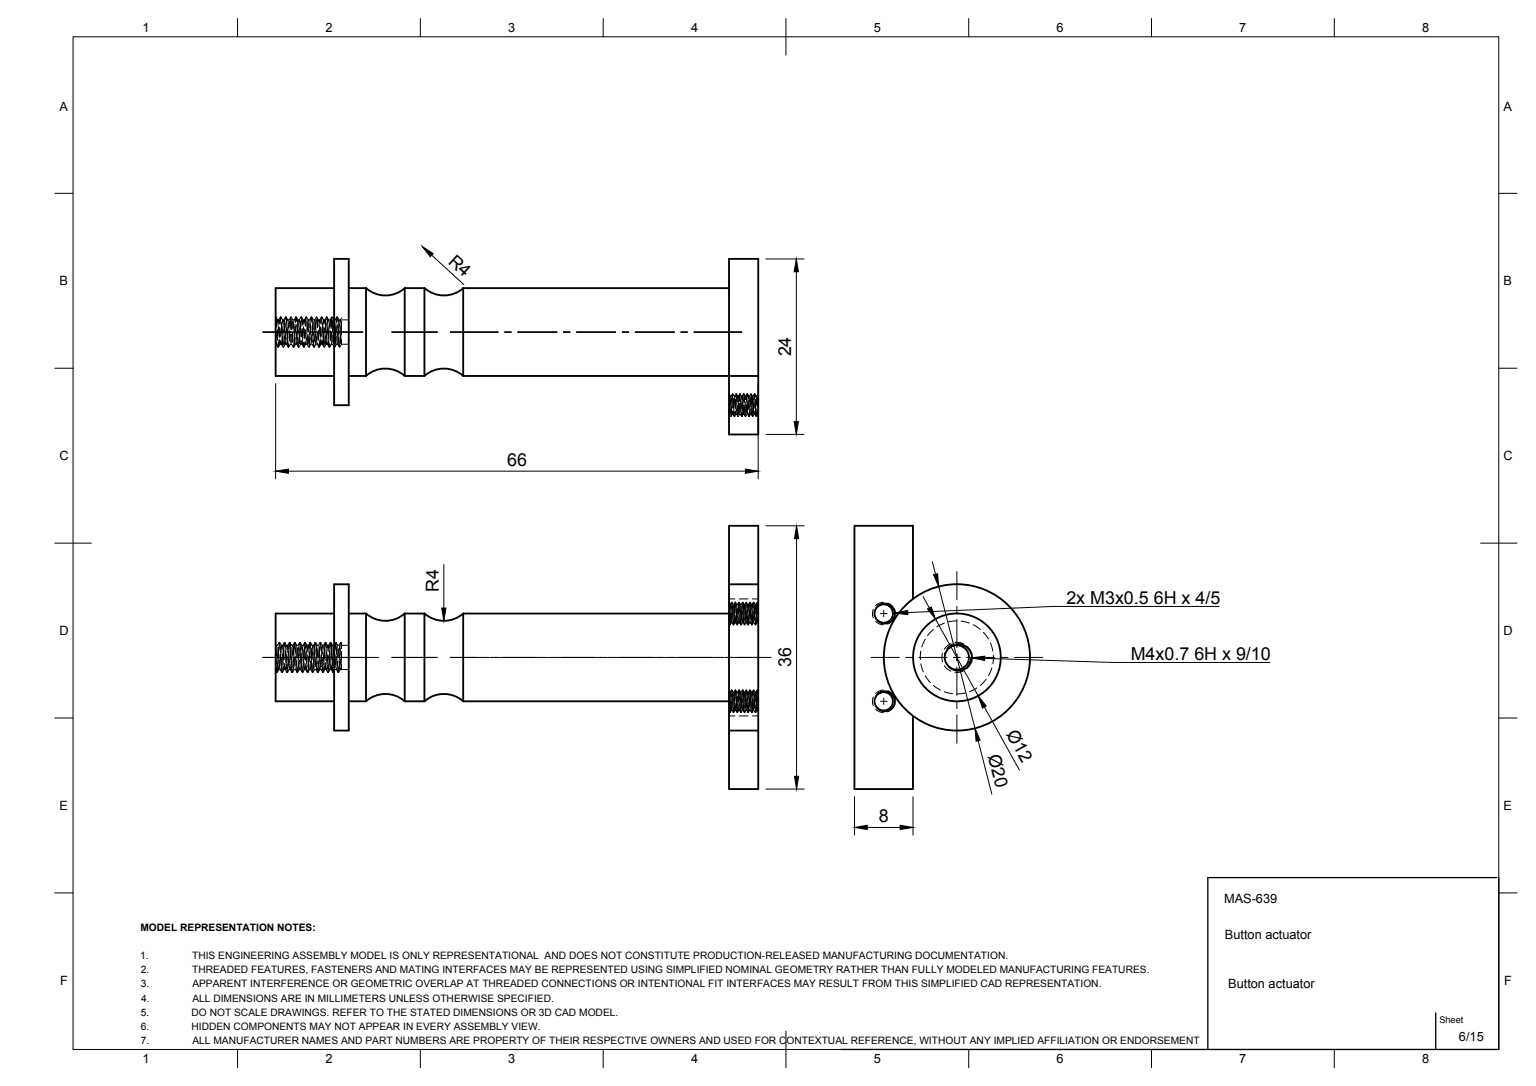
ISO-10303-21;
HEADER;
/* Generated by software containing ST-Developer
 * from STEP Tools, Inc. (www.steptools.com) 
 */

FILE_DESCRIPTION(
/* description */ ('Independent maintained push-to-latch/pull-to-reset mushroom-operator 
CAD. Two opposed spring-loaded ball detents in turned circular seats b
ias both travel stops; direct normally-closed bridge opens6mm when pre
ssed. Rounded palm/pull rim, captured head screw, removable detent clo
sures, native Coil spring families, insulated shared terminals and ord
inary machining features. Manual geometric states and ideal same-mater
ial spring-energy direction only; no electrical/safety certification, 
force/contact dynamics, wear, load or life rating. Requested blue/gray
 visual palette, not safety identification. External wiring/anchors an
d application engineering omitted.'),
/* implementation_level */ '2;1');

FILE_NAME(
/* name */ 'Button actuator.step',
/* time_stamp */ '2026-11-08T17:54:26-08:00',
/* author */ (''),
/* organization */ (''),
/* preprocessor_version */ 'ST-DEVELOPER v20.2',
/* originating_system */ 'Autodesk Translation Framework v15.17.0.0',
/* authorisation */ '');

FILE_SCHEMA (('AUTOMOTIVE_DESIGN { 1 0 10303 214 3 1 1 }'));
ENDSEC;

DATA;
#10=MECHANICAL_DESIGN_GEOMETRIC_PRESENTATION_REPRESENTATION('',(#193),#43980);
#152=TOROIDAL_SURFACE('',#11821,0.899999999999998,0.399999999999998);
#153=TOROIDAL_SURFACE('',#11827,0.900000000000001,0.4);
#159=SHAPE_REPRESENTATION_RELATIONSHIP('SRR','None',#44059,#176);
#176=ADVANCED_BREP_SHAPE_REPRESENTATION('',(#210),#43966);
#193=STYLED_ITEM('',(#44153),#210);
#210=MANIFOLD_SOLID_BREP('Body1',#11234);
#236=B_SPLINE_SURFACE_WITH_KNOTS('',3,3,((#26841,#26842,#26843,#26844,#26845,
#26846,#26847,#26848,#26849,#26850,#26851,#26852,#26853,#26854,#26855,#26856,
#26857,#26858,#26859,#26860,#26861,#26862,#26863,#26864,#26865,#26866,#26867,
#26868,#26869,#26870,#26871,#26872,#26873,#26874,#26875,#26876,#26877,#26878,
#26879,#26880,#26881,#26882,#26883,#26884,#26885,#26886,#26887,#26888,#26889,
#26890,#26891,#26892,#26893,#26894,#26895,#26896),(#26897,#26898,#26899,
#26900,#26901,#26902,#26903,#26904,#26905,#26906,#26907,#26908,#26909,#26910,
#26911,#26912,#26913,#26914,#26915,#26916,#26917,#26918,#26919,#26920,#26921,
#26922,#26923,#26924,#26925,#26926,#26927,#26928,#26929,#26930,#26931,#26932,
#26933,#26934,#26935,#26936,#26937,#26938,#26939,#26940,#26941,#26942,#26943,
#26944,#26945,#26946,#26947,#26948,#26949,#26950,#26951,#26952),(#26953,
#26954,#26955,#26956,#26957,#26958,#26959,#26960,#26961,#26962,#26963,#26964,
#26965,#26966,#26967,#26968,#26969,#26970,#26971,#26972,#26973,#26974,#26975,
#26976,#26977,#26978,#26979,#26980,#26981,#26982,#26983,#26984,#26985,#26986,
#26987,#26988,#26989,#26990,#26991,#26992,#26993,#26994,#26995,#26996,#26997,
#26998,#26999,#27000,#27001,#27002,#27003,#27004,#27005,#27006,#27007,#27008),
(#27009,#27010,#27011,#27012,#27013,#27014,#27015,#27016,#27017,#27018,
#27019,#27020,#27021,#27022,#27023,#27024,#27025,#27026,#27027,#27028,#27029,
#27030,#27031,#27032,#27033,#27034,#27035,#27036,#27037,#27038,#27039,#27040,
#27041,#27042,#27043,#27044,#27045,#27046,#27047,#27048,#27049,#27050,#27051,
#27052,#27053,#27054,#27055,#27056,#27057,#27058,#27059,#27060,#27061,#27062,
#27063,#27064)),.UNSPECIFIED.,.F.,.F.,.F.,(4,4),(4,1,1,1,1,1,1,1,1,1,1,
1,1,1,1,1,1,1,1,1,1,1,1,1,1,1,1,1,1,1,1,1,1,1,1,1,1,1,1,1,1,1,1,1,1,1,1,
1,1,1,1,1,1,4),(0.,0.0321584099938621),(11.8553612635793,12.8418906022433,
13.8284199409074,14.8149492795714,15.8014786182354,16.7880079568995,17.7745372955635,
18.7610666342275,19.7475959728915,20.7341253115556,21.7206546502196,22.7071839888836,
23.6937133275477,24.6802426662117,25.6667720048757,26.6533013435398,27.6398306822038,
28.6263600208678,29.6128893595319,30.5994186981959,31.5859480368599,32.5724773755239,
33.559006714188,34.545536052852,35.532065391516,36.5185947301801,37.5051240688441,
38.4916534075081,39.4781827461722,40.4647120848362,41.4512414235002,42.4377707621643,
43.4243001008283,44.4108294394923,45.3973587781563,46.3838881168204,47.3704174554844,
48.3569467941484,49.3434761328125,50.3300054714765,51.3165348101405,52.3030641488046,
53.2895934874686,54.2761228261326,55.2626521647967,56.2491815034607,57.2357108421247,
58.2222401807888,59.2087695194528,60.1952988581168,61.1818281967808,62.1683575354449,
63.1548868741089,64.1414162127729),.UNSPECIFIED.);
#237=B_SPLINE_SURFACE_WITH_KNOTS('',3,3,((#27191,#27192,#27193,#27194,#27195,
#27196,#27197,#27198,#27199,#27200,#27201,#27202,#27203,#27204,#27205,#27206,
#27207,#27208,#27209,#27210,#27211,#27212,#27213,#27214,#27215,#27216,#27217,
#27218,#27219,#27220,#27221,#27222,#27223,#27224,#27225,#27226,#27227,#27228,
#27229,#27230,#27231,#27232,#27233,#27234,#27235,#27236,#27237,#27238,#27239,
#27240,#27241,#27242,#27243,#27244,#27245,#27246),(#27247,#27248,#27249,
#27250,#27251,#27252,#27253,#27254,#27255,#27256,#27257,#27258,#27259,#27260,
#27261,#27262,#27263,#27264,#27265,#27266,#27267,#27268,#27269,#27270,#27271,
#27272,#27273,#27274,#27275,#27276,#27277,#27278,#27279,#27280,#27281,#27282,
#27283,#27284,#27285,#27286,#27287,#27288,#27289,#27290,#27291,#27292,#27293,
#27294,#27295,#27296,#27297,#27298,#27299,#27300,#27301,#27302),(#27303,
#27304,#27305,#27306,#27307,#27308,#27309,#27310,#27311,#27312,#27313,#27314,
#27315,#27316,#27317,#27318,#27319,#27320,#27321,#27322,#27323,#27324,#27325,
#27326,#27327,#27328,#27329,#27330,#27331,#27332,#27333,#27334,#27335,#27336,
#27337,#27338,#27339,#27340,#27341,#27342,#27343,#27344,#27345,#27346,#27347,
#27348,#27349,#27350,#27351,#27352,#27353,#27354,#27355,#27356,#27357,#27358),
(#27359,#27360,#27361,#27362,#27363,#27364,#27365,#27366,#27367,#27368,
#27369,#27370,#27371,#27372,#27373,#27374,#27375,#27376,#27377,#27378,#27379,
#27380,#27381,#27382,#27383,#27384,#27385,#27386,#27387,#27388,#27389,#27390,
#27391,#27392,#27393,#27394,#27395,#27396,#27397,#27398,#27399,#27400,#27401,
#27402,#27403,#27404,#27405,#27406,#27407,#27408,#27409,#27410,#27411,#27412,
#27413,#27414)),.UNSPECIFIED.,.F.,.F.,.F.,(4,4),(4,1,1,1,1,1,1,1,1,1,1,
1,1,1,1,1,1,1,1,1,1,1,1,1,1,1,1,1,1,1,1,1,1,1,1,1,1,1,1,1,1,1,1,1,1,1,1,
1,1,1,1,1,1,4),(0.,0.0321584099938621),(14.3984001269718,15.3849294656359,
16.3714588042999,17.3579881429639,18.344517481628,19.331046820292,20.317576158956,
21.30410549762,22.2906348362841,23.2771641749481,24.2636935136121,25.2502228522762,
26.2367521909402,27.2232815296042,28.2098108682683,29.1963402069323,30.1828695455963,
31.1693988842604,32.1559282229244,33.1424575615884,34.1289869002524,35.1155162389165,
36.1020455775805,37.0885749162445,38.0751042549086,39.0616335935726,40.0481629322366,
41.0346922709007,42.0212216095647,43.0077509482287,43.9942802868928,44.9808096255568,
45.9673389642208,46.9538683028848,47.9403976415489,48.9269269802129,49.9134563188769,
50.899985657541,51.886514996205,52.873044334869,53.8595736735331,54.8461030121971,
55.8326323508611,56.8191616895251,57.8056910281892,58.7922203668532,59.7787497055172,
60.7652790441813,61.7518083828453,62.7383377215093,63.7248670601734,64.7113963988374,
65.6979257375014,66.6844550761655),.UNSPECIFIED.);
#238=B_SPLINE_SURFACE_WITH_KNOTS('',3,3,((#27677,#27678,#27679,#27680,#27681,
#27682,#27683,#27684,#27685,#27686,#27687,#27688,#27689,#27690,#27691,#27692,
#27693,#27694,#27695,#27696,#27697,#27698,#27699,#27700,#27701,#27702,#27703,
#27704,#27705,#27706,#27707,#27708,#27709,#27710,#27711,#27712,#27713,#27714,
#27715,#27716,#27717,#27718,#27719,#27720,#27721,#27722,#27723,#27724,#27725,
#27726,#27727,#27728,#27729,#27730,#27731,#27732),(#27733,#27734,#27735,
#27736,#27737,#27738,#27739,#27740,#27741,#27742,#27743,#27744,#27745,#27746,
#27747,#27748,#27749,#27750,#27751,#27752,#27753,#27754,#27755,#27756,#27757,
#27758,#27759,#27760,#27761,#27762,#27763,#27764,#27765,#27766,#27767,#27768,
#27769,#27770,#27771,#27772,#27773,#27774,#27775,#27776,#27777,#27778,#27779,
#27780,#27781,#27782,#27783,#27784,#27785,#27786,#27787,#27788),(#27789,
#27790,#27791,#27792,#27793,#27794,#27795,#27796,#27797,#27798,#27799,#27800,
#27801,#27802,#27803,#27804,#27805,#27806,#27807,#27808,#27809,#27810,#27811,
#27812,#27813,#27814,#27815,#27816,#27817,#27818,#27819,#27820,#27821,#27822,
#27823,#27824,#27825,#27826,#27827,#27828,#27829,#27830,#27831,#27832,#27833,
#27834,#27835,#27836,#27837,#27838,#27839,#27840,#27841,#27842,#27843,#27844),
(#27845,#27846,#27847,#27848,#27849,#27850,#27851,#27852,#27853,#27854,
#27855,#27856,#27857,#27858,#27859,#27860,#27861,#27862,#27863,#27864,#27865,
#27866,#27867,#27868,#27869,#27870,#27871,#27872,#27873,#27874,#27875,#27876,
#27877,#27878,#27879,#27880,#27881,#27882,#27883,#27884,#27885,#27886,#27887,
#27888,#27889,#27890,#27891,#27892,#27893,#27894,#27895,#27896,#27897,#27898,
#27899,#27900)),.UNSPECIFIED.,.F.,.F.,.F.,(4,4),(4,1,1,1,1,1,1,1,1,1,1,
1,1,1,1,1,1,1,1,1,1,1,1,1,1,1,1,1,1,1,1,1,1,1,1,1,1,1,1,1,1,1,1,1,1,1,1,
1,1,1,1,1,1,4),(0.,0.0321584099938621),(11.8553612635793,12.8418906022433,
13.8284199409074,14.8149492795714,15.8014786182354,16.7880079568995,17.7745372955635,
18.7610666342275,19.7475959728915,20.7341253115556,21.7206546502196,22.7071839888836,
23.6937133275477,24.6802426662117,25.6667720048757,26.6533013435398,27.6398306822038,
28.6263600208678,29.6128893595319,30.5994186981959,31.5859480368599,32.5724773755239,
33.559006714188,34.545536052852,35.532065391516,36.5185947301801,37.5051240688441,
38.4916534075081,39.4781827461722,40.4647120848362,41.4512414235002,42.4377707621643,
43.4243001008283,44.4108294394923,45.3973587781563,46.3838881168204,47.3704174554844,
48.3569467941484,49.3434761328125,50.3300054714765,51.3165348101405,52.3030641488046,
53.2895934874686,54.2761228261326,55.2626521647967,56.2491815034607,57.2357108421247,
58.2222401807888,59.2087695194528,60.1952988581168,61.1818281967808,62.1683575354449,
63.1548868741089,64.1414162127729),.UNSPECIFIED.);
#239=B_SPLINE_SURFACE_WITH_KNOTS('',3,3,((#27975,#27976,#27977,#27978,#27979,
#27980,#27981,#27982,#27983,#27984,#27985,#27986,#27987,#27988,#27989,#27990,
#27991,#27992,#27993,#27994,#27995,#27996,#27997,#27998,#27999,#28000,#28001,
#28002,#28003,#28004,#28005,#28006,#28007,#28008,#28009,#28010,#28011,#28012,
#28013,#28014,#28015,#28016,#28017,#28018,#28019,#28020,#28021,#28022,#28023,
#28024,#28025,#28026,#28027,#28028,#28029,#28030),(#28031,#28032,#28033,
#28034,#28035,#28036,#28037,#28038,#28039,#28040,#28041,#28042,#28043,#28044,
#28045,#28046,#28047,#28048,#28049,#28050,#28051,#28052,#28053,#28054,#28055,
#28056,#28057,#28058,#28059,#28060,#28061,#28062,#28063,#28064,#28065,#28066,
#28067,#28068,#28069,#28070,#28071,#28072,#28073,#28074,#28075,#28076,#28077,
#28078,#28079,#28080,#28081,#28082,#28083,#28084,#28085,#28086),(#28087,
#28088,#28089,#28090,#28091,#28092,#28093,#28094,#28095,#28096,#28097,#28098,
#28099,#28100,#28101,#28102,#28103,#28104,#28105,#28106,#28107,#28108,#28109,
#28110,#28111,#28112,#28113,#28114,#28115,#28116,#28117,#28118,#28119,#28120,
#28121,#28122,#28123,#28124,#28125,#28126,#28127,#28128,#28129,#28130,#28131,
#28132,#28133,#28134,#28135,#28136,#28137,#28138,#28139,#28140,#28141,#28142),
(#28143,#28144,#28145,#28146,#28147,#28148,#28149,#28150,#28151,#28152,
#28153,#28154,#28155,#28156,#28157,#28158,#28159,#28160,#28161,#28162,#28163,
#28164,#28165,#28166,#28167,#28168,#28169,#28170,#28171,#28172,#28173,#28174,
#28175,#28176,#28177,#28178,#28179,#28180,#28181,#28182,#28183,#28184,#28185,
#28186,#28187,#28188,#28189,#28190,#28191,#28192,#28193,#28194,#28195,#28196,
#28197,#28198)),.UNSPECIFIED.,.F.,.F.,.F.,(4,4),(4,1,1,1,1,1,1,1,1,1,1,
1,1,1,1,1,1,1,1,1,1,1,1,1,1,1,1,1,1,1,1,1,1,1,1,1,1,1,1,1,1,1,1,1,1,1,1,
1,1,1,1,1,1,4),(0.,0.0321584099938621),(14.3984001269718,15.3849294656359,
16.3714588042999,17.3579881429639,18.344517481628,19.331046820292,20.317576158956,
21.30410549762,22.2906348362841,23.2771641749481,24.2636935136121,25.2502228522762,
26.2367521909402,27.2232815296042,28.2098108682683,29.1963402069323,30.1828695455963,
31.1693988842604,32.1559282229244,33.1424575615884,34.1289869002524,35.1155162389165,
36.1020455775805,37.0885749162445,38.0751042549086,39.0616335935726,40.0481629322366,
41.0346922709007,42.0212216095647,43.0077509482287,43.9942802868928,44.9808096255568,
45.9673389642208,46.9538683028848,47.9403976415489,48.9269269802129,49.9134563188769,
50.899985657541,51.886514996205,52.873044334869,53.8595736735331,54.8461030121971,
55.8326323508611,56.8191616895251,57.8056910281892,58.7922203668532,59.7787497055172,
60.7652790441813,61.7518083828453,62.7383377215093,63.7248670601734,64.7113963988374,
65.6979257375014,66.6844550761655),.UNSPECIFIED.);
#240=B_SPLINE_SURFACE_WITH_KNOTS('',3,3,((#28411,#28412,#28413,#28414,#28415,
#28416,#28417,#28418,#28419,#28420,#28421,#28422,#28423,#28424,#28425,#28426,
#28427,#28428,#28429,#28430,#28431,#28432,#28433,#28434,#28435,#28436,#28437,
#28438,#28439,#28440,#28441,#28442,#28443,#28444,#28445,#28446,#28447,#28448,
#28449,#28450,#28451,#28452,#28453,#28454,#28455,#28456,#28457,#28458,#28459,
#28460,#28461,#28462,#28463,#28464,#28465,#28466,#28467,#28468,#28469,#28470,
#28471,#28472,#28473,#28474,#28475,#28476,#28477,#28478,#28479,#28480,#28481,
#28482,#28483,#28484,#28485,#28486,#28487,#28488,#28489,#28490,#28491,#28492,
#28493,#28494,#28495,#28496),(#28497,#28498,#28499,#28500,#28501,#28502,
#28503,#28504,#28505,#28506,#28507,#28508,#28509,#28510,#28511,#28512,#28513,
#28514,#28515,#28516,#28517,#28518,#28519,#28520,#28521,#28522,#28523,#28524,
#28525,#28526,#28527,#28528,#28529,#28530,#28531,#28532,#28533,#28534,#28535,
#28536,#28537,#28538,#28539,#28540,#28541,#28542,#28543,#28544,#28545,#28546,
#28547,#28548,#28549,#28550,#28551,#28552,#28553,#28554,#28555,#28556,#28557,
#28558,#28559,#28560,#28561,#28562,#28563,#28564,#28565,#28566,#28567,#28568,
#28569,#28570,#28571,#28572,#28573,#28574,#28575,#28576,#28577,#28578,#28579,
#28580,#28581,#28582),(#28583,#28584,#28585,#28586,#28587,#28588,#28589,
#28590,#28591,#28592,#28593,#28594,#28595,#28596,#28597,#28598,#28599,#28600,
#28601,#28602,#28603,#28604,#28605,#28606,#28607,#28608,#28609,#28610,#28611,
#28612,#28613,#28614,#28615,#28616,#28617,#28618,#28619,#28620,#28621,#28622,
#28623,#28624,#28625,#28626,#28627,#28628,#28629,#28630,#28631,#28632,#28633,
#28634,#28635,#28636,#28637,#28638,#28639,#28640,#28641,#28642,#28643,#28644,
#28645,#28646,#28647,#28648,#28649,#28650,#28651,#28652,#28653,#28654,#28655,
#28656,#28657,#28658,#28659,#28660,#28661,#28662,#28663,#28664,#28665,#28666,
#28667,#28668),(#28669,#28670,#28671,#28672,#28673,#28674,#28675,#28676,
#28677,#28678,#28679,#28680,#28681,#28682,#28683,#28684,#28685,#28686,#28687,
#28688,#28689,#28690,#28691,#28692,#28693,#28694,#28695,#28696,#28697,#28698,
#28699,#28700,#28701,#28702,#28703,#28704,#28705,#28706,#28707,#28708,#28709,
#28710,#28711,#28712,#28713,#28714,#28715,#28716,#28717,#28718,#28719,#28720,
#28721,#28722,#28723,#28724,#28725,#28726,#28727,#28728,#28729,#28730,#28731,
#28732,#28733,#28734,#28735,#28736,#28737,#28738,#28739,#28740,#28741,#28742,
#28743,#28744,#28745,#28746,#28747,#28748,#28749,#28750,#28751,#28752,#28753,
#28754)),.UNSPECIFIED.,.F.,.F.,.F.,(4,4),(4,1,1,1,1,1,1,1,1,1,1,1,1,1,1,
1,1,1,1,1,1,1,1,1,1,1,1,1,1,1,1,1,1,1,1,1,1,1,1,1,1,1,1,1,1,1,1,1,1,1,1,
1,1,1,1,1,1,1,1,1,1,1,1,1,1,1,1,1,1,1,1,1,1,1,1,1,1,1,1,1,1,1,1,4),(0.,
0.0448889834294937),(11.8615800042566,12.8591513772395,13.8567227502225,
14.8542941232054,15.8518654961883,16.8494368691713,17.8470082421542,18.8445796151371,
19.8421509881201,20.839722361103,21.837293734086,22.8348651070689,23.8324364800518,
24.8300078530348,25.8275792260177,26.8251505990006,27.8227219719836,28.8202933449665,
29.8178647179494,30.8154360909324,31.8130074639153,32.8105788368982,33.8081502098812,
34.8057215828641,35.803292955847,36.80086432883,37.7984357018129,38.7960070747958,
39.7935784477788,40.7911498207617,41.7887211937446,42.7862925667276,43.7838639397105,
44.7814353126934,45.7790066856764,46.7765780586593,47.7741494316422,48.7717208046252,
49.7692921776081,50.766863550591,51.764434923574,52.7620062965569,53.7595776695398,
54.7571490425228,55.7547204155057,56.7522917884886,57.7498631614716,58.7474345344545,
59.7450059074374,60.7425772804204,61.7401486534033,62.7377200263862,63.7352913993692,
64.7328627723521,65.730434145335,66.728005518318,67.7255768913009,68.7231482642838,
69.7207196372668,70.7182910102497,71.7158623832326,72.7134337562156,73.7110051291985,
74.7085765021814,75.7061478751644,76.7037192481473,77.7012906211302,78.6988619941132,
79.6964333670961,80.6940047400791,81.691576113062,82.6891474860449,83.6867188590278,
84.6842902320108,85.6818616049937,86.6794329779766,87.6770043509596,88.6745757239425,
89.6721470969255,90.6697184699084,91.6672898428913,92.6648612158743,93.6624325888572,
94.6600039618401),.UNSPECIFIED.);
#241=B_SPLINE_SURFACE_WITH_KNOTS('',3,3,((#28832,#28833,#28834,#28835,#28836,
#28837,#28838,#28839,#28840,#28841,#28842,#28843,#28844,#28845,#28846,#28847,
#28848,#28849,#28850,#28851,#28852,#28853,#28854,#28855,#28856,#28857,#28858,
#28859,#28860,#28861,#28862,#28863,#28864,#28865,#28866,#28867,#28868,#28869,
#28870,#28871,#28872,#28873,#28874,#28875,#28876,#28877,#28878,#28879,#28880,
#28881,#28882,#28883,#28884,#28885,#28886,#28887,#28888,#28889,#28890,#28891,
#28892,#28893,#28894,#28895,#28896,#28897,#28898,#28899,#28900,#28901,#28902,
#28903,#28904,#28905,#28906,#28907,#28908,#28909,#28910,#28911,#28912,#28913,
#28914,#28915,#28916,#28917),(#28918,#28919,#28920,#28921,#28922,#28923,
#28924,#28925,#28926,#28927,#28928,#28929,#28930,#28931,#28932,#28933,#28934,
#28935,#28936,#28937,#28938,#28939,#28940,#28941,#28942,#28943,#28944,#28945,
#28946,#28947,#28948,#28949,#28950,#28951,#28952,#28953,#28954,#28955,#28956,
#28957,#28958,#28959,#28960,#28961,#28962,#28963,#28964,#28965,#28966,#28967,
#28968,#28969,#28970,#28971,#28972,#28973,#28974,#28975,#28976,#28977,#28978,
#28979,#28980,#28981,#28982,#28983,#28984,#28985,#28986,#28987,#28988,#28989,
#28990,#28991,#28992,#28993,#28994,#28995,#28996,#28997,#28998,#28999,#29000,
#29001,#29002,#29003),(#29004,#29005,#29006,#29007,#29008,#29009,#29010,
#29011,#29012,#29013,#29014,#29015,#29016,#29017,#29018,#29019,#29020,#29021,
#29022,#29023,#29024,#29025,#29026,#29027,#29028,#29029,#29030,#29031,#29032,
#29033,#29034,#29035,#29036,#29037,#29038,#29039,#29040,#29041,#29042,#29043,
#29044,#29045,#29046,#29047,#29048,#29049,#29050,#29051,#29052,#29053,#29054,
#29055,#29056,#29057,#29058,#29059,#29060,#29061,#29062,#29063,#29064,#29065,
#29066,#29067,#29068,#29069,#29070,#29071,#29072,#29073,#29074,#29075,#29076,
#29077,#29078,#29079,#29080,#29081,#29082,#29083,#29084,#29085,#29086,#29087,
#29088,#29089),(#29090,#29091,#29092,#29093,#29094,#29095,#29096,#29097,
#29098,#29099,#29100,#29101,#29102,#29103,#29104,#29105,#29106,#29107,#29108,
#29109,#29110,#29111,#29112,#29113,#29114,#29115,#29116,#29117,#29118,#29119,
#29120,#29121,#29122,#29123,#29124,#29125,#29126,#29127,#29128,#29129,#29130,
#29131,#29132,#29133,#29134,#29135,#29136,#29137,#29138,#29139,#29140,#29141,
#29142,#29143,#29144,#29145,#29146,#29147,#29148,#29149,#29150,#29151,#29152,
#29153,#29154,#29155,#29156,#29157,#29158,#29159,#29160,#29161,#29162,#29163,
#29164,#29165,#29166,#29167,#29168,#29169,#29170,#29171,#29172,#29173,#29174,
#29175)),.UNSPECIFIED.,.F.,.F.,.F.,(4,4),(4,1,1,1,1,1,1,1,1,1,1,1,1,1,1,
1,1,1,1,1,1,1,1,1,1,1,1,1,1,1,1,1,1,1,1,1,1,1,1,1,1,1,1,1,1,1,1,1,1,1,1,
1,1,1,1,1,1,1,1,1,1,1,1,1,1,1,1,1,1,1,1,1,1,1,1,1,1,1,1,1,1,1,1,4),(0.,
0.0448889834294937),(14.3981410127768,15.3957123857598,16.3932837587427,
17.3908551317256,18.3884265047086,19.3859978776915,20.3835692506744,21.3811406236574,
22.3787119966403,23.3762833696232,24.3738547426062,25.3714261155891,26.368997488572,
27.366568861555,28.3641402345379,29.3617116075208,30.3592829805038,31.3568543534867,
32.3544257264696,33.3519970994526,34.3495684724355,35.3471398454184,36.3447112184014,
37.3422825913843,38.3398539643672,39.3374253373502,40.3349967103331,41.332568083316,
42.330139456299,43.3277108292819,44.3252822022648,45.3228535752478,46.3204249482307,
47.3179963212136,48.3155676941966,49.3131390671795,50.3107104401624,51.3082818131454,
52.3058531861283,53.3034245591112,54.3009959320942,55.2985673050771,56.29613867806,
57.293710051043,58.2912814240259,59.2888527970089,60.2864241699918,61.2839955429747,
62.2815669159576,63.2791382889406,64.2767096619235,65.2742810349065,66.2718524078894,
67.2694237808723,68.2669951538552,69.2645665268382,70.2621378998211,71.2597092728041,
72.257280645787,73.2548520187699,74.2524233917528,75.2499947647358,76.2475661377187,
77.2451375107017,78.2427088836846,79.2402802566675,80.2378516296505,81.2354230026334,
82.2329943756163,83.2305657485992,84.2281371215822,85.2257084945651,86.2232798675481,
87.220851240531,88.2184226135139,89.2159939864968,90.2135653594798,91.2111367324627,
92.2087081054457,93.2062794784286,94.2038508514115,95.2014222243945,96.1989935973774,
97.1965649703603),.UNSPECIFIED.);
#298=FACE_BOUND('',#1431,.T.);
#299=FACE_BOUND('',#1432,.T.);
#300=FACE_BOUND('',#1449,.T.);
#301=FACE_BOUND('',#1451,.T.);
#302=FACE_BOUND('',#1462,.T.);
#303=FACE_BOUND('',#1464,.T.);
#304=FACE_BOUND('',#1465,.T.);
#305=FACE_BOUND('',#1466,.T.);
#388=PLANE('',#11812);
#389=PLANE('',#11817);
#390=PLANE('',#11820);
#391=PLANE('',#11832);
#392=PLANE('',#11835);
#393=PLANE('',#11840);
#394=PLANE('',#11841);
#395=PLANE('',#11842);
#396=PLANE('',#11843);
#397=PLANE('',#11844);
#398=PLANE('',#11849);
#399=PLANE('',#11850);
#708=FACE_OUTER_BOUND('',#1370,.T.);
#709=FACE_OUTER_BOUND('',#1371,.T.);
#710=FACE_OUTER_BOUND('',#1372,.T.);
#711=FACE_OUTER_BOUND('',#1373,.T.);
#712=FACE_OUTER_BOUND('',#1374,.T.);
#713=FACE_OUTER_BOUND('',#1375,.T.);
#714=FACE_OUTER_BOUND('',#1376,.T.);
#715=FACE_OUTER_BOUND('',#1377,.T.);
#716=FACE_OUTER_BOUND('',#1378,.T.);
#717=FACE_OUTER_BOUND('',#1379,.T.);
#718=FACE_OUTER_BOUND('',#1380,.T.);
#719=FACE_OUTER_BOUND('',#1381,.T.);
#720=FACE_OUTER_BOUND('',#1382,.T.);
#721=FACE_OUTER_BOUND('',#1383,.T.);
#722=FACE_OUTER_BOUND('',#1384,.T.);
#723=FACE_OUTER_BOUND('',#1385,.T.);
#724=FACE_OUTER_BOUND('',#1386,.T.);
#725=FACE_OUTER_BOUND('',#1387,.T.);
#726=FACE_OUTER_BOUND('',#1388,.T.);
#727=FACE_OUTER_BOUND('',#1389,.T.);
#728=FACE_OUTER_BOUND('',#1390,.T.);
#729=FACE_OUTER_BOUND('',#1391,.T.);
#730=FACE_OUTER_BOUND('',#1392,.T.);
#731=FACE_OUTER_BOUND('',#1393,.T.);
#732=FACE_OUTER_BOUND('',#1394,.T.);
#733=FACE_OUTER_BOUND('',#1395,.T.);
#734=FACE_OUTER_BOUND('',#1396,.T.);
#735=FACE_OUTER_BOUND('',#1397,.T.);
#736=FACE_OUTER_BOUND('',#1398,.T.);
#737=FACE_OUTER_BOUND('',#1399,.T.);
#738=FACE_OUTER_BOUND('',#1400,.T.);
#739=FACE_OUTER_BOUND('',#1401,.T.);
#740=FACE_OUTER_BOUND('',#1402,.T.);
#741=FACE_OUTER_BOUND('',#1403,.T.);
#742=FACE_OUTER_BOUND('',#1404,.T.);
#743=FACE_OUTER_BOUND('',#1405,.T.);
#744=FACE_OUTER_BOUND('',#1406,.T.);
#745=FACE_OUTER_BOUND('',#1407,.T.);
#746=FACE_OUTER_BOUND('',#1408,.T.);
#747=FACE_OUTER_BOUND('',#1409,.T.);
#748=FACE_OUTER_BOUND('',#1410,.T.);
#749=FACE_OUTER_BOUND('',#1411,.T.);
#750=FACE_OUTER_BOUND('',#1412,.T.);
#751=FACE_OUTER_BOUND('',#1413,.T.);
#752=FACE_OUTER_BOUND('',#1414,.T.);
#753=FACE_OUTER_BOUND('',#1415,.T.);
#754=FACE_OUTER_BOUND('',#1416,.T.);
#755=FACE_OUTER_BOUND('',#1417,.T.);
#756=FACE_OUTER_BOUND('',#1418,.T.);
#757=FACE_OUTER_BOUND('',#1419,.T.);
#758=FACE_OUTER_BOUND('',#1420,.T.);
#759=FACE_OUTER_BOUND('',#1421,.T.);
#760=FACE_OUTER_BOUND('',#1422,.T.);
#761=FACE_OUTER_BOUND('',#1423,.T.);
#762=FACE_OUTER_BOUND('',#1424,.T.);
#763=FACE_OUTER_BOUND('',#1425,.T.);
#764=FACE_OUTER_BOUND('',#1426,.T.);
#765=FACE_OUTER_BOUND('',#1427,.T.);
#766=FACE_OUTER_BOUND('',#1428,.T.);
#767=FACE_OUTER_BOUND('',#1429,.T.);
#768=FACE_OUTER_BOUND('',#1430,.T.);
#769=FACE_OUTER_BOUND('',#1433,.T.);
#770=FACE_OUTER_BOUND('',#1434,.T.);
#771=FACE_OUTER_BOUND('',#1435,.T.);
#772=FACE_OUTER_BOUND('',#1436,.T.);
#773=FACE_OUTER_BOUND('',#1437,.T.);
#774=FACE_OUTER_BOUND('',#1438,.T.);
#775=FACE_OUTER_BOUND('',#1439,.T.);
#776=FACE_OUTER_BOUND('',#1440,.T.);
#777=FACE_OUTER_BOUND('',#1441,.T.);
#778=FACE_OUTER_BOUND('',#1442,.T.);
#779=FACE_OUTER_BOUND('',#1443,.T.);
#780=FACE_OUTER_BOUND('',#1444,.T.);
#781=FACE_OUTER_BOUND('',#1445,.T.);
#782=FACE_OUTER_BOUND('',#1446,.T.);
#783=FACE_OUTER_BOUND('',#1447,.T.);
#784=FACE_OUTER_BOUND('',#1448,.T.);
#785=FACE_OUTER_BOUND('',#1450,.T.);
#786=FACE_OUTER_BOUND('',#1452,.T.);
#787=FACE_OUTER_BOUND('',#1453,.T.);
#788=FACE_OUTER_BOUND('',#1454,.T.);
#789=FACE_OUTER_BOUND('',#1455,.T.);
#790=FACE_OUTER_BOUND('',#1456,.T.);
#791=FACE_OUTER_BOUND('',#1457,.T.);
#792=FACE_OUTER_BOUND('',#1458,.T.);
#793=FACE_OUTER_BOUND('',#1459,.T.);
#794=FACE_OUTER_BOUND('',#1460,.T.);
#795=FACE_OUTER_BOUND('',#1461,.T.);
#796=FACE_OUTER_BOUND('',#1463,.T.);
#1370=EDGE_LOOP('',(#8081,#8082,#8083,#8084,#8085,#8086,#8087,#8088));
#1371=EDGE_LOOP('',(#8089,#8090,#8091,#8092));
#1372=EDGE_LOOP('',(#8093,#8094,#8095,#8096));
#1373=EDGE_LOOP('',(#8097,#8098,#8099,#8100));
#1374=EDGE_LOOP('',(#8101,#8102,#8103,#8104));
#1375=EDGE_LOOP('',(#8105,#8106,#8107,#8108));
#1376=EDGE_LOOP('',(#8109,#8110,#8111,#8112));
#1377=EDGE_LOOP('',(#8113,#8114,#8115,#8116));
#1378=EDGE_LOOP('',(#8117,#8118,#8119,#8120));
#1379=EDGE_LOOP('',(#8121,#8122,#8123,#8124));
#1380=EDGE_LOOP('',(#8125,#8126,#8127,#8128));
#1381=EDGE_LOOP('',(#8129,#8130,#8131,#8132));
#1382=EDGE_LOOP('',(#8133,#8134,#8135,#8136));
#1383=EDGE_LOOP('',(#8137,#8138,#8139,#8140));
#1384=EDGE_LOOP('',(#8141,#8142,#8143,#8144));
#1385=EDGE_LOOP('',(#8145,#8146,#8147,#8148));
#1386=EDGE_LOOP('',(#8149,#8150,#8151,#8152));
#1387=EDGE_LOOP('',(#8153,#8154,#8155,#8156));
#1388=EDGE_LOOP('',(#8157,#8158,#8159,#8160));
#1389=EDGE_LOOP('',(#8161,#8162,#8163,#8164));
#1390=EDGE_LOOP('',(#8165,#8166,#8167,#8168));
#1391=EDGE_LOOP('',(#8169,#8170,#8171,#8172));
#1392=EDGE_LOOP('',(#8173,#8174,#8175,#8176));
#1393=EDGE_LOOP('',(#8177,#8178,#8179,#8180));
#1394=EDGE_LOOP('',(#8181,#8182,#8183,#8184));
#1395=EDGE_LOOP('',(#8185,#8186,#8187,#8188));
#1396=EDGE_LOOP('',(#8189,#8190,#8191,#8192));
#1397=EDGE_LOOP('',(#8193,#8194,#8195,#8196));
#1398=EDGE_LOOP('',(#8197,#8198,#8199,#8200));
#1399=EDGE_LOOP('',(#8201,#8202,#8203,#8204));
#1400=EDGE_LOOP('',(#8205,#8206,#8207,#8208));
#1401=EDGE_LOOP('',(#8209,#8210,#8211,#8212));
#1402=EDGE_LOOP('',(#8213,#8214,#8215,#8216));
#1403=EDGE_LOOP('',(#8217,#8218,#8219,#8220));
#1404=EDGE_LOOP('',(#8221,#8222,#8223,#8224));
#1405=EDGE_LOOP('',(#8225,#8226,#8227,#8228));
#1406=EDGE_LOOP('',(#8229,#8230,#8231,#8232));
#1407=EDGE_LOOP('',(#8233,#8234,#8235,#8236));
#1408=EDGE_LOOP('',(#8237,#8238,#8239,#8240));
#1409=EDGE_LOOP('',(#8241,#8242,#8243,#8244));
#1410=EDGE_LOOP('',(#8245,#8246,#8247,#8248));
#1411=EDGE_LOOP('',(#8249,#8250,#8251,#8252));
#1412=EDGE_LOOP('',(#8253,#8254,#8255,#8256));
#1413=EDGE_LOOP('',(#8257,#8258,#8259,#8260));
#1414=EDGE_LOOP('',(#8261,#8262,#8263,#8264));
#1415=EDGE_LOOP('',(#8265,#8266,#8267,#8268));
#1416=EDGE_LOOP('',(#8269,#8270,#8271,#8272));
#1417=EDGE_LOOP('',(#8273,#8274,#8275,#8276));
#1418=EDGE_LOOP('',(#8277,#8278,#8279,#8280));
#1419=EDGE_LOOP('',(#8281,#8282,#8283,#8284));
#1420=EDGE_LOOP('',(#8285,#8286,#8287,#8288));
#1421=EDGE_LOOP('',(#8289,#8290,#8291,#8292));
#1422=EDGE_LOOP('',(#8293,#8294,#8295,#8296));
#1423=EDGE_LOOP('',(#8297,#8298,#8299,#8300));
#1424=EDGE_LOOP('',(#8301,#8302,#8303,#8304));
#1425=EDGE_LOOP('',(#8305,#8306,#8307,#8308));
#1426=EDGE_LOOP('',(#8309,#8310,#8311,#8312));
#1427=EDGE_LOOP('',(#8313,#8314,#8315,#8316));
#1428=EDGE_LOOP('',(#8317,#8318,#8319,#8320,#8321,#8322,#8323,#8324,#8325,
#8326,#8327,#8328,#8329,#8330,#8331,#8332,#8333,#8334,#8335,#8336));
#1429=EDGE_LOOP('',(#8337,#8338,#8339,#8340,#8341,#8342,#8343,#8344,#8345,
#8346,#8347,#8348,#8349,#8350,#8351,#8352,#8353,#8354,#8355,#8356));
#1430=EDGE_LOOP('',(#8357,#8358,#8359,#8360,#8361,#8362));
#1431=EDGE_LOOP('',(#8363,#8364,#8365,#8366));
#1432=EDGE_LOOP('',(#8367,#8368,#8369,#8370));
#1433=EDGE_LOOP('',(#8371,#8372,#8373,#8374));
#1434=EDGE_LOOP('',(#8375,#8376,#8377,#8378,#8379,#8380,#8381,#8382,#8383,
#8384,#8385,#8386,#8387,#8388,#8389,#8390,#8391,#8392,#8393,#8394));
#1435=EDGE_LOOP('',(#8395,#8396,#8397,#8398,#8399,#8400,#8401,#8402,#8403,
#8404,#8405,#8406,#8407,#8408,#8409,#8410,#8411,#8412,#8413,#8414));
#1436=EDGE_LOOP('',(#8415,#8416,#8417,#8418));
#1437=EDGE_LOOP('',(#8419,#8420,#8421,#8422));
#1438=EDGE_LOOP('',(#8423,#8424,#8425,#8426));
#1439=EDGE_LOOP('',(#8427,#8428,#8429,#8430));
#1440=EDGE_LOOP('',(#8431,#8432,#8433,#8434,#8435,#8436,#8437,#8438,#8439,
#8440,#8441,#8442,#8443,#8444,#8445,#8446,#8447,#8448,#8449,#8450,#8451,
#8452,#8453,#8454,#8455,#8456,#8457,#8458,#8459,#8460));
#1441=EDGE_LOOP('',(#8461,#8462,#8463,#8464,#8465,#8466,#8467,#8468,#8469,
#8470,#8471,#8472,#8473,#8474,#8475,#8476,#8477,#8478,#8479,#8480,#8481,
#8482,#8483,#8484,#8485,#8486,#8487,#8488,#8489));
#1442=EDGE_LOOP('',(#8490,#8491,#8492,#8493));
#1443=EDGE_LOOP('',(#8494));
#1444=EDGE_LOOP('',(#8495,#8496,#8497,#8498));
#1445=EDGE_LOOP('',(#8499,#8500,#8501,#8502));
#1446=EDGE_LOOP('',(#8503,#8504,#8505,#8506));
#1447=EDGE_LOOP('',(#8507,#8508,#8509,#8510));
#1448=EDGE_LOOP('',(#8511));
#1449=EDGE_LOOP('',(#8512));
#1450=EDGE_LOOP('',(#8513));
#1451=EDGE_LOOP('',(#8514));
#1452=EDGE_LOOP('',(#8515,#8516,#8517,#8518));
#1453=EDGE_LOOP('',(#8519,#8520,#8521,#8522));
#1454=EDGE_LOOP('',(#8523,#8524,#8525,#8526));
#1455=EDGE_LOOP('',(#8527,#8528,#8529,#8530));
#1456=EDGE_LOOP('',(#8531,#8532,#8533,#8534));
#1457=EDGE_LOOP('',(#8535,#8536,#8537,#8538));
#1458=EDGE_LOOP('',(#8539,#8540,#8541,#8542));
#1459=EDGE_LOOP('',(#8543,#8544,#8545,#8546));
#1460=EDGE_LOOP('',(#8547,#8548,#8549,#8550));
#1461=EDGE_LOOP('',(#8551));
#1462=EDGE_LOOP('',(#8552,#8553,#8554,#8555));
#1463=EDGE_LOOP('',(#8556,#8557,#8558,#8559,#8560,#8561));
#1464=EDGE_LOOP('',(#8562,#8563,#8564,#8565));
#1465=EDGE_LOOP('',(#8566,#8567,#8568,#8569));
#1466=EDGE_LOOP('',(#8570));
#1889=CIRCLE('',#11742,0.1666);
#1890=CIRCLE('',#11743,0.1666);
#1891=CIRCLE('',#11755,0.1666);
#1892=CIRCLE('',#11757,0.205475);
#1893=CIRCLE('',#11770,0.205475);
#1894=CIRCLE('',#11772,0.12645);
#1895=CIRCLE('',#11780,0.12645);
#1896=CIRCLE('',#11782,0.12645);
#1897=CIRCLE('',#11790,0.12645);
#1898=CIRCLE('',#11792,0.1543);
#1899=CIRCLE('',#11800,0.1543);
#1900=CIRCLE('',#11802,0.1543);
#1901=CIRCLE('',#11810,0.1543);
#1902=CIRCLE('',#11813,1.);
#1903=CIRCLE('',#11822,0.6);
#1904=CIRCLE('',#11823,0.399999999999998);
#1905=CIRCLE('',#11824,0.6);
#1906=CIRCLE('',#11826,0.6);
#1907=CIRCLE('',#11828,0.4);
#1908=CIRCLE('',#11829,0.6);
#1909=CIRCLE('',#11831,0.6);
#1910=CIRCLE('',#11833,1.);
#1911=CIRCLE('',#11834,0.6);
#1912=CIRCLE('',#11836,1.);
#1913=CIRCLE('',#11837,0.6);
#1914=CIRCLE('',#11846,1.);
#1915=CIRCLE('',#11848,0.6);
#2282=B_SPLINE_CURVE_WITH_KNOTS('',3,(#24821,#24822,#24823,#24824,#24825,
#24826,#24827,#24828,#24829,#24830,#24831,#24832,#24833,#24834,#24835,#24836,
#24837,#24838,#24839,#24840,#24841,#24842),.UNSPECIFIED.,.F.,.F.,(4,3,3,
3,3,3,3,4),(76.7080459413271,76.8129957196859,77.8105670926688,78.8081384656518,
79.8057098386347,80.8032812116176,81.8008525846005,82.7984239575835),
 .UNSPECIFIED.);
#2283=B_SPLINE_CURVE_WITH_KNOTS('',3,(#24846,#24847,#24848,#24849,#24850,
#24851,#24852),.UNSPECIFIED.,.F.,.F.,(4,3,4),(-80.783811092309,-79.8057098386347,
-79.2446069498474),.UNSPECIFIED.);
#2284=B_SPLINE_CURVE_WITH_KNOTS('',3,(#24856,#24857,#24858,#24859,#24860,
#24861,#24862,#24863,#24864,#24865,#24866,#24867,#24868,#24869,#24870,#24871,
#24872,#24873,#24874,#24875,#24876,#24877),.UNSPECIFIED.,.F.,.F.,(4,3,3,
3,3,3,3,4),(-79.2446069498474,-78.8081384656518,-77.8105670926689,-76.8129957196859,
-75.815424346703,-74.81785297372,-73.8202816007371,-72.9614216426678),
 .UNSPECIFIED.);
#2285=B_SPLINE_CURVE_WITH_KNOTS('',3,(#24882,#24883,#24884,#24885,#24886,
#24887,#24888,#24889,#24890,#24891,#24892,#24893,#24894,#24895,#24896,#24897,
#24898,#24899,#24900,#24901,#24902,#24903),.UNSPECIFIED.,.F.,.F.,(4,3,3,
3,3,3,3,4),(70.4248606341475,70.8275674817883,71.8251388547712,72.8227102277541,
73.8202816007371,74.81785297372,75.815424346703,76.7080459413271),
 .UNSPECIFIED.);
#2286=B_SPLINE_CURVE_WITH_KNOTS('',3,(#24904,#24905,#24906,#24907,#24908,
#24909,#24910,#24911,#24912,#24913,#24914,#24915,#24916,#24917,#24918,#24919,
#24920,#24921,#24922,#24923,#24924,#24925,#24926,#24927,#24928),
 .UNSPECIFIED.,.F.,.F.,(4,3,3,3,3,3,3,3,4),(-72.9614216426678,-72.8227102277542,
-71.8251388547712,-70.8275674817883,-69.8299961088054,-68.8324247358224,
-67.8348533628395,-66.8372819898566,-66.6782363354882),.UNSPECIFIED.);
#2287=B_SPLINE_CURVE_WITH_KNOTS('',3,(#24933,#24934,#24935,#24936,#24937,
#24938,#24939,#24940,#24941,#24942,#24943,#24944,#24945,#24946,#24947,#24948,
#24949,#24950,#24951,#24952,#24953,#24954),.UNSPECIFIED.,.F.,.F.,(4,3,3,
3,3,3,3,4),(64.1416753269679,64.8421392438907,65.8397106168736,66.8372819898565,
67.8348533628395,68.8324247358224,69.8299961088054,70.4248606341475),
 .UNSPECIFIED.);
#2288=B_SPLINE_CURVE_WITH_KNOTS('',3,(#24955,#24956,#24957,#24958,#24959,
#24960,#24961,#24962,#24963,#24964,#24965,#24966,#24967,#24968,#24969,#24970,
#24971,#24972,#24973,#24974,#24975,#24976),.UNSPECIFIED.,.F.,.F.,(4,3,3,
3,3,3,3,4),(-66.6782363354882,-65.8397106168736,-64.8421392438907,-63.8445678709078,
-62.8469964979248,-61.8494251249419,-60.851853751959,-60.3950510283086),
 .UNSPECIFIED.);
#2289=B_SPLINE_CURVE_WITH_KNOTS('',3,(#24981,#24982,#24983,#24984,#24985,
#24986,#24987,#24988,#24989,#24990,#24991,#24992,#24993,#24994,#24995,#24996,
#24997,#24998,#24999,#25000,#25001,#25002),.UNSPECIFIED.,.F.,.F.,(4,3,3,
3,3,3,3,4),(57.8584900197883,58.8567110059931,59.854282378976,60.851853751959,
61.8494251249419,62.8469964979248,63.8445678709078,64.1416753269679),
 .UNSPECIFIED.);
#2290=B_SPLINE_CURVE_WITH_KNOTS('',3,(#25003,#25004,#25005,#25006,#25007,
#25008,#25009,#25010,#25011,#25012,#25013,#25014,#25015,#25016,#25017,#25018,
#25019,#25020,#25021,#25022,#25023,#25024),.UNSPECIFIED.,.F.,.F.,(4,3,3,
3,3,3,3,4),(-60.3950510283086,-59.8542823789761,-58.8567110059931,-57.8591396330102,
-56.8615682600272,-55.8639968870443,-54.8664255140614,-54.111865721129),
 .UNSPECIFIED.);
#2291=B_SPLINE_CURVE_WITH_KNOTS('',3,(#25029,#25030,#25031,#25032,#25033,
#25034,#25035,#25036,#25037,#25038,#25039,#25040,#25041,#25042,#25043,#25044,
#25045,#25046,#25047,#25048,#25049,#25050),.UNSPECIFIED.,.F.,.F.,(4,3,3,
3,3,3,3,4),(51.5753047126088,51.8737113951125,52.8712827680955,53.8688541410784,
54.8664255140613,55.8639968870443,56.8615682600272,57.8584900197883),
 .UNSPECIFIED.);
#2292=B_SPLINE_CURVE_WITH_KNOTS('',3,(#25051,#25052,#25053,#25054,#25055,
#25056,#25057,#25058,#25059,#25060,#25061,#25062,#25063,#25064,#25065,#25066,
#25067,#25068,#25069,#25070,#25071,#25072,#25073,#25074,#25075),
 .UNSPECIFIED.,.F.,.F.,(4,3,3,3,3,3,3,3,4),(-54.111865721129,-53.8688541410784,
-52.8712827680955,-51.8737113951126,-50.8761400221296,-49.8785686491467,
-48.8809972761638,-47.8834259031808,-47.8286804139494),.UNSPECIFIED.);
#2293=B_SPLINE_CURVE_WITH_KNOTS('',3,(#25080,#25081,#25082,#25083,#25084,
#25085,#25086,#25087,#25088,#25089,#25090,#25091,#25092,#25093,#25094,#25095,
#25096,#25097,#25098,#25099,#25100,#25101),.UNSPECIFIED.,.F.,.F.,(4,3,3,
3,3,3,3,4),(45.2921194054292,45.8882831572149,46.8858545301979,47.8834259031808,
48.8809972761637,49.8785686491467,50.8761400221296,51.5753047126088),
 .UNSPECIFIED.);
#2294=B_SPLINE_CURVE_WITH_KNOTS('',3,(#25102,#25103,#25104,#25105,#25106,
#25107,#25108,#25109,#25110,#25111,#25112,#25113,#25114,#25115,#25116,#25117,
#25118,#25119,#25120,#25121,#25122,#25123),.UNSPECIFIED.,.F.,.F.,(4,3,3,
3,3,3,3,4),(-47.8286804139494,-46.8858545301979,-45.888283157215,-44.890711784232,
-43.8931404112491,-42.8955690382662,-41.8979976652832,-41.5454951067698),
 .UNSPECIFIED.);
#2295=B_SPLINE_CURVE_WITH_KNOTS('',3,(#25128,#25129,#25130,#25131,#25132,
#25133,#25134,#25135,#25136,#25137,#25138,#25139,#25140,#25141,#25142,#25143,
#25144,#25145,#25146,#25147,#25148,#25149),.UNSPECIFIED.,.F.,.F.,(4,3,3,
3,3,3,3,4),(39.0089340982495,39.9028549193173,40.9004262923003,41.8979976652832,
42.8955690382661,43.8931404112491,44.890711784232,45.2921194054292),
 .UNSPECIFIED.);
#2296=B_SPLINE_CURVE_WITH_KNOTS('',3,(#25150,#25151,#25152,#25153,#25154,
#25155,#25156,#25157,#25158,#25159,#25160,#25161,#25162,#25163,#25164,#25165,
#25166,#25167,#25168,#25169,#25170,#25171),.UNSPECIFIED.,.F.,.F.,(4,3,3,
3,3,3,3,4),(-41.5454951067698,-40.9004262923003,-39.9028549193174,-38.9052835463344,
-37.9077121733515,-36.9101408003686,-35.9125694273856,-35.2623097995902),
 .UNSPECIFIED.);
#2297=B_SPLINE_CURVE_WITH_KNOTS('',3,(#25176,#25177,#25178,#25179,#25180,
#25181,#25182,#25183,#25184,#25185,#25186,#25187,#25188,#25189,#25190,#25191,
#25192,#25193,#25194,#25195,#25196,#25197,#25198,#25199,#25200),
 .UNSPECIFIED.,.F.,.F.,(4,3,3,3,3,3,3,3,4),(32.7257487910699,32.9198553084368,
33.9174266814197,34.9149980544027,35.9125694273856,36.9101408003685,37.9077121733515,
38.9052835463344,39.0089340982495),.UNSPECIFIED.);
#2298=B_SPLINE_CURVE_WITH_KNOTS('',3,(#25201,#25202,#25203,#25204,#25205,
#25206,#25207,#25208,#25209,#25210,#25211,#25212,#25213,#25214,#25215,#25216,
#25217,#25218,#25219,#25220,#25221,#25222),.UNSPECIFIED.,.F.,.F.,(4,3,3,
3,3,3,3,4),(-35.2623097995902,-34.9149980544027,-33.9174266814197,-32.9198553084368,
-31.9222839354539,-30.924712562471,-29.927141189488,-28.9791244924107),
 .UNSPECIFIED.);
#2299=B_SPLINE_CURVE_WITH_KNOTS('',3,(#25227,#25228,#25229,#25230,#25231,
#25232,#25233,#25234,#25235,#25236,#25237,#25238,#25239,#25240,#25241,#25242,
#25243,#25244,#25245,#25246,#25247,#25248),.UNSPECIFIED.,.F.,.F.,(4,3,3,
3,3,3,3,4),(26.4425634838903,26.9344270705392,27.9319984435221,28.9295698165051,
29.927141189488,30.9247125624709,31.9222839354539,32.7257487910699),
 .UNSPECIFIED.);
#2300=B_SPLINE_CURVE_WITH_KNOTS('',3,(#25249,#25250,#25251,#25252,#25253,
#25254,#25255,#25256,#25257,#25258,#25259,#25260,#25261,#25262,#25263,#25264,
#25265,#25266,#25267,#25268,#25269,#25270,#25271,#25272,#25273),
 .UNSPECIFIED.,.F.,.F.,(4,3,3,3,3,3,3,3,4),(-28.9791244924107,-28.9295698165051,
-27.9319984435222,-26.9344270705392,-25.9368556975563,-24.9392843245734,
-23.9417129515904,-22.9441415786075,-22.6959391852311),.UNSPECIFIED.);
#2301=B_SPLINE_CURVE_WITH_KNOTS('',3,(#25278,#25279,#25280,#25281,#25282,
#25283,#25284,#25285,#25286,#25287,#25288,#25289,#25290,#25291,#25292,#25293,
#25294,#25295,#25296,#25297,#25298,#25299),.UNSPECIFIED.,.F.,.F.,(4,3,3,
3,3,3,3,4),(20.1593781767107,20.9489988326416,21.9465702056245,22.9441415786075,
23.9417129515904,24.9392843245733,25.9368556975563,26.4425634838903),
 .UNSPECIFIED.);
#2302=B_SPLINE_CURVE_WITH_KNOTS('',3,(#25300,#25301,#25302,#25303,#25304,
#25305,#25306,#25307,#25308,#25309,#25310,#25311,#25312,#25313,#25314,#25315,
#25316,#25317,#25318,#25319,#25320,#25321),.UNSPECIFIED.,.F.,.F.,(4,3,3,
3,3,3,3,4),(-22.6959391852311,-21.9465702056245,-20.9489988326416,-19.9514274596587,
-18.9538560866757,-17.9562847136928,-16.9587133407099,-16.4127538780515),
 .UNSPECIFIED.);
#2303=B_SPLINE_CURVE_WITH_KNOTS('',3,(#25326,#25327,#25328,#25329,#25330,
#25331,#25332,#25333,#25334,#25335,#25336,#25337,#25338,#25339,#25340,#25341,
#25342,#25343,#25344,#25345,#25346,#25347,#25348,#25349,#25350),
 .UNSPECIFIED.,.F.,.F.,(4,3,3,3,3,3,3,3,4),(13.8761928695313,13.9659992217611,
14.963570594744,15.9611419677269,16.9587133407099,17.9562847136928,18.9538560866757,
19.9514274596587,20.1593781767107),.UNSPECIFIED.);
#2304=B_SPLINE_CURVE_WITH_KNOTS('',3,(#25351,#25352,#25353,#25354,#25355,
#25356,#25357,#25358,#25359,#25360,#25361,#25362,#25363,#25364,#25365,#25366,
#25367,#25368,#25369,#25370,#25371,#25372),.UNSPECIFIED.,.F.,.F.,(4,3,3,
3,3,3,3,4),(-16.4127538780515,-15.9611419677269,-14.963570594744,-13.9659992217611,
-12.9684278487781,-11.9708564757952,-10.9732851028123,-10.1295685708719),
 .UNSPECIFIED.);
#2305=B_SPLINE_CURVE_WITH_KNOTS('',3,(#25378,#25379,#25380,#25381,#25382,
#25383,#25384,#25385,#25386,#25387,#25388,#25389,#25390),.UNSPECIFIED.,
 .F.,.F.,(4,3,3,3,4),(-3.84638326369226,-2.9927141189488,-1.99514274596587,
-0.997571372982934,0.),.UNSPECIFIED.);
#2306=B_SPLINE_CURVE_WITH_KNOTS('',3,(#25393,#25394,#25395,#25396,#25397,
#25398,#25399,#25400,#25401,#25402,#25403,#25404,#25405,#25406,#25407,#25408,
#25409,#25410,#25411),.UNSPECIFIED.,.F.,.F.,(4,3,3,3,3,3,4),(2.01461286527449,
2.9927141189488,3.99028549193173,4.98785686491467,5.9854282378976,6.98299961088053,
7.59300756235165),.UNSPECIFIED.);
#2307=B_SPLINE_CURVE_WITH_KNOTS('',3,(#25417,#25418,#25419,#25420,#25421,
#25422,#25423),.UNSPECIFIED.,.F.,.F.,(4,1,1,1,4),(91.106186954104,91.6672898428913,
92.6648612158743,93.6624325888572,94.6600039618401),.UNSPECIFIED.);
#2308=B_SPLINE_CURVE_WITH_KNOTS('',3,(#25426,#25427,#25428,#25429,#25430,
#25431,#25432,#25433),.UNSPECIFIED.,.F.,.F.,(4,1,1,1,1,4),(91.106186954104,
91.2111367324627,92.2087081054457,93.2062794784286,94.2038508514115,95.1819521050858),
 .UNSPECIFIED.);
#2309=B_SPLINE_CURVE_WITH_KNOTS('',3,(#25438,#25439,#25440,#25441,#25442,
#25443,#25444,#25445,#25446,#25447),.UNSPECIFIED.,.F.,.F.,(4,1,1,1,1,1,
1,4),(84.8230016469244,85.6818616049937,86.6794329779766,87.6770043509596,
88.6745757239425,89.6721470969255,90.6697184699084,91.106186954104),
 .UNSPECIFIED.);
#2310=B_SPLINE_CURVE_WITH_KNOTS('',3,(#25448,#25449,#25450,#25451,#25452,
#25453,#25454,#25455,#25456,#25457),.UNSPECIFIED.,.F.,.F.,(4,1,1,1,1,1,
1,4),(84.8230016469244,85.2257084945651,86.2232798675481,87.220851240531,
88.2184226135139,89.2159939864968,90.2135653594798,91.106186954104),
 .UNSPECIFIED.);
#2311=B_SPLINE_CURVE_WITH_KNOTS('',3,(#25462,#25463,#25464,#25465,#25466,
#25467,#25468,#25469,#25470,#25471,#25472),.UNSPECIFIED.,.F.,.F.,(4,1,1,
1,1,1,1,1,4),(78.5398163397448,78.6988619941132,79.6964333670961,80.6940047400791,
81.691576113062,82.6891474860449,83.6867188590278,84.6842902320108,84.8230016469244),
 .UNSPECIFIED.);
#2312=B_SPLINE_CURVE_WITH_KNOTS('',3,(#25473,#25474,#25475,#25476,#25477,
#25478,#25479,#25480,#25481,#25482),.UNSPECIFIED.,.F.,.F.,(4,1,1,1,1,1,
1,4),(78.5398163397448,79.2402802566675,80.2378516296505,81.2354230026334,
82.2329943756163,83.2305657485992,84.2281371215822,84.8230016469244),
 .UNSPECIFIED.);
#2313=B_SPLINE_CURVE_WITH_KNOTS('',3,(#25487,#25488,#25489,#25490,#25491,
#25492,#25493,#25494,#25495,#25496),.UNSPECIFIED.,.F.,.F.,(4,1,1,1,1,1,
1,4),(72.2566310325652,72.7134337562156,73.7110051291985,74.7085765021814,
75.7061478751644,76.7037192481473,77.7012906211302,78.5398163397448),
 .UNSPECIFIED.);
#2314=B_SPLINE_CURVE_WITH_KNOTS('',3,(#25497,#25498,#25499,#25500,#25501,
#25502,#25503,#25504,#25505,#25506,#25507),.UNSPECIFIED.,.F.,.F.,(4,1,1,
1,1,1,1,1,4),(72.2566310325652,72.257280645787,73.2548520187699,74.2524233917528,
75.2499947647358,76.2475661377187,77.2451375107017,78.2427088836846,78.5398163397448),
 .UNSPECIFIED.);
#2315=B_SPLINE_CURVE_WITH_KNOTS('',3,(#25512,#25513,#25514,#25515,#25516,
#25517,#25518,#25519,#25520,#25521),.UNSPECIFIED.,.F.,.F.,(4,1,1,1,1,1,
1,4),(65.9734457253856,66.728005518318,67.7255768913009,68.7231482642838,
69.7207196372668,70.7182910102497,71.7158623832326,72.2566310325652),
 .UNSPECIFIED.);
#2316=B_SPLINE_CURVE_WITH_KNOTS('',3,(#25522,#25523,#25524,#25525,#25526,
#25527,#25528,#25529,#25530,#25531),.UNSPECIFIED.,.F.,.F.,(4,1,1,1,1,1,
1,4),(65.9734457253856,66.2718524078894,67.2694237808723,68.2669951538552,
69.2645665268382,70.2621378998211,71.2597092728041,72.2566310325652),
 .UNSPECIFIED.);
#2317=B_SPLINE_CURVE_WITH_KNOTS('',3,(#25536,#25537,#25538,#25539,#25540,
#25541,#25542,#25543,#25544,#25545,#25546),.UNSPECIFIED.,.F.,.F.,(4,1,1,
1,1,1,1,1,4),(59.690260418206,59.7450059074374,60.7425772804204,61.7401486534033,
62.7377200263862,63.7352913993692,64.7328627723521,65.730434145335,65.9734457253856),
 .UNSPECIFIED.);
#2318=B_SPLINE_CURVE_WITH_KNOTS('',3,(#25547,#25548,#25549,#25550,#25551,
#25552,#25553,#25554,#25555,#25556),.UNSPECIFIED.,.F.,.F.,(4,1,1,1,1,1,
1,4),(59.690260418206,60.2864241699918,61.2839955429747,62.2815669159576,
63.2791382889406,64.2767096619235,65.2742810349065,65.9734457253856),
 .UNSPECIFIED.);
#2319=B_SPLINE_CURVE_WITH_KNOTS('',3,(#25561,#25562,#25563,#25564,#25565,
#25566,#25567,#25568,#25569,#25570),.UNSPECIFIED.,.F.,.F.,(4,1,1,1,1,1,
1,4),(53.4070751110264,53.7595776695398,54.7571490425228,55.7547204155057,
56.7522917884886,57.7498631614716,58.7474345344545,59.690260418206),
 .UNSPECIFIED.);
#2320=B_SPLINE_CURVE_WITH_KNOTS('',3,(#25571,#25572,#25573,#25574,#25575,
#25576,#25577,#25578,#25579,#25580),.UNSPECIFIED.,.F.,.F.,(4,1,1,1,1,1,
1,4),(53.4070751110264,54.3009959320942,55.2985673050771,56.29613867806,
57.293710051043,58.2912814240259,59.2888527970089,59.690260418206),
 .UNSPECIFIED.);
#2321=B_SPLINE_CURVE_WITH_KNOTS('',3,(#25585,#25586,#25587,#25588,#25589,
#25590,#25591,#25592,#25593,#25594),.UNSPECIFIED.,.F.,.F.,(4,1,1,1,1,1,
1,4),(47.1238898038468,47.7741494316422,48.7717208046252,49.7692921776081,
50.766863550591,51.764434923574,52.7620062965569,53.4070751110264),
 .UNSPECIFIED.);
#2322=B_SPLINE_CURVE_WITH_KNOTS('',3,(#25595,#25596,#25597,#25598,#25599,
#25600,#25601,#25602,#25603,#25604,#25605),.UNSPECIFIED.,.F.,.F.,(4,1,1,
1,1,1,1,1,4),(47.1238898038468,47.3179963212136,48.3155676941966,49.3131390671795,
50.3107104401624,51.3082818131454,52.3058531861283,53.3034245591112,53.4070751110264),
 .UNSPECIFIED.);
#2323=B_SPLINE_CURVE_WITH_KNOTS('',3,(#25610,#25611,#25612,#25613,#25614,
#25615,#25616,#25617,#25618,#25619),.UNSPECIFIED.,.F.,.F.,(4,1,1,1,1,1,
1,4),(40.8407044966672,41.7887211937446,42.7862925667276,43.7838639397105,
44.7814353126934,45.7790066856764,46.7765780586593,47.1238898038468),
 .UNSPECIFIED.);
#2324=B_SPLINE_CURVE_WITH_KNOTS('',3,(#25620,#25621,#25622,#25623,#25624,
#25625,#25626,#25627,#25628,#25629),.UNSPECIFIED.,.F.,.F.,(4,1,1,1,1,1,
1,4),(40.8407044966672,41.332568083316,42.330139456299,43.3277108292819,
44.3252822022648,45.3228535752478,46.3204249482307,47.1238898038468),
 .UNSPECIFIED.);
#2325=B_SPLINE_CURVE_WITH_KNOTS('',3,(#25634,#25635,#25636,#25637,#25638,
#25639,#25640,#25641,#25642,#25643,#25644),.UNSPECIFIED.,.F.,.F.,(4,1,1,
1,1,1,1,1,4),(34.5575191894877,34.8057215828641,35.803292955847,36.80086432883,
37.7984357018129,38.7960070747958,39.7935784477788,40.7911498207617,40.8407044966672),
 .UNSPECIFIED.);
#2326=B_SPLINE_CURVE_WITH_KNOTS('',3,(#25645,#25646,#25647,#25648,#25649,
#25650,#25651,#25652,#25653,#25654),.UNSPECIFIED.,.F.,.F.,(4,1,1,1,1,1,
1,4),(34.5575191894877,35.3471398454184,36.3447112184014,37.3422825913843,
38.3398539643672,39.3374253373502,40.3349967103331,40.8407044966672),
 .UNSPECIFIED.);
#2327=B_SPLINE_CURVE_WITH_KNOTS('',3,(#25659,#25660,#25661,#25662,#25663,
#25664,#25665,#25666,#25667,#25668),.UNSPECIFIED.,.F.,.F.,(4,1,1,1,1,1,
1,4),(28.2743338823081,28.8202933449665,29.8178647179494,30.8154360909324,
31.8130074639153,32.8105788368982,33.8081502098812,34.5575191894877),
 .UNSPECIFIED.);
#2328=B_SPLINE_CURVE_WITH_KNOTS('',3,(#25669,#25670,#25671,#25672,#25673,
#25674,#25675,#25676,#25677,#25678,#25679),.UNSPECIFIED.,.F.,.F.,(4,1,1,
1,1,1,1,1,4),(28.2743338823081,28.3641402345379,29.3617116075208,30.3592829805038,
31.3568543534867,32.3544257264696,33.3519970994526,34.3495684724355,34.5575191894877),
 .UNSPECIFIED.);
#2329=B_SPLINE_CURVE_WITH_KNOTS('',3,(#25684,#25685,#25686,#25687,#25688,
#25689,#25690,#25691,#25692,#25693),.UNSPECIFIED.,.F.,.F.,(4,1,1,1,1,1,
1,4),(21.9911485751285,22.8348651070689,23.8324364800518,24.8300078530348,
25.8275792260177,26.8251505990006,27.8227219719836,28.2743338823081),
 .UNSPECIFIED.);
#2330=B_SPLINE_CURVE_WITH_KNOTS('',3,(#25694,#25695,#25696,#25697,#25698,
#25699,#25700,#25701,#25702,#25703),.UNSPECIFIED.,.F.,.F.,(4,1,1,1,1,1,
1,4),(21.9911485751285,22.3787119966403,23.3762833696232,24.3738547426062,
25.3714261155891,26.368997488572,27.366568861555,28.2743338823081),
 .UNSPECIFIED.);
#2331=B_SPLINE_CURVE_WITH_KNOTS('',3,(#25709,#25710,#25711,#25712,#25713),
 .UNSPECIFIED.,.F.,.F.,(4,1,4),(14.3981410127768,15.3957123857598,15.7079632679489),
 .UNSPECIFIED.);
#2332=B_SPLINE_CURVE_WITH_KNOTS('',3,(#25716,#25717,#25718,#25719,#25720),
 .UNSPECIFIED.,.F.,.F.,(4,1,4),(13.8761928695311,14.8542941232054,15.7079632679489),
 .UNSPECIFIED.);
#2333=B_SPLINE_CURVE_WITH_KNOTS('',3,(#25726,#25727,#25728,#25729),
 .UNSPECIFIED.,.F.,.F.,(4,4),(51.5750455984138,52.2860549491936),
 .UNSPECIFIED.);
#2334=B_SPLINE_CURVE_WITH_KNOTS('',3,(#25732,#25733,#25734,#25735,#25736,
#25737,#25738,#25739,#25740,#25741),.UNSPECIFIED.,.F.,.F.,(4,3,3,4),(-50.2654824574367,
-49.3264669332015,-48.3399375945375,-47.8348991546268),.UNSPECIFIED.);
#2335=B_SPLINE_CURVE_WITH_KNOTS('',3,(#25746,#25747,#25748,#25749,#25750,
#25751,#25752,#25753,#25754,#25755,#25756,#25757,#25758,#25759,#25760,#25761,
#25762,#25763,#25764,#25765,#25766,#25767,#25768,#25769,#25770),
 .UNSPECIFIED.,.F.,.F.,(4,3,3,3,3,3,3,3,4),(45.2918602912342,45.3803495785454,
46.3668789172094,47.3534082558735,48.3399375945375,49.3264669332015,50.3129962718656,
51.2995256105296,51.5750455984138),.UNSPECIFIED.);
#2336=B_SPLINE_CURVE_WITH_KNOTS('',3,(#25771,#25772,#25773,#25774,#25775,
#25776,#25777,#25778,#25779,#25780,#25781,#25782,#25783,#25784,#25785,#25786,
#25787,#25788,#25789,#25790,#25791,#25792),.UNSPECIFIED.,.F.,.F.,(4,3,3,
3,3,3,3,4),(-47.8348991546268,-47.3534082558735,-46.3668789172095,-45.3803495785454,
-44.3938202398814,-43.4072909012174,-42.4207615625533,-41.5517138474472),
 .UNSPECIFIED.);
#2337=B_SPLINE_CURVE_WITH_KNOTS('',3,(#25797,#25798,#25799,#25800,#25801,
#25802,#25803,#25804,#25805,#25806,#25807,#25808,#25809,#25810,#25811,#25812,
#25813,#25814,#25815,#25816,#25817,#25818),.UNSPECIFIED.,.F.,.F.,(4,3,3,
3,3,3,3,4),(39.0086749840546,39.4611735465612,40.4477028852253,41.4342322238893,
42.4207615625533,43.4072909012174,44.3938202398814,45.2918602912342),
 .UNSPECIFIED.);
#2338=B_SPLINE_CURVE_WITH_KNOTS('',3,(#25819,#25820,#25821,#25822,#25823,
#25824,#25825,#25826,#25827,#25828,#25829,#25830,#25831,#25832,#25833,#25834,
#25835,#25836,#25837,#25838,#25839,#25840,#25841,#25842,#25843),
 .UNSPECIFIED.,.F.,.F.,(4,3,3,3,3,3,3,3,4),(-41.5517138474472,-41.4342322238893,
-40.4477028852253,-39.4611735465612,-38.4746442078972,-37.4881148692332,
-36.5015855305691,-35.5150561919051,-35.2685285402676),.UNSPECIFIED.);
#2339=B_SPLINE_CURVE_WITH_KNOTS('',3,(#25848,#25849,#25850,#25851,#25852,
#25853,#25854,#25855,#25856,#25857,#25858,#25859,#25860,#25861,#25862,#25863,
#25864,#25865,#25866,#25867,#25868,#25869),.UNSPECIFIED.,.F.,.F.,(4,3,3,
3,3,3,3,4),(32.725489676875,33.541997514577,34.5285268532411,35.5150561919051,
36.5015855305691,37.4881148692332,38.4746442078972,39.0086749840546),
 .UNSPECIFIED.);
#2340=B_SPLINE_CURVE_WITH_KNOTS('',3,(#25870,#25871,#25872,#25873,#25874,
#25875,#25876,#25877,#25878,#25879,#25880,#25881,#25882,#25883,#25884,#25885,
#25886,#25887,#25888,#25889,#25890,#25891),.UNSPECIFIED.,.F.,.F.,(4,3,3,
3,3,3,3,4),(-35.2685285402676,-34.5285268532411,-33.541997514577,-32.555468175913,
-31.568938837249,-30.582409498585,-29.5958801599209,-28.985343233088),
 .UNSPECIFIED.);
#2341=B_SPLINE_CURVE_WITH_KNOTS('',3,(#25896,#25897,#25898,#25899,#25900,
#25901,#25902,#25903,#25904,#25905,#25906,#25907,#25908,#25909,#25910,#25911,
#25912,#25913,#25914,#25915,#25916,#25917,#25918,#25919,#25920),
 .UNSPECIFIED.,.F.,.F.,(4,3,3,3,3,3,3,3,4),(26.4423043696954,26.6362921439288,
27.6228214825929,28.6093508212569,29.5958801599209,30.582409498585,31.568938837249,
32.555468175913,32.725489676875),.UNSPECIFIED.);
#2342=B_SPLINE_CURVE_WITH_KNOTS('',3,(#25921,#25922,#25923,#25924,#25925,
#25926,#25927,#25928,#25929,#25930,#25931,#25932,#25933,#25934,#25935,#25936,
#25937,#25938,#25939,#25940,#25941,#25942),.UNSPECIFIED.,.F.,.F.,(4,3,3,
3,3,3,3,4),(-28.985343233088,-28.6093508212569,-27.6228214825929,-26.6362921439288,
-25.6497628052648,-24.6632334666008,-23.6767041279367,-22.7021579259084),
 .UNSPECIFIED.);
#2343=B_SPLINE_CURVE_WITH_KNOTS('',3,(#25947,#25948,#25949,#25950,#25951,
#25952,#25953,#25954,#25955,#25956,#25957,#25958,#25959,#25960,#25961,#25962,
#25963,#25964,#25965,#25966,#25967,#25968),.UNSPECIFIED.,.F.,.F.,(4,3,3,
3,3,3,3,4),(20.1591190625159,20.7171161119446,21.7036454506087,22.6901747892727,
23.6767041279367,24.6632334666008,25.6497628052648,26.4423043696954),
 .UNSPECIFIED.);
#2344=B_SPLINE_CURVE_WITH_KNOTS('',3,(#25969,#25970,#25971,#25972,#25973,
#25974,#25975,#25976,#25977,#25978,#25979,#25980,#25981,#25982,#25983,#25984,
#25985,#25986,#25987,#25988,#25989,#25990,#25991,#25992,#25993),
 .UNSPECIFIED.,.F.,.F.,(4,3,3,3,3,3,3,3,4),(-22.7021579259084,-22.6901747892727,
-21.7036454506087,-20.7171161119446,-19.7305867732806,-18.7440574346166,
-17.7575280959526,-16.7709987572885,-16.4189726187288),.UNSPECIFIED.);
#2345=B_SPLINE_CURVE_WITH_KNOTS('',3,(#25998,#25999,#26000,#26001,#26002,
#26003,#26004,#26005,#26006,#26007,#26008,#26009,#26010,#26011,#26012,#26013,
#26014,#26015,#26016,#26017,#26018,#26019),.UNSPECIFIED.,.F.,.F.,(4,3,3,
3,3,3,3,4),(13.8759337553363,14.7979400799605,15.7844694186245,16.7709987572885,
17.7575280959526,18.7440574346166,19.7305867732806,20.1591190625159),
 .UNSPECIFIED.);
#2346=B_SPLINE_CURVE_WITH_KNOTS('',3,(#26020,#26021,#26022,#26023,#26024,
#26025,#26026,#26027,#26028,#26029,#26030,#26031,#26032,#26033,#26034,#26035,
#26036,#26037,#26038,#26039,#26040,#26041),.UNSPECIFIED.,.F.,.F.,(4,3,3,
3,3,3,3,4),(-16.4189726187288,-15.7844694186245,-14.7979400799605,-13.8114107412964,
-12.8248814026324,-11.8383520639684,-10.8518227253043,-10.1357873115492),
 .UNSPECIFIED.);
#2347=B_SPLINE_CURVE_WITH_KNOTS('',3,(#26047,#26048,#26049,#26050,#26051,
#26052,#26053,#26054,#26055,#26056,#26057,#26058,#26059),.UNSPECIFIED.,
 .F.,.F.,(4,3,3,3,4),(-3.85260200436966,-2.95958801599209,-1.97305867732806,
-0.986529338664031,0.),.UNSPECIFIED.);
#2348=B_SPLINE_CURVE_WITH_KNOTS('',3,(#26062,#26063,#26064,#26065,#26066,
#26067,#26068,#26069,#26070,#26071,#26072,#26073,#26074,#26075,#26076,#26077,
#26078,#26079,#26080),.UNSPECIFIED.,.F.,.F.,(4,3,3,3,3,3,4),(2.0205724917569,
2.95958801599209,3.94611735465613,4.93264669332016,5.91917603198418,6.90570537064821,
7.5927484481567),.UNSPECIFIED.);
#2349=B_SPLINE_CURVE_WITH_KNOTS('',3,(#26086,#26087,#26088,#26089),
 .UNSPECIFIED.,.F.,.F.,(4,4),(51.5750455984138,52.2860549491936),
 .UNSPECIFIED.);
#2350=B_SPLINE_CURVE_WITH_KNOTS('',3,(#26092,#26093,#26094,#26095,#26096,
#26097,#26098,#26099,#26100,#26101),.UNSPECIFIED.,.F.,.F.,(4,3,3,4),(-50.2654824574367,
-49.3264669332015,-48.3399375945375,-47.8348991546268),.UNSPECIFIED.);
#2351=B_SPLINE_CURVE_WITH_KNOTS('',3,(#26106,#26107,#26108,#26109,#26110,
#26111,#26112,#26113,#26114,#26115,#26116,#26117,#26118,#26119,#26120,#26121,
#26122,#26123,#26124,#26125,#26126,#26127,#26128,#26129,#26130),
 .UNSPECIFIED.,.F.,.F.,(4,3,3,3,3,3,3,3,4),(45.2918602912342,45.3803495785454,
46.3668789172094,47.3534082558735,48.3399375945375,49.3264669332015,50.3129962718656,
51.2995256105296,51.5750455984138),.UNSPECIFIED.);
#2352=B_SPLINE_CURVE_WITH_KNOTS('',3,(#26131,#26132,#26133,#26134,#26135,
#26136,#26137,#26138,#26139,#26140,#26141,#26142,#26143,#26144,#26145,#26146,
#26147,#26148,#26149,#26150,#26151,#26152),.UNSPECIFIED.,.F.,.F.,(4,3,3,
3,3,3,3,4),(-47.8348991546268,-47.3534082558735,-46.3668789172095,-45.3803495785454,
-44.3938202398814,-43.4072909012174,-42.4207615625533,-41.5517138474472),
 .UNSPECIFIED.);
#2353=B_SPLINE_CURVE_WITH_KNOTS('',3,(#26157,#26158,#26159,#26160,#26161,
#26162,#26163,#26164,#26165,#26166,#26167,#26168,#26169,#26170,#26171,#26172,
#26173,#26174,#26175,#26176,#26177,#26178),.UNSPECIFIED.,.F.,.F.,(4,3,3,
3,3,3,3,4),(39.0086749840546,39.4611735465612,40.4477028852253,41.4342322238893,
42.4207615625533,43.4072909012174,44.3938202398814,45.2918602912342),
 .UNSPECIFIED.);
#2354=B_SPLINE_CURVE_WITH_KNOTS('',3,(#26179,#26180,#26181,#26182,#26183,
#26184,#26185,#26186,#26187,#26188,#26189,#26190,#26191,#26192,#26193,#26194,
#26195,#26196,#26197,#26198,#26199,#26200,#26201,#26202,#26203),
 .UNSPECIFIED.,.F.,.F.,(4,3,3,3,3,3,3,3,4),(-41.5517138474472,-41.4342322238893,
-40.4477028852253,-39.4611735465612,-38.4746442078972,-37.4881148692332,
-36.5015855305691,-35.5150561919051,-35.2685285402676),.UNSPECIFIED.);
#2355=B_SPLINE_CURVE_WITH_KNOTS('',3,(#26208,#26209,#26210,#26211,#26212,
#26213,#26214,#26215,#26216,#26217,#26218,#26219,#26220,#26221,#26222,#26223,
#26224,#26225,#26226,#26227,#26228,#26229),.UNSPECIFIED.,.F.,.F.,(4,3,3,
3,3,3,3,4),(32.725489676875,33.541997514577,34.5285268532411,35.5150561919051,
36.5015855305691,37.4881148692332,38.4746442078972,39.0086749840546),
 .UNSPECIFIED.);
#2356=B_SPLINE_CURVE_WITH_KNOTS('',3,(#26230,#26231,#26232,#26233,#26234,
#26235,#26236,#26237,#26238,#26239,#26240,#26241,#26242,#26243,#26244,#26245,
#26246,#26247,#26248,#26249,#26250,#26251),.UNSPECIFIED.,.F.,.F.,(4,3,3,
3,3,3,3,4),(-35.2685285402676,-34.5285268532411,-33.541997514577,-32.555468175913,
-31.568938837249,-30.582409498585,-29.5958801599209,-28.985343233088),
 .UNSPECIFIED.);
#2357=B_SPLINE_CURVE_WITH_KNOTS('',3,(#26256,#26257,#26258,#26259,#26260,
#26261,#26262,#26263,#26264,#26265,#26266,#26267,#26268,#26269,#26270,#26271,
#26272,#26273,#26274,#26275,#26276,#26277,#26278,#26279,#26280),
 .UNSPECIFIED.,.F.,.F.,(4,3,3,3,3,3,3,3,4),(26.4423043696954,26.6362921439288,
27.6228214825929,28.6093508212569,29.5958801599209,30.582409498585,31.568938837249,
32.555468175913,32.725489676875),.UNSPECIFIED.);
#2358=B_SPLINE_CURVE_WITH_KNOTS('',3,(#26281,#26282,#26283,#26284,#26285,
#26286,#26287,#26288,#26289,#26290,#26291,#26292,#26293,#26294,#26295,#26296,
#26297,#26298,#26299,#26300,#26301,#26302),.UNSPECIFIED.,.F.,.F.,(4,3,3,
3,3,3,3,4),(-28.985343233088,-28.6093508212569,-27.6228214825929,-26.6362921439288,
-25.6497628052648,-24.6632334666008,-23.6767041279367,-22.7021579259084),
 .UNSPECIFIED.);
#2359=B_SPLINE_CURVE_WITH_KNOTS('',3,(#26307,#26308,#26309,#26310,#26311,
#26312,#26313,#26314,#26315,#26316,#26317,#26318,#26319,#26320,#26321,#26322,
#26323,#26324,#26325,#26326,#26327,#26328),.UNSPECIFIED.,.F.,.F.,(4,3,3,
3,3,3,3,4),(20.1591190625159,20.7171161119446,21.7036454506087,22.6901747892727,
23.6767041279367,24.6632334666008,25.6497628052648,26.4423043696954),
 .UNSPECIFIED.);
#2360=B_SPLINE_CURVE_WITH_KNOTS('',3,(#26329,#26330,#26331,#26332,#26333,
#26334,#26335,#26336,#26337,#26338,#26339,#26340,#26341,#26342,#26343,#26344,
#26345,#26346,#26347,#26348,#26349,#26350,#26351,#26352,#26353),
 .UNSPECIFIED.,.F.,.F.,(4,3,3,3,3,3,3,3,4),(-22.7021579259084,-22.6901747892727,
-21.7036454506087,-20.7171161119446,-19.7305867732806,-18.7440574346166,
-17.7575280959526,-16.7709987572885,-16.4189726187288),.UNSPECIFIED.);
#2361=B_SPLINE_CURVE_WITH_KNOTS('',3,(#26358,#26359,#26360,#26361,#26362,
#26363,#26364,#26365,#26366,#26367,#26368,#26369,#26370,#26371,#26372,#26373,
#26374,#26375,#26376,#26377,#26378,#26379),.UNSPECIFIED.,.F.,.F.,(4,3,3,
3,3,3,3,4),(13.8759337553363,14.7979400799605,15.7844694186245,16.7709987572885,
17.7575280959526,18.7440574346166,19.7305867732806,20.1591190625159),
 .UNSPECIFIED.);
#2362=B_SPLINE_CURVE_WITH_KNOTS('',3,(#26380,#26381,#26382,#26383,#26384,
#26385,#26386,#26387,#26388,#26389,#26390,#26391,#26392,#26393,#26394,#26395,
#26396,#26397,#26398,#26399,#26400,#26401),.UNSPECIFIED.,.F.,.F.,(4,3,3,
3,3,3,3,4),(-16.4189726187288,-15.7844694186245,-14.7979400799605,-13.8114107412964,
-12.8248814026324,-11.8383520639684,-10.8518227253043,-10.1357873115492),
 .UNSPECIFIED.);
#2363=B_SPLINE_CURVE_WITH_KNOTS('',3,(#26407,#26408,#26409,#26410,#26411,
#26412,#26413,#26414,#26415,#26416,#26417,#26418,#26419),.UNSPECIFIED.,
 .F.,.F.,(4,3,3,3,4),(-3.85260200436966,-2.95958801599209,-1.97305867732806,
-0.986529338664031,0.),.UNSPECIFIED.);
#2364=B_SPLINE_CURVE_WITH_KNOTS('',3,(#26422,#26423,#26424,#26425,#26426,
#26427,#26428,#26429,#26430,#26431,#26432,#26433,#26434,#26435,#26436,#26437,
#26438,#26439,#26440),.UNSPECIFIED.,.F.,.F.,(4,3,3,3,3,3,4),(2.0205724917569,
2.95958801599209,3.94611735465612,4.93264669332016,5.91917603198418,6.90570537064822,
7.5927484481567),.UNSPECIFIED.);
#2365=B_SPLINE_CURVE_WITH_KNOTS('',3,(#26446,#26447,#26448,#26449,#26450,
#26451,#26452,#26453),.UNSPECIFIED.,.F.,.F.,(4,1,1,1,1,4),(59.6902604182061,
60.1952988581168,61.1818281967808,62.1683575354449,63.1548868741089,64.1414162127729),
 .UNSPECIFIED.);
#2366=B_SPLINE_CURVE_WITH_KNOTS('',3,(#26456,#26457,#26458,#26459,#26460,
#26461,#26462,#26463,#26464),.UNSPECIFIED.,.F.,.F.,(4,1,1,1,1,1,4),(59.6902604182061,
59.7787497055172,60.7652790441813,61.7518083828453,62.7383377215093,63.7248670601734,
64.6638825844086),.UNSPECIFIED.);
#2367=B_SPLINE_CURVE_WITH_KNOTS('',3,(#26469,#26470,#26471,#26472,#26473,
#26474,#26475,#26476,#26477,#26478),.UNSPECIFIED.,.F.,.F.,(4,1,1,1,1,1,
1,4),(53.4070751110265,54.2761228261326,55.2626521647967,56.2491815034607,
57.2357108421247,58.2222401807888,59.2087695194528,59.6902604182061),
 .UNSPECIFIED.);
#2368=B_SPLINE_CURVE_WITH_KNOTS('',3,(#26479,#26480,#26481,#26482,#26483,
#26484,#26485,#26486,#26487,#26488),.UNSPECIFIED.,.F.,.F.,(4,1,1,1,1,1,
1,4),(53.4070751110265,53.8595736735331,54.8461030121971,55.8326323508611,
56.8191616895251,57.8056910281892,58.7922203668532,59.6902604182061),
 .UNSPECIFIED.);
#2369=B_SPLINE_CURVE_WITH_KNOTS('',3,(#26493,#26494,#26495,#26496,#26497,
#26498,#26499,#26500,#26501,#26502,#26503),.UNSPECIFIED.,.F.,.F.,(4,1,1,
1,1,1,1,1,4),(47.1238898038469,47.3704174554844,48.3569467941484,49.3434761328125,
50.3300054714765,51.3165348101405,52.3030641488046,53.2895934874686,53.4070751110265),
 .UNSPECIFIED.);
#2370=B_SPLINE_CURVE_WITH_KNOTS('',3,(#26504,#26505,#26506,#26507,#26508,
#26509,#26510,#26511,#26512,#26513),.UNSPECIFIED.,.F.,.F.,(4,1,1,1,1,1,
1,4),(47.1238898038469,47.9403976415489,48.9269269802129,49.9134563188769,
50.899985657541,51.886514996205,52.873044334869,53.4070751110265),
 .UNSPECIFIED.);
#2371=B_SPLINE_CURVE_WITH_KNOTS('',3,(#26518,#26519,#26520,#26521,#26522,
#26523,#26524,#26525,#26526,#26527),.UNSPECIFIED.,.F.,.F.,(4,1,1,1,1,1,
1,4),(40.8407044966673,41.4512414235002,42.4377707621643,43.4243001008283,
44.4108294394923,45.3973587781563,46.3838881168204,47.1238898038469),
 .UNSPECIFIED.);
#2372=B_SPLINE_CURVE_WITH_KNOTS('',3,(#26528,#26529,#26530,#26531,#26532,
#26533,#26534,#26535,#26536,#26537,#26538),.UNSPECIFIED.,.F.,.F.,(4,1,1,
1,1,1,1,1,4),(40.8407044966673,41.0346922709007,42.0212216095647,43.0077509482287,
43.9942802868928,44.9808096255568,45.9673389642208,46.9538683028848,47.1238898038469),
 .UNSPECIFIED.);
#2373=B_SPLINE_CURVE_WITH_KNOTS('',3,(#26543,#26544,#26545,#26546,#26547,
#26548,#26549,#26550,#26551,#26552),.UNSPECIFIED.,.F.,.F.,(4,1,1,1,1,1,
1,4),(34.5575191894877,35.532065391516,36.5185947301801,37.5051240688441,
38.4916534075081,39.4781827461722,40.4647120848362,40.8407044966673),
 .UNSPECIFIED.);
#2374=B_SPLINE_CURVE_WITH_KNOTS('',3,(#26553,#26554,#26555,#26556,#26557,
#26558,#26559,#26560,#26561,#26562),.UNSPECIFIED.,.F.,.F.,(4,1,1,1,1,1,
1,4),(34.5575191894877,35.1155162389165,36.1020455775805,37.0885749162445,
38.0751042549086,39.0616335935726,40.0481629322366,40.8407044966673),
 .UNSPECIFIED.);
#2375=B_SPLINE_CURVE_WITH_KNOTS('',3,(#26567,#26568,#26569,#26570,#26571,
#26572,#26573,#26574,#26575,#26576,#26577),.UNSPECIFIED.,.F.,.F.,(4,1,1,
1,1,1,1,1,4),(28.2743338823081,28.6263600208678,29.6128893595319,30.5994186981959,
31.5859480368599,32.5724773755239,33.559006714188,34.545536052852,34.5575191894877),
 .UNSPECIFIED.);
#2376=B_SPLINE_CURVE_WITH_KNOTS('',3,(#26578,#26579,#26580,#26581,#26582,
#26583,#26584,#26585,#26586,#26587),.UNSPECIFIED.,.F.,.F.,(4,1,1,1,1,1,
1,4),(28.2743338823081,29.1963402069323,30.1828695455963,31.1693988842604,
32.1559282229244,33.1424575615884,34.1289869002524,34.5575191894877),
 .UNSPECIFIED.);
#2377=B_SPLINE_CURVE_WITH_KNOTS('',3,(#26592,#26593,#26594,#26595,#26596,
#26597,#26598,#26599,#26600,#26601),.UNSPECIFIED.,.F.,.F.,(4,1,1,1,1,1,
1,4),(21.9911485751285,22.7071839888836,23.6937133275477,24.6802426662117,
25.6667720048757,26.6533013435398,27.6398306822038,28.2743338823081),
 .UNSPECIFIED.);
#2378=B_SPLINE_CURVE_WITH_KNOTS('',3,(#26602,#26603,#26604,#26605,#26606,
#26607,#26608,#26609,#26610,#26611,#26612),.UNSPECIFIED.,.F.,.F.,(4,1,1,
1,1,1,1,1,4),(21.9911485751285,22.2906348362841,23.2771641749481,24.2636935136121,
25.2502228522762,26.2367521909402,27.2232815296042,28.2098108682683,28.2743338823081),
 .UNSPECIFIED.);
#2379=B_SPLINE_CURVE_WITH_KNOTS('',3,(#26618,#26619,#26620,#26621,#26622),
 .UNSPECIFIED.,.F.,.F.,(4,1,4),(14.3984001269718,15.3849294656359,15.707963267949),
 .UNSPECIFIED.);
#2380=B_SPLINE_CURVE_WITH_KNOTS('',3,(#26625,#26626,#26627,#26628,#26629),
 .UNSPECIFIED.,.F.,.F.,(4,1,4),(13.8759337553362,14.8149492795714,15.7079632679489),
 .UNSPECIFIED.);
#2381=B_SPLINE_CURVE_WITH_KNOTS('',3,(#26635,#26636,#26637,#26638,#26639,
#26640,#26641,#26642),.UNSPECIFIED.,.F.,.F.,(4,1,1,1,1,4),(59.6902604182061,
60.1952988581168,61.1818281967808,62.1683575354449,63.1548868741089,64.1414162127729),
 .UNSPECIFIED.);
#2382=B_SPLINE_CURVE_WITH_KNOTS('',3,(#26645,#26646,#26647,#26648,#26649,
#26650,#26651,#26652,#26653),.UNSPECIFIED.,.F.,.F.,(4,1,1,1,1,1,4),(59.6902604182061,
59.7787497055172,60.7652790441813,61.7518083828453,62.7383377215093,63.7248670601734,
64.6638825844086),.UNSPECIFIED.);
#2383=B_SPLINE_CURVE_WITH_KNOTS('',3,(#26658,#26659,#26660,#26661,#26662,
#26663,#26664,#26665,#26666,#26667),.UNSPECIFIED.,.F.,.F.,(4,1,1,1,1,1,
1,4),(53.4070751110265,54.2761228261326,55.2626521647967,56.2491815034607,
57.2357108421247,58.2222401807888,59.2087695194528,59.6902604182061),
 .UNSPECIFIED.);
#2384=B_SPLINE_CURVE_WITH_KNOTS('',3,(#26668,#26669,#26670,#26671,#26672,
#26673,#26674,#26675,#26676,#26677),.UNSPECIFIED.,.F.,.F.,(4,1,1,1,1,1,
1,4),(53.4070751110265,53.8595736735331,54.8461030121971,55.8326323508611,
56.8191616895251,57.8056910281892,58.7922203668532,59.6902604182061),
 .UNSPECIFIED.);
#2385=B_SPLINE_CURVE_WITH_KNOTS('',3,(#26682,#26683,#26684,#26685,#26686,
#26687,#26688,#26689,#26690,#26691,#26692),.UNSPECIFIED.,.F.,.F.,(4,1,1,
1,1,1,1,1,4),(47.1238898038469,47.3704174554844,48.3569467941484,49.3434761328125,
50.3300054714765,51.3165348101405,52.3030641488046,53.2895934874686,53.4070751110265),
 .UNSPECIFIED.);
#2386=B_SPLINE_CURVE_WITH_KNOTS('',3,(#26693,#26694,#26695,#26696,#26697,
#26698,#26699,#26700,#26701,#26702),.UNSPECIFIED.,.F.,.F.,(4,1,1,1,1,1,
1,4),(47.1238898038469,47.9403976415489,48.9269269802129,49.9134563188769,
50.899985657541,51.886514996205,52.873044334869,53.4070751110265),
 .UNSPECIFIED.);
#2387=B_SPLINE_CURVE_WITH_KNOTS('',3,(#26707,#26708,#26709,#26710,#26711,
#26712,#26713,#26714,#26715,#26716),.UNSPECIFIED.,.F.,.F.,(4,1,1,1,1,1,
1,4),(40.8407044966673,41.4512414235002,42.4377707621643,43.4243001008283,
44.4108294394923,45.3973587781563,46.3838881168204,47.1238898038469),
 .UNSPECIFIED.);
#2388=B_SPLINE_CURVE_WITH_KNOTS('',3,(#26717,#26718,#26719,#26720,#26721,
#26722,#26723,#26724,#26725,#26726,#26727),.UNSPECIFIED.,.F.,.F.,(4,1,1,
1,1,1,1,1,4),(40.8407044966673,41.0346922709007,42.0212216095647,43.0077509482287,
43.9942802868928,44.9808096255568,45.9673389642208,46.9538683028848,47.1238898038469),
 .UNSPECIFIED.);
#2389=B_SPLINE_CURVE_WITH_KNOTS('',3,(#26732,#26733,#26734,#26735,#26736,
#26737,#26738,#26739,#26740,#26741),.UNSPECIFIED.,.F.,.F.,(4,1,1,1,1,1,
1,4),(34.5575191894877,35.532065391516,36.5185947301801,37.5051240688441,
38.4916534075081,39.4781827461722,40.4647120848362,40.8407044966673),
 .UNSPECIFIED.);
#2390=B_SPLINE_CURVE_WITH_KNOTS('',3,(#26742,#26743,#26744,#26745,#26746,
#26747,#26748,#26749,#26750,#26751),.UNSPECIFIED.,.F.,.F.,(4,1,1,1,1,1,
1,4),(34.5575191894877,35.1155162389165,36.1020455775805,37.0885749162445,
38.0751042549086,39.0616335935726,40.0481629322366,40.8407044966673),
 .UNSPECIFIED.);
#2391=B_SPLINE_CURVE_WITH_KNOTS('',3,(#26756,#26757,#26758,#26759,#26760,
#26761,#26762,#26763,#26764,#26765,#26766),.UNSPECIFIED.,.F.,.F.,(4,1,1,
1,1,1,1,1,4),(28.2743338823081,28.6263600208678,29.6128893595319,30.5994186981959,
31.5859480368599,32.5724773755239,33.559006714188,34.545536052852,34.5575191894877),
 .UNSPECIFIED.);
#2392=B_SPLINE_CURVE_WITH_KNOTS('',3,(#26767,#26768,#26769,#26770,#26771,
#26772,#26773,#26774,#26775,#26776),.UNSPECIFIED.,.F.,.F.,(4,1,1,1,1,1,
1,4),(28.2743338823081,29.1963402069323,30.1828695455963,31.1693988842604,
32.1559282229244,33.1424575615884,34.1289869002524,34.5575191894877),
 .UNSPECIFIED.);
#2393=B_SPLINE_CURVE_WITH_KNOTS('',3,(#26781,#26782,#26783,#26784,#26785,
#26786,#26787,#26788,#26789,#26790),.UNSPECIFIED.,.F.,.F.,(4,1,1,1,1,1,
1,4),(21.9911485751285,22.7071839888836,23.6937133275477,24.6802426662117,
25.6667720048757,26.6533013435398,27.6398306822038,28.2743338823081),
 .UNSPECIFIED.);
#2394=B_SPLINE_CURVE_WITH_KNOTS('',3,(#26791,#26792,#26793,#26794,#26795,
#26796,#26797,#26798,#26799,#26800,#26801),.UNSPECIFIED.,.F.,.F.,(4,1,1,
1,1,1,1,1,4),(21.9911485751285,22.2906348362841,23.2771641749481,24.2636935136121,
25.2502228522762,26.2367521909402,27.2232815296042,28.2098108682683,28.2743338823081),
 .UNSPECIFIED.);
#2395=B_SPLINE_CURVE_WITH_KNOTS('',3,(#26807,#26808,#26809,#26810,#26811),
 .UNSPECIFIED.,.F.,.F.,(4,1,4),(14.3984001269718,15.3849294656359,15.707963267949),
 .UNSPECIFIED.);
#2396=B_SPLINE_CURVE_WITH_KNOTS('',3,(#26814,#26815,#26816,#26817,#26818),
 .UNSPECIFIED.,.F.,.F.,(4,1,4),(13.8759337553362,14.8149492795714,15.7079632679489),
 .UNSPECIFIED.);
#2397=B_SPLINE_CURVE_WITH_KNOTS('',3,(#26820,#26821,#26822,#26823,#26824,
#26825,#26826,#26827,#26828,#26829,#26830),.UNSPECIFIED.,.F.,.F.,(4,1,1,
1,1,1,1,1,4),(15.7079632679489,15.8014786182354,16.7880079568995,17.7745372955635,
18.7610666342275,19.7475959728915,20.7341253115556,21.7206546502196,21.9911485751285),
 .UNSPECIFIED.);
#2398=B_SPLINE_CURVE_WITH_KNOTS('',3,(#26831,#26832,#26833,#26834,#26835,
#26836,#26837,#26838,#26839,#26840),.UNSPECIFIED.,.F.,.F.,(4,1,1,1,1,1,
1,4),(15.707963267949,16.3714588042999,17.3579881429639,18.344517481628,
19.331046820292,20.317576158956,21.30410549762,21.9911485751285),
 .UNSPECIFIED.);
#2399=B_SPLINE_CURVE_WITH_KNOTS('',3,(#27065,#27066,#27067,#27068,#27069,
#27070,#27071,#27072,#27073,#27074,#27075,#27076,#27077,#27078,#27079,#27080,
#27081,#27082,#27083,#27084,#27085,#27086,#27087,#27088,#27089,#27090,#27091,
#27092,#27093,#27094,#27095,#27096,#27097,#27098,#27099,#27100,#27101,#27102,
#27103,#27104,#27105,#27106,#27107,#27108,#27109,#27110,#27111,#27112,#27113,
#27114,#27115,#27116),.UNSPECIFIED.,.F.,.F.,(4,3,3,3,3,3,3,3,3,3,3,3,3,
3,3,3,3,4),(0.,0.0320331684328983,0.047982254793735,0.0587463569853809,
0.068374331906695,0.0996455206564278,0.112637667143497,0.122453511831961,
0.146764141737192,0.169126652772842,0.178509832567225,0.203948034872107,
0.222826517887668,0.233934300135679,0.251364503567911,0.26339901807632,
0.280262641786753,0.286347380332264),.UNSPECIFIED.);
#2400=B_SPLINE_CURVE_WITH_KNOTS('',3,(#27117,#27118,#27119,#27120,#27121,
#27122,#27123,#27124,#27125,#27126,#27127,#27128,#27129,#27130,#27131,#27132,
#27133,#27134,#27135,#27136,#27137,#27138,#27139,#27140,#27141,#27142,#27143,
#27144,#27145,#27146,#27147,#27148,#27149,#27150,#27151,#27152,#27153,#27154,
#27155,#27156,#27157,#27158,#27159,#27160,#27161,#27162,#27163,#27164,#27165),
 .UNSPECIFIED.,.F.,.F.,(4,3,3,3,3,3,3,3,3,3,3,3,3,3,3,3,4),(0.,0.0274255978447832,
0.048809316595412,0.0580010326491972,0.0875347374149519,0.101224292480011,
0.111280556216297,0.132431451325231,0.155780476821444,0.165670961223459,
0.193708256295631,0.208717590629974,0.219760914288732,0.239138299607853,
0.257256761910142,0.277820141512149,0.28514280399518),.UNSPECIFIED.);
#2401=B_SPLINE_CURVE_WITH_KNOTS('',3,(#27166,#27167,#27168,#27169,#27170,
#27171,#27172,#27173,#27174,#27175,#27176,#27177,#27178,#27179,#27180,#27181,
#27182,#27183,#27184,#27185,#27186,#27187,#27188,#27189,#27190),
 .UNSPECIFIED.,.F.,.F.,(4,3,3,3,3,3,3,3,4),(-10.1357873115492,-9.8652933866403,
-8.87876404797627,-7.89223470931224,-6.90570537064821,-5.91917603198418,
-4.93264669332015,-3.94611735465612,-3.85260200436966),.UNSPECIFIED.);
#2402=B_SPLINE_CURVE_WITH_KNOTS('',3,(#27415,#27416,#27417,#27418,#27419,
#27420,#27421,#27422,#27423,#27424,#27425,#27426,#27427,#27428,#27429,#27430,
#27431,#27432,#27433,#27434,#27435,#27436,#27437,#27438,#27439,#27440,#27441,
#27442,#27443,#27444,#27445,#27446,#27447,#27448,#27449,#27450,#27451,#27452,
#27453,#27454,#27455,#27456,#27457,#27458,#27459,#27460,#27461,#27462,#27463),
 .UNSPECIFIED.,.F.,.F.,(4,3,3,3,3,3,3,3,3,3,3,3,3,3,3,3,4),(0.,0.0274255913653339,
0.0488093131133246,0.0580010269694127,0.0875347308595416,0.101224269152377,
0.111280553657591,0.132431451325227,0.155780477659062,0.165670961808075,
0.193708256734092,0.208717605217266,0.21976091765614,0.239138308570995,
0.257256762582239,0.277820141512144,0.28514280399514),.UNSPECIFIED.);
#2403=B_SPLINE_CURVE_WITH_KNOTS('',3,(#27464,#27465,#27466,#27467,#27468,
#27469,#27470,#27471,#27472,#27473,#27474,#27475,#27476,#27477,#27478,#27479,
#27480,#27481,#27482,#27483,#27484,#27485,#27486,#27487,#27488),
 .UNSPECIFIED.,.F.,.F.,(4,3,3,3,3,3,3,3,4),(7.5927484481567,7.89223470931224,
8.87876404797628,9.86529338664031,10.8518227253043,11.8383520639684,12.8248814026324,
13.8114107412964,13.8759337553363),.UNSPECIFIED.);
#2404=B_SPLINE_CURVE_WITH_KNOTS('',3,(#27489,#27490,#27491,#27492,#27493,
#27494,#27495,#27496,#27497,#27498,#27499,#27500,#27501,#27502,#27503,#27504,
#27505,#27506,#27507,#27508,#27509,#27510,#27511,#27512,#27513,#27514,#27515,
#27516,#27517,#27518,#27519,#27520,#27521,#27522,#27523,#27524,#27525,#27526,
#27527,#27528,#27529,#27530,#27531,#27532,#27533,#27534,#27535,#27536,#27537,
#27538,#27539,#27540),.UNSPECIFIED.,.F.,.F.,(4,3,3,3,3,3,3,3,3,3,3,3,3,
3,3,3,3,4),(0.,0.0320331645440323,0.0479822944538874,0.0587463983360561,
0.0683743388328265,0.0996455292883743,0.112637688108393,0.122453518454582,
0.146764141737195,0.169126651893336,0.178509831787203,0.20394803428708,
0.222826505940554,0.233934299906464,0.251364515046202,0.263399023832158,
0.280262641786714,0.28634738033223),.UNSPECIFIED.);
#2405=B_SPLINE_CURVE_WITH_KNOTS('',3,(#27554,#27555,#27556,#27557,#27558,
#27559,#27560,#27561,#27562,#27563,#27564,#27565,#27566,#27567,#27568,#27569,
#27570,#27571,#27572,#27573,#27574,#27575,#27576,#27577,#27578,#27579,#27580,
#27581,#27582,#27583,#27584,#27585,#27586,#27587,#27588,#27589,#27590,#27591,
#27592,#27593,#27594,#27595,#27596,#27597,#27598,#27599,#27600,#27601,#27602),
 .UNSPECIFIED.,.F.,.F.,(4,3,3,3,3,3,3,3,3,3,3,3,3,3,3,3,4),(0.,0.0274256070877454,
0.0488093215641943,0.0580010407627361,0.0875347467776894,0.101224325795315,
0.111280559869577,0.132431451325226,0.155780475624762,0.165670960389251,
0.193708255669975,0.208717569845021,0.219760909477782,0.239138286790648,
0.257256760954527,0.277820141512144,0.285142803995137),.UNSPECIFIED.);
#2406=B_SPLINE_CURVE_WITH_KNOTS('',3,(#27603,#27604,#27605,#27606,#27607,
#27608,#27609,#27610,#27611,#27612,#27613,#27614,#27615,#27616,#27617,#27618,
#27619,#27620,#27621,#27622,#27623,#27624,#27625,#27626,#27627,#27628,#27629,
#27630,#27631,#27632,#27633,#27634,#27635,#27636,#27637,#27638,#27639,#27640,
#27641,#27642,#27643,#27644,#27645,#27646,#27647,#27648,#27649,#27650,#27651,
#27652,#27653,#27654),.UNSPECIFIED.,.F.,.F.,(4,3,3,3,3,3,3,3,3,3,3,3,3,
3,3,3,3,4),(0.,0.032033144059138,0.0479825033685422,0.058746616231457,0.068374375333449,
0.0996455747709087,0.112637798572108,0.122453553351573,0.146764141737196,
0.169126647261903,0.17850982771232,0.203948031230928,0.22282644299279,0.233934298697096,
0.251364575521066,0.263399054117863,0.280262641786752,0.286347380332261),
 .UNSPECIFIED.);
#2407=B_SPLINE_CURVE_WITH_KNOTS('',3,(#27656,#27657,#27658,#27659,#27660,
#27661,#27662,#27663,#27664,#27665,#27666),.UNSPECIFIED.,.F.,.F.,(4,1,1,
1,1,1,1,1,4),(15.7079632679489,15.8014786182354,16.7880079568995,17.7745372955635,
18.7610666342275,19.7475959728915,20.7341253115556,21.7206546502196,21.9911485751285),
 .UNSPECIFIED.);
#2408=B_SPLINE_CURVE_WITH_KNOTS('',3,(#27667,#27668,#27669,#27670,#27671,
#27672,#27673,#27674,#27675,#27676),.UNSPECIFIED.,.F.,.F.,(4,1,1,1,1,1,
1,4),(15.707963267949,16.3714588042999,17.3579881429639,18.344517481628,
19.331046820292,20.317576158956,21.30410549762,21.9911485751285),
 .UNSPECIFIED.);
#2409=B_SPLINE_CURVE_WITH_KNOTS('',3,(#27901,#27902,#27903,#27904,#27905,
#27906,#27907,#27908,#27909,#27910,#27911,#27912,#27913,#27914,#27915,#27916,
#27917,#27918,#27919,#27920,#27921,#27922,#27923,#27924,#27925,#27926,#27927,
#27928,#27929,#27930,#27931,#27932,#27933,#27934,#27935,#27936,#27937,#27938,
#27939,#27940,#27941,#27942,#27943,#27944,#27945,#27946,#27947,#27948,#27949),
 .UNSPECIFIED.,.F.,.F.,(4,3,3,3,3,3,3,3,3,3,3,3,3,3,3,3,4),(0.,0.0274255572386018,
0.0488092947703195,0.0580009970300377,0.0875346963040298,0.101224146180659,
0.111280540172636,0.132431451325231,0.155780482071967,0.165670964883965,
0.19370825904101,0.208717681926172,0.219760935414438,0.239138355867989,
0.257256766122231,0.277820141512143,0.285142803995174),.UNSPECIFIED.);
#2410=B_SPLINE_CURVE_WITH_KNOTS('',3,(#27950,#27951,#27952,#27953,#27954,
#27955,#27956,#27957,#27958,#27959,#27960,#27961,#27962,#27963,#27964,#27965,
#27966,#27967,#27968,#27969,#27970,#27971,#27972,#27973,#27974),
 .UNSPECIFIED.,.F.,.F.,(4,3,3,3,3,3,3,3,4),(-10.1357873115492,-9.8652933866403,
-8.87876404797628,-7.89223470931224,-6.90570537064821,-5.91917603198418,
-4.93264669332015,-3.94611735465612,-3.85260200436966),.UNSPECIFIED.);
#2411=B_SPLINE_CURVE_WITH_KNOTS('',3,(#28199,#28200,#28201,#28202,#28203,
#28204,#28205,#28206,#28207,#28208,#28209,#28210,#28211,#28212,#28213,#28214,
#28215,#28216,#28217,#28218,#28219,#28220,#28221,#28222,#28223),
 .UNSPECIFIED.,.F.,.F.,(4,3,3,3,3,3,3,3,4),(7.5927484481567,7.89223470931225,
8.87876404797628,9.86529338664031,10.8518227253043,11.8383520639684,12.8248814026324,
13.8114107412964,13.8759337553363),.UNSPECIFIED.);
#2412=B_SPLINE_CURVE_WITH_KNOTS('',3,(#28224,#28225,#28226,#28227,#28228,
#28229,#28230,#28231,#28232,#28233,#28234,#28235,#28236,#28237,#28238,#28239,
#28240,#28241,#28242,#28243,#28244,#28245,#28246,#28247,#28248,#28249,#28250,
#28251,#28252,#28253,#28254,#28255,#28256,#28257,#28258,#28259,#28260,#28261,
#28262,#28263,#28264,#28265,#28266,#28267,#28268,#28269,#28270,#28271,#28272,
#28273,#28274,#28275),.UNSPECIFIED.,.F.,.F.,(4,3,3,3,3,3,3,3,3,3,3,3,3,
3,3,3,3,4),(0.,0.0320331739806594,0.047982198208099,0.0587462979950865,
0.0683743220264688,0.0996455083427913,0.112637637236076,0.122453502382791,
0.146764141737189,0.169126654027335,0.178509833663637,0.203948035694404,
0.222826534951851,0.233934300464251,0.251364487179106,0.263399009878289,
0.280262641786705,0.286347380332219),.UNSPECIFIED.);
#2413=B_SPLINE_CURVE_WITH_KNOTS('',3,(#28279,#28280,#28281,#28282,#28283,
#28284,#28285,#28286,#28287,#28288,#28289,#28290,#28291,#28292,#28293,#28294,
#28295,#28296,#28297,#28298,#28299,#28300,#28301,#28302,#28303,#28304,#28305,
#28306,#28307,#28308,#28309,#28310,#28311,#28312,#28313,#28314,#28315,#28316,
#28317,#28318,#28319,#28320,#28321,#28322,#28323,#28324,#28325,#28326,#28327,
#28328,#28329,#28330,#28331,#28332,#28333),.UNSPECIFIED.,.F.,.F.,(4,3,3,
3,3,3,3,3,3,3,3,3,3,3,3,3,3,3,4),(-0.378621596831506,-0.353562246876325,
-0.339726745125034,-0.324795320074381,-0.299965799454646,-0.289116647258409,
-0.252367455997566,-0.234471207960412,-0.219335677585236,-0.200829495678116,
-0.174828907630048,-0.155853084460074,-0.144932199137797,-0.109703302304573,
-0.0896821993996096,-0.0773430052299345,-0.0372184478821882,-0.00401661180490171,
0.),.UNSPECIFIED.);
#2414=B_SPLINE_CURVE_WITH_KNOTS('',3,(#28334,#28335,#28336,#28337,#28338,
#28339,#28340,#28341,#28342,#28343,#28344,#28345,#28346,#28347,#28348,#28349,
#28350,#28351,#28352,#28353,#28354,#28355,#28356,#28357,#28358,#28359,#28360,
#28361,#28362,#28363,#28364,#28365,#28366,#28367,#28368,#28369,#28370,#28371,
#28372,#28373,#28374,#28375,#28376,#28377,#28378,#28379,#28380,#28381,#28382,
#28383,#28384,#28385,#28386,#28387,#28388),.UNSPECIFIED.,.F.,.F.,(4,3,3,
3,3,3,3,3,3,3,3,3,3,3,3,3,3,3,4),(-0.376940817211645,-0.351602392887994,
-0.33251855101009,-0.318227201330527,-0.288328241243131,-0.272716591979397,
-0.234504390923632,-0.216959715082621,-0.205491684554535,-0.180854828870955,
-0.153735831424588,-0.136659504603933,-0.126241092823357,-0.0954984218751326,
-0.0666697806071311,-0.0558640204611096,-0.021970383107796,-0.00327040903045916,
0.),.UNSPECIFIED.);
#2415=B_SPLINE_CURVE_WITH_KNOTS('',3,(#28390,#28391,#28392,#28393,#28394,
#28395,#28396,#28397,#28398,#28399,#28400),.UNSPECIFIED.,.F.,.F.,(4,1,1,
1,1,1,1,1,4),(15.7079632679489,15.8518654961883,16.8494368691713,17.8470082421542,
18.8445796151371,19.8421509881201,20.839722361103,21.837293734086,21.9911485751285),
 .UNSPECIFIED.);
#2416=B_SPLINE_CURVE_WITH_KNOTS('',3,(#28401,#28402,#28403,#28404,#28405,
#28406,#28407,#28408,#28409,#28410),.UNSPECIFIED.,.F.,.F.,(4,1,1,1,1,1,
1,4),(15.7079632679489,16.3932837587427,17.3908551317256,18.3884265047086,
19.3859978776915,20.3835692506744,21.3811406236574,21.9911485751285),
 .UNSPECIFIED.);
#2417=B_SPLINE_CURVE_WITH_KNOTS('',3,(#28755,#28756,#28757,#28758,#28759,
#28760,#28761,#28762,#28763,#28764,#28765,#28766,#28767,#28768,#28769,#28770,
#28771,#28772,#28773,#28774,#28775,#28776,#28777,#28778,#28779,#28780,#28781,
#28782,#28783,#28784,#28785,#28786,#28787,#28788,#28789,#28790,#28791,#28792,
#28793,#28794,#28795,#28796,#28797,#28798,#28799,#28800,#28801,#28802,#28803,
#28804,#28805,#28806),.UNSPECIFIED.,.F.,.F.,(4,3,3,3,3,3,3,3,3,3,3,3,3,
3,3,3,3,4),(0.,0.0336928872610179,0.0587353899469406,0.0734853414895339,
0.10979289593323,0.132866050933898,0.143634155874187,0.177205256270033,
0.19591174232575,0.207613838096411,0.244893860705133,0.269595977941347,
0.282504950871715,0.310154017664246,0.327714110380406,0.342573451622329,
0.372940760482264,0.376940817211574),.UNSPECIFIED.);
#2418=B_SPLINE_CURVE_WITH_KNOTS('',3,(#28807,#28808,#28809,#28810,#28811,
#28812,#28813,#28814,#28815,#28816,#28817,#28818,#28819,#28820,#28821,#28822,
#28823,#28824,#28825,#28826,#28827,#28828,#28829,#28830,#28831),
 .UNSPECIFIED.,.F.,.F.,(4,3,3,3,3,3,3,3,4),(-10.1295685708719,-9.97571372982934,
-8.9781423568464,-7.98057098386347,-6.98299961088054,-5.9854282378976,-4.98785686491467,
-3.99028549193173,-3.84638326369226),.UNSPECIFIED.);
#2419=B_SPLINE_CURVE_WITH_KNOTS('',3,(#29176,#29177,#29178,#29179,#29180,
#29181,#29182,#29183,#29184,#29185,#29186,#29187,#29188,#29189,#29190,#29191,
#29192,#29193,#29194,#29195,#29196,#29197),.UNSPECIFIED.,.F.,.F.,(4,3,3,
3,3,3,3,4),(7.59300756235165,7.98057098386347,8.9781423568464,9.97571372982934,
10.9732851028123,11.9708564757952,12.9684278487781,13.8761928695313),
 .UNSPECIFIED.);
#2420=B_SPLINE_CURVE_WITH_KNOTS('',3,(#29198,#29199,#29200,#29201,#29202,
#29203,#29204,#29205,#29206,#29207,#29208,#29209,#29210,#29211,#29212,#29213,
#29214,#29215,#29216,#29217,#29218,#29219,#29220,#29221,#29222,#29223,#29224,
#29225,#29226,#29227,#29228,#29229,#29230,#29231,#29232,#29233,#29234,#29235,
#29236,#29237,#29238,#29239,#29240,#29241,#29242,#29243,#29244,#29245,#29246,
#29247,#29248,#29249),.UNSPECIFIED.,.F.,.F.,(4,3,3,3,3,3,3,3,3,3,3,3,3,
3,3,3,3,4),(0.,0.0396802077059044,0.0598020944317896,0.0772905411980831,
0.0898519540170797,0.128513068109953,0.153545960121946,0.165105837651985,
0.197163594226428,0.224451618228952,0.234159833899698,0.269454677349509,
0.287586460843776,0.305420009888492,0.333077118982087,0.347224172298259,
0.375339207698941,0.37862159683149),.UNSPECIFIED.);
#3062=LINE('',#24819,#3694);
#3063=LINE('',#24854,#3695);
#3064=LINE('',#24881,#3696);
#3065=LINE('',#24932,#3697);
#3066=LINE('',#24980,#3698);
#3067=LINE('',#25028,#3699);
#3068=LINE('',#25079,#3700);
#3069=LINE('',#25127,#3701);
#3070=LINE('',#25175,#3702);
#3071=LINE('',#25226,#3703);
#3072=LINE('',#25277,#3704);
#3073=LINE('',#25325,#3705);
#3074=LINE('',#25376,#3706);
#3075=LINE('',#25415,#3707);
#3076=LINE('',#25437,#3708);
#3077=LINE('',#25461,#3709);
#3078=LINE('',#25486,#3710);
#3079=LINE('',#25511,#3711);
#3080=LINE('',#25535,#3712);
#3081=LINE('',#25560,#3713);
#3082=LINE('',#25584,#3714);
#3083=LINE('',#25609,#3715);
#3084=LINE('',#25633,#3716);
#3085=LINE('',#25658,#3717);
#3086=LINE('',#25683,#3718);
#3087=LINE('',#25707,#3719);
#3088=LINE('',#25724,#3720);
#3089=LINE('',#25745,#3721);
#3090=LINE('',#25796,#3722);
#3091=LINE('',#25847,#3723);
#3092=LINE('',#25895,#3724);
#3093=LINE('',#25946,#3725);
#3094=LINE('',#25997,#3726);
#3095=LINE('',#26045,#3727);
#3096=LINE('',#26084,#3728);
#3097=LINE('',#26105,#3729);
#3098=LINE('',#26156,#3730);
#3099=LINE('',#26207,#3731);
#3100=LINE('',#26255,#3732);
#3101=LINE('',#26306,#3733);
#3102=LINE('',#26357,#3734);
#3103=LINE('',#26405,#3735);
#3104=LINE('',#26444,#3736);
#3105=LINE('',#26468,#3737);
#3106=LINE('',#26492,#3738);
#3107=LINE('',#26517,#3739);
#3108=LINE('',#26542,#3740);
#3109=LINE('',#26566,#3741);
#3110=LINE('',#26591,#3742);
#3111=LINE('',#26616,#3743);
#3112=LINE('',#26633,#3744);
#3113=LINE('',#26657,#3745);
#3114=LINE('',#26681,#3746);
#3115=LINE('',#26706,#3747);
#3116=LINE('',#26731,#3748);
#3117=LINE('',#26755,#3749);
#3118=LINE('',#26780,#3750);
#3119=LINE('',#26805,#3751);
#3120=LINE('',#27546,#3752);
#3121=LINE('',#27548,#3753);
#3122=LINE('',#27550,#3754);
#3123=LINE('',#27552,#3755);
#3124=LINE('',#27553,#3756);
#3125=LINE('',#29260,#3757);
#3126=LINE('',#29268,#3758);
#3127=LINE('',#29281,#3759);
#3128=LINE('',#29283,#3760);
#3129=LINE('',#29286,#3761);
#3130=LINE('',#29288,#3762);
#3131=LINE('',#29289,#3763);
#3132=LINE('',#29292,#3764);
#3133=LINE('',#29294,#3765);
#3134=LINE('',#29295,#3766);
#3135=LINE('',#29297,#3767);
#3136=LINE('',#29300,#3768);
#3137=LINE('',#29302,#3769);
#3138=LINE('',#29303,#3770);
#3139=LINE('',#29305,#3771);
#3140=LINE('',#29311,#3772);
#3694=VECTOR('',#13111,0.2);
#3695=VECTOR('',#13114,0.2);
#3696=VECTOR('',#13119,0.2);
#3697=VECTOR('',#13122,0.2);
#3698=VECTOR('',#13125,0.2);
#3699=VECTOR('',#13128,0.2);
#3700=VECTOR('',#13131,0.2);
#3701=VECTOR('',#13134,0.2);
#3702=VECTOR('',#13137,0.2);
#3703=VECTOR('',#13140,0.2);
#3704=VECTOR('',#13143,0.2);
#3705=VECTOR('',#13146,0.2);
#3706=VECTOR('',#13149,0.2);
#3707=VECTOR('',#13154,0.205475);
#3708=VECTOR('',#13159,0.205475);
#3709=VECTOR('',#13162,0.205475);
#3710=VECTOR('',#13165,0.205475);
#3711=VECTOR('',#13168,0.205475);
#3712=VECTOR('',#13171,0.205475);
#3713=VECTOR('',#13174,0.205475);
#3714=VECTOR('',#13177,0.205475);
#3715=VECTOR('',#13180,0.205475);
#3716=VECTOR('',#13183,0.205475);
#3717=VECTOR('',#13186,0.205475);
#3718=VECTOR('',#13189,0.205475);
#3719=VECTOR('',#13192,0.205475);
#3720=VECTOR('',#13197,0.15);
#3721=VECTOR('',#13202,0.15);
#3722=VECTOR('',#13205,0.15);
#3723=VECTOR('',#13208,0.15);
#3724=VECTOR('',#13211,0.15);
#3725=VECTOR('',#13214,0.15);
#3726=VECTOR('',#13217,0.15);
#3727=VECTOR('',#13220,0.15);
#3728=VECTOR('',#13225,0.15);
#3729=VECTOR('',#13230,0.15);
#3730=VECTOR('',#13233,0.15);
#3731=VECTOR('',#13236,0.15);
#3732=VECTOR('',#13239,0.15);
#3733=VECTOR('',#13242,0.15);
#3734=VECTOR('',#13245,0.15);
#3735=VECTOR('',#13248,0.15);
#3736=VECTOR('',#13253,0.1543);
#3737=VECTOR('',#13258,0.1543);
#3738=VECTOR('',#13261,0.1543);
#3739=VECTOR('',#13264,0.1543);
#3740=VECTOR('',#13267,0.1543);
#3741=VECTOR('',#13270,0.1543);
#3742=VECTOR('',#13273,0.1543);
#3743=VECTOR('',#13276,0.1543);
#3744=VECTOR('',#13281,0.1543);
#3745=VECTOR('',#13286,0.1543);
#3746=VECTOR('',#13289,0.1543);
#3747=VECTOR('',#13292,0.1543);
#3748=VECTOR('',#13295,0.1543);
#3749=VECTOR('',#13298,0.1543);
#3750=VECTOR('',#13301,0.1543);
#3751=VECTOR('',#13304,0.1543);
#3752=VECTOR('',#13313,1.);
#3753=VECTOR('',#13314,1.);
#3754=VECTOR('',#13315,1.);
#3755=VECTOR('',#13316,1.);
#3756=VECTOR('',#13317,1.);
#3757=VECTOR('',#13342,0.6);
#3758=VECTOR('',#13353,0.6);
#3759=VECTOR('',#13370,1.);
#3760=VECTOR('',#13373,0.6);
#3761=VECTOR('',#13376,1.);
#3762=VECTOR('',#13377,1.);
#3763=VECTOR('',#13378,1.);
#3764=VECTOR('',#13381,1.);
#3765=VECTOR('',#13382,1.);
#3766=VECTOR('',#13383,1.);
#3767=VECTOR('',#13386,1.);
#3768=VECTOR('',#13389,1.);
#3769=VECTOR('',#13390,1.);
#3770=VECTOR('',#13391,1.);
#3771=VECTOR('',#13394,1.);
#3772=VECTOR('',#13403,0.6);
#4500=VERTEX_POINT('',#24817);
#4501=VERTEX_POINT('',#24818);
#4502=VERTEX_POINT('',#24820);
#4503=VERTEX_POINT('',#24843);
#4504=VERTEX_POINT('',#24845);
#4505=VERTEX_POINT('',#24853);
#4506=VERTEX_POINT('',#24879);
#4507=VERTEX_POINT('',#24880);
#4508=VERTEX_POINT('',#24930);
#4509=VERTEX_POINT('',#24931);
#4510=VERTEX_POINT('',#24978);
#4511=VERTEX_POINT('',#24979);
#4512=VERTEX_POINT('',#25026);
#4513=VERTEX_POINT('',#25027);
#4514=VERTEX_POINT('',#25077);
#4515=VERTEX_POINT('',#25078);
#4516=VERTEX_POINT('',#25125);
#4517=VERTEX_POINT('',#25126);
#4518=VERTEX_POINT('',#25173);
#4519=VERTEX_POINT('',#25174);
#4520=VERTEX_POINT('',#25224);
#4521=VERTEX_POINT('',#25225);
#4522=VERTEX_POINT('',#25275);
#4523=VERTEX_POINT('',#25276);
#4524=VERTEX_POINT('',#25323);
#4525=VERTEX_POINT('',#25324);
#4526=VERTEX_POINT('',#25374);
#4527=VERTEX_POINT('',#25375);
#4528=VERTEX_POINT('',#25377);
#4529=VERTEX_POINT('',#25391);
#4530=VERTEX_POINT('',#25413);
#4531=VERTEX_POINT('',#25414);
#4532=VERTEX_POINT('',#25416);
#4533=VERTEX_POINT('',#25424);
#4534=VERTEX_POINT('',#25435);
#4535=VERTEX_POINT('',#25436);
#4536=VERTEX_POINT('',#25459);
#4537=VERTEX_POINT('',#25460);
#4538=VERTEX_POINT('',#25484);
#4539=VERTEX_POINT('',#25485);
#4540=VERTEX_POINT('',#25509);
#4541=VERTEX_POINT('',#25510);
#4542=VERTEX_POINT('',#25533);
#4543=VERTEX_POINT('',#25534);
#4544=VERTEX_POINT('',#25558);
#4545=VERTEX_POINT('',#25559);
#4546=VERTEX_POINT('',#25582);
#4547=VERTEX_POINT('',#25583);
#4548=VERTEX_POINT('',#25607);
#4549=VERTEX_POINT('',#25608);
#4550=VERTEX_POINT('',#25631);
#4551=VERTEX_POINT('',#25632);
#4552=VERTEX_POINT('',#25656);
#4553=VERTEX_POINT('',#25657);
#4554=VERTEX_POINT('',#25681);
#4555=VERTEX_POINT('',#25682);
#4556=VERTEX_POINT('',#25705);
#4557=VERTEX_POINT('',#25706);
#4558=VERTEX_POINT('',#25708);
#4559=VERTEX_POINT('',#25714);
#4560=VERTEX_POINT('',#25722);
#4561=VERTEX_POINT('',#25723);
#4562=VERTEX_POINT('',#25725);
#4563=VERTEX_POINT('',#25730);
#4564=VERTEX_POINT('',#25743);
#4565=VERTEX_POINT('',#25744);
#4566=VERTEX_POINT('',#25794);
#4567=VERTEX_POINT('',#25795);
#4568=VERTEX_POINT('',#25845);
#4569=VERTEX_POINT('',#25846);
#4570=VERTEX_POINT('',#25893);
#4571=VERTEX_POINT('',#25894);
#4572=VERTEX_POINT('',#25944);
#4573=VERTEX_POINT('',#25945);
#4574=VERTEX_POINT('',#25995);
#4575=VERTEX_POINT('',#25996);
#4576=VERTEX_POINT('',#26043);
#4577=VERTEX_POINT('',#26044);
#4578=VERTEX_POINT('',#26046);
#4579=VERTEX_POINT('',#26060);
#4580=VERTEX_POINT('',#26082);
#4581=VERTEX_POINT('',#26083);
#4582=VERTEX_POINT('',#26085);
#4583=VERTEX_POINT('',#26090);
#4584=VERTEX_POINT('',#26103);
#4585=VERTEX_POINT('',#26104);
#4586=VERTEX_POINT('',#26154);
#4587=VERTEX_POINT('',#26155);
#4588=VERTEX_POINT('',#26205);
#4589=VERTEX_POINT('',#26206);
#4590=VERTEX_POINT('',#26253);
#4591=VERTEX_POINT('',#26254);
#4592=VERTEX_POINT('',#26304);
#4593=VERTEX_POINT('',#26305);
#4594=VERTEX_POINT('',#26355);
#4595=VERTEX_POINT('',#26356);
#4596=VERTEX_POINT('',#26403);
#4597=VERTEX_POINT('',#26404);
#4598=VERTEX_POINT('',#26406);
#4599=VERTEX_POINT('',#26420);
#4600=VERTEX_POINT('',#26442);
#4601=VERTEX_POINT('',#26443);
#4602=VERTEX_POINT('',#26445);
#4603=VERTEX_POINT('',#26454);
#4604=VERTEX_POINT('',#26466);
#4605=VERTEX_POINT('',#26467);
#4606=VERTEX_POINT('',#26490);
#4607=VERTEX_POINT('',#26491);
#4608=VERTEX_POINT('',#26515);
#4609=VERTEX_POINT('',#26516);
#4610=VERTEX_POINT('',#26540);
#4611=VERTEX_POINT('',#26541);
#4612=VERTEX_POINT('',#26564);
#4613=VERTEX_POINT('',#26565);
#4614=VERTEX_POINT('',#26589);
#4615=VERTEX_POINT('',#26590);
#4616=VERTEX_POINT('',#26614);
#4617=VERTEX_POINT('',#26615);
#4618=VERTEX_POINT('',#26617);
#4619=VERTEX_POINT('',#26623);
#4620=VERTEX_POINT('',#26631);
#4621=VERTEX_POINT('',#26632);
#4622=VERTEX_POINT('',#26634);
#4623=VERTEX_POINT('',#26643);
#4624=VERTEX_POINT('',#26655);
#4625=VERTEX_POINT('',#26656);
#4626=VERTEX_POINT('',#26679);
#4627=VERTEX_POINT('',#26680);
#4628=VERTEX_POINT('',#26704);
#4629=VERTEX_POINT('',#26705);
#4630=VERTEX_POINT('',#26729);
#4631=VERTEX_POINT('',#26730);
#4632=VERTEX_POINT('',#26753);
#4633=VERTEX_POINT('',#26754);
#4634=VERTEX_POINT('',#26778);
#4635=VERTEX_POINT('',#26779);
#4636=VERTEX_POINT('',#26803);
#4637=VERTEX_POINT('',#26804);
#4638=VERTEX_POINT('',#26806);
#4639=VERTEX_POINT('',#26812);
#4640=VERTEX_POINT('',#27542);
#4641=VERTEX_POINT('',#27543);
#4642=VERTEX_POINT('',#27545);
#4643=VERTEX_POINT('',#27547);
#4644=VERTEX_POINT('',#27549);
#4645=VERTEX_POINT('',#27551);
#4646=VERTEX_POINT('',#29253);
#4647=VERTEX_POINT('',#29255);
#4648=VERTEX_POINT('',#29259);
#4649=VERTEX_POINT('',#29263);
#4650=VERTEX_POINT('',#29267);
#4651=VERTEX_POINT('',#29271);
#4652=VERTEX_POINT('',#29273);
#4653=VERTEX_POINT('',#29276);
#4654=VERTEX_POINT('',#29278);
#4655=VERTEX_POINT('',#29285);
#4656=VERTEX_POINT('',#29287);
#4657=VERTEX_POINT('',#29291);
#4658=VERTEX_POINT('',#29293);
#4659=VERTEX_POINT('',#29299);
#4660=VERTEX_POINT('',#29301);
#4661=VERTEX_POINT('',#29309);
#5810=EDGE_CURVE('',#4500,#4501,#3062,.T.);
#5811=EDGE_CURVE('',#4501,#4502,#2282,.T.);
#5812=EDGE_CURVE('',#4502,#4503,#1889,.T.);
#5813=EDGE_CURVE('',#4503,#4504,#2283,.T.);
#5814=EDGE_CURVE('',#4504,#4505,#3063,.T.);
#5815=EDGE_CURVE('',#4505,#4505,#1890,.F.);
#5816=EDGE_CURVE('',#4504,#4500,#2284,.T.);
#5817=EDGE_CURVE('',#4506,#4507,#3064,.T.);
#5818=EDGE_CURVE('',#4507,#4501,#2285,.T.);
#5819=EDGE_CURVE('',#4500,#4506,#2286,.T.);
#5820=EDGE_CURVE('',#4508,#4509,#3065,.T.);
#5821=EDGE_CURVE('',#4509,#4507,#2287,.T.);
#5822=EDGE_CURVE('',#4506,#4508,#2288,.T.);
#5823=EDGE_CURVE('',#4510,#4511,#3066,.T.);
#5824=EDGE_CURVE('',#4511,#4509,#2289,.T.);
#5825=EDGE_CURVE('',#4508,#4510,#2290,.T.);
#5826=EDGE_CURVE('',#4512,#4513,#3067,.T.);
#5827=EDGE_CURVE('',#4513,#4511,#2291,.T.);
#5828=EDGE_CURVE('',#4510,#4512,#2292,.T.);
#5829=EDGE_CURVE('',#4514,#4515,#3068,.T.);
#5830=EDGE_CURVE('',#4515,#4513,#2293,.T.);
#5831=EDGE_CURVE('',#4512,#4514,#2294,.T.);
#5832=EDGE_CURVE('',#4516,#4517,#3069,.T.);
#5833=EDGE_CURVE('',#4517,#4515,#2295,.T.);
#5834=EDGE_CURVE('',#4514,#4516,#2296,.T.);
#5835=EDGE_CURVE('',#4518,#4519,#3070,.T.);
#5836=EDGE_CURVE('',#4519,#4517,#2297,.T.);
#5837=EDGE_CURVE('',#4516,#4518,#2298,.T.);
#5838=EDGE_CURVE('',#4520,#4521,#3071,.T.);
#5839=EDGE_CURVE('',#4521,#4519,#2299,.T.);
#5840=EDGE_CURVE('',#4518,#4520,#2300,.T.);
#5841=EDGE_CURVE('',#4522,#4523,#3072,.T.);
#5842=EDGE_CURVE('',#4523,#4521,#2301,.T.);
#5843=EDGE_CURVE('',#4520,#4522,#2302,.T.);
#5844=EDGE_CURVE('',#4524,#4525,#3073,.T.);
#5845=EDGE_CURVE('',#4525,#4523,#2303,.T.);
#5846=EDGE_CURVE('',#4522,#4524,#2304,.T.);
#5847=EDGE_CURVE('',#4526,#4527,#3074,.T.);
#5848=EDGE_CURVE('',#4526,#4528,#2305,.T.);
#5849=EDGE_CURVE('',#4529,#4528,#1891,.T.);
#5850=EDGE_CURVE('',#4529,#4527,#2306,.T.);
#5851=EDGE_CURVE('',#4530,#4531,#3075,.T.);
#5852=EDGE_CURVE('',#4531,#4532,#2307,.T.);
#5853=EDGE_CURVE('',#4533,#4532,#1892,.T.);
#5854=EDGE_CURVE('',#4530,#4533,#2308,.T.);
#5855=EDGE_CURVE('',#4534,#4535,#3076,.T.);
#5856=EDGE_CURVE('',#4535,#4531,#2309,.T.);
#5857=EDGE_CURVE('',#4534,#4530,#2310,.T.);
#5858=EDGE_CURVE('',#4536,#4537,#3077,.T.);
#5859=EDGE_CURVE('',#4537,#4535,#2311,.T.);
#5860=EDGE_CURVE('',#4536,#4534,#2312,.T.);
#5861=EDGE_CURVE('',#4538,#4539,#3078,.T.);
#5862=EDGE_CURVE('',#4539,#4537,#2313,.T.);
#5863=EDGE_CURVE('',#4538,#4536,#2314,.T.);
#5864=EDGE_CURVE('',#4540,#4541,#3079,.T.);
#5865=EDGE_CURVE('',#4541,#4539,#2315,.T.);
#5866=EDGE_CURVE('',#4540,#4538,#2316,.T.);
#5867=EDGE_CURVE('',#4542,#4543,#3080,.T.);
#5868=EDGE_CURVE('',#4543,#4541,#2317,.T.);
#5869=EDGE_CURVE('',#4542,#4540,#2318,.T.);
#5870=EDGE_CURVE('',#4544,#4545,#3081,.T.);
#5871=EDGE_CURVE('',#4545,#4543,#2319,.T.);
#5872=EDGE_CURVE('',#4544,#4542,#2320,.T.);
#5873=EDGE_CURVE('',#4546,#4547,#3082,.T.);
#5874=EDGE_CURVE('',#4547,#4545,#2321,.T.);
#5875=EDGE_CURVE('',#4546,#4544,#2322,.T.);
#5876=EDGE_CURVE('',#4548,#4549,#3083,.T.);
#5877=EDGE_CURVE('',#4549,#4547,#2323,.T.);
#5878=EDGE_CURVE('',#4548,#4546,#2324,.T.);
#5879=EDGE_CURVE('',#4550,#4551,#3084,.T.);
#5880=EDGE_CURVE('',#4551,#4549,#2325,.T.);
#5881=EDGE_CURVE('',#4550,#4548,#2326,.T.);
#5882=EDGE_CURVE('',#4552,#4553,#3085,.T.);
#5883=EDGE_CURVE('',#4553,#4551,#2327,.T.);
#5884=EDGE_CURVE('',#4552,#4550,#2328,.T.);
#5885=EDGE_CURVE('',#4554,#4555,#3086,.T.);
#5886=EDGE_CURVE('',#4555,#4553,#2329,.T.);
#5887=EDGE_CURVE('',#4554,#4552,#2330,.T.);
#5888=EDGE_CURVE('',#4556,#4557,#3087,.T.);
#5889=EDGE_CURVE('',#4558,#4556,#2331,.T.);
#5890=EDGE_CURVE('',#4559,#4558,#1893,.T.);
#5891=EDGE_CURVE('',#4559,#4557,#2332,.T.);
#5892=EDGE_CURVE('',#4560,#4561,#3088,.T.);
#5893=EDGE_CURVE('',#4561,#4562,#2333,.T.);
#5894=EDGE_CURVE('',#4563,#4562,#1894,.F.);
#5895=EDGE_CURVE('',#4563,#4560,#2334,.T.);
#5896=EDGE_CURVE('',#4564,#4565,#3089,.T.);
#5897=EDGE_CURVE('',#4565,#4561,#2335,.T.);
#5898=EDGE_CURVE('',#4560,#4564,#2336,.T.);
#5899=EDGE_CURVE('',#4566,#4567,#3090,.T.);
#5900=EDGE_CURVE('',#4567,#4565,#2337,.T.);
#5901=EDGE_CURVE('',#4564,#4566,#2338,.T.);
#5902=EDGE_CURVE('',#4568,#4569,#3091,.T.);
#5903=EDGE_CURVE('',#4569,#4567,#2339,.T.);
#5904=EDGE_CURVE('',#4566,#4568,#2340,.T.);
#5905=EDGE_CURVE('',#4570,#4571,#3092,.T.);
#5906=EDGE_CURVE('',#4571,#4569,#2341,.T.);
#5907=EDGE_CURVE('',#4568,#4570,#2342,.T.);
#5908=EDGE_CURVE('',#4572,#4573,#3093,.T.);
#5909=EDGE_CURVE('',#4573,#4571,#2343,.T.);
#5910=EDGE_CURVE('',#4570,#4572,#2344,.T.);
#5911=EDGE_CURVE('',#4574,#4575,#3094,.T.);
#5912=EDGE_CURVE('',#4575,#4573,#2345,.T.);
#5913=EDGE_CURVE('',#4572,#4574,#2346,.T.);
#5914=EDGE_CURVE('',#4576,#4577,#3095,.T.);
#5915=EDGE_CURVE('',#4576,#4578,#2347,.T.);
#5916=EDGE_CURVE('',#4579,#4578,#1895,.T.);
#5917=EDGE_CURVE('',#4579,#4577,#2348,.T.);
#5918=EDGE_CURVE('',#4580,#4581,#3096,.T.);
#5919=EDGE_CURVE('',#4581,#4582,#2349,.T.);
#5920=EDGE_CURVE('',#4583,#4582,#1896,.F.);
#5921=EDGE_CURVE('',#4583,#4580,#2350,.T.);
#5922=EDGE_CURVE('',#4584,#4585,#3097,.T.);
#5923=EDGE_CURVE('',#4585,#4581,#2351,.T.);
#5924=EDGE_CURVE('',#4580,#4584,#2352,.T.);
#5925=EDGE_CURVE('',#4586,#4587,#3098,.T.);
#5926=EDGE_CURVE('',#4587,#4585,#2353,.T.);
#5927=EDGE_CURVE('',#4584,#4586,#2354,.T.);
#5928=EDGE_CURVE('',#4588,#4589,#3099,.T.);
#5929=EDGE_CURVE('',#4589,#4587,#2355,.T.);
#5930=EDGE_CURVE('',#4586,#4588,#2356,.T.);
#5931=EDGE_CURVE('',#4590,#4591,#3100,.T.);
#5932=EDGE_CURVE('',#4591,#4589,#2357,.T.);
#5933=EDGE_CURVE('',#4588,#4590,#2358,.T.);
#5934=EDGE_CURVE('',#4592,#4593,#3101,.T.);
#5935=EDGE_CURVE('',#4593,#4591,#2359,.T.);
#5936=EDGE_CURVE('',#4590,#4592,#2360,.T.);
#5937=EDGE_CURVE('',#4594,#4595,#3102,.T.);
#5938=EDGE_CURVE('',#4595,#4593,#2361,.T.);
#5939=EDGE_CURVE('',#4592,#4594,#2362,.T.);
#5940=EDGE_CURVE('',#4596,#4597,#3103,.T.);
#5941=EDGE_CURVE('',#4596,#4598,#2363,.T.);
#5942=EDGE_CURVE('',#4599,#4598,#1897,.T.);
#5943=EDGE_CURVE('',#4599,#4597,#2364,.T.);
#5944=EDGE_CURVE('',#4600,#4601,#3104,.T.);
#5945=EDGE_CURVE('',#4601,#4602,#2365,.T.);
#5946=EDGE_CURVE('',#4603,#4602,#1898,.T.);
#5947=EDGE_CURVE('',#4600,#4603,#2366,.T.);
#5948=EDGE_CURVE('',#4604,#4605,#3105,.T.);
#5949=EDGE_CURVE('',#4605,#4601,#2367,.T.);
#5950=EDGE_CURVE('',#4604,#4600,#2368,.T.);
#5951=EDGE_CURVE('',#4606,#4607,#3106,.T.);
#5952=EDGE_CURVE('',#4607,#4605,#2369,.T.);
#5953=EDGE_CURVE('',#4606,#4604,#2370,.T.);
#5954=EDGE_CURVE('',#4608,#4609,#3107,.T.);
#5955=EDGE_CURVE('',#4609,#4607,#2371,.T.);
#5956=EDGE_CURVE('',#4608,#4606,#2372,.T.);
#5957=EDGE_CURVE('',#4610,#4611,#3108,.T.);
#5958=EDGE_CURVE('',#4611,#4609,#2373,.T.);
#5959=EDGE_CURVE('',#4610,#4608,#2374,.T.);
#5960=EDGE_CURVE('',#4612,#4613,#3109,.T.);
#5961=EDGE_CURVE('',#4613,#4611,#2375,.T.);
#5962=EDGE_CURVE('',#4612,#4610,#2376,.T.);
#5963=EDGE_CURVE('',#4614,#4615,#3110,.T.);
#5964=EDGE_CURVE('',#4615,#4613,#2377,.T.);
#5965=EDGE_CURVE('',#4614,#4612,#2378,.T.);
#5966=EDGE_CURVE('',#4616,#4617,#3111,.T.);
#5967=EDGE_CURVE('',#4618,#4616,#2379,.T.);
#5968=EDGE_CURVE('',#4619,#4618,#1899,.T.);
#5969=EDGE_CURVE('',#4619,#4617,#2380,.T.);
#5970=EDGE_CURVE('',#4620,#4621,#3112,.T.);
#5971=EDGE_CURVE('',#4621,#4622,#2381,.T.);
#5972=EDGE_CURVE('',#4623,#4622,#1900,.T.);
#5973=EDGE_CURVE('',#4620,#4623,#2382,.T.);
#5974=EDGE_CURVE('',#4624,#4625,#3113,.T.);
#5975=EDGE_CURVE('',#4625,#4621,#2383,.T.);
#5976=EDGE_CURVE('',#4624,#4620,#2384,.T.);
#5977=EDGE_CURVE('',#4626,#4627,#3114,.T.);
#5978=EDGE_CURVE('',#4627,#4625,#2385,.T.);
#5979=EDGE_CURVE('',#4626,#4624,#2386,.T.);
#5980=EDGE_CURVE('',#4628,#4629,#3115,.T.);
#5981=EDGE_CURVE('',#4629,#4627,#2387,.T.);
#5982=EDGE_CURVE('',#4628,#4626,#2388,.T.);
#5983=EDGE_CURVE('',#4630,#4631,#3116,.T.);
#5984=EDGE_CURVE('',#4631,#4629,#2389,.T.);
#5985=EDGE_CURVE('',#4630,#4628,#2390,.T.);
#5986=EDGE_CURVE('',#4632,#4633,#3117,.T.);
#5987=EDGE_CURVE('',#4633,#4631,#2391,.T.);
#5988=EDGE_CURVE('',#4632,#4630,#2392,.T.);
#5989=EDGE_CURVE('',#4634,#4635,#3118,.T.);
#5990=EDGE_CURVE('',#4635,#4633,#2393,.T.);
#5991=EDGE_CURVE('',#4634,#4632,#2394,.T.);
#5992=EDGE_CURVE('',#4636,#4637,#3119,.T.);
#5993=EDGE_CURVE('',#4638,#4636,#2395,.T.);
#5994=EDGE_CURVE('',#4639,#4638,#1901,.T.);
#5995=EDGE_CURVE('',#4639,#4637,#2396,.T.);
#5996=EDGE_CURVE('',#4637,#4635,#2397,.T.);
#5997=EDGE_CURVE('',#4636,#4634,#2398,.T.);
#5998=EDGE_CURVE('',#4622,#4583,#2399,.T.);
#5999=EDGE_CURVE('',#4598,#4639,#2400,.T.);
#6000=EDGE_CURVE('',#4594,#4596,#2401,.T.);
#6001=EDGE_CURVE('',#4582,#4623,#2402,.T.);
#6002=EDGE_CURVE('',#4597,#4595,#2403,.T.);
#6003=EDGE_CURVE('',#4638,#4599,#2404,.T.);
#6004=EDGE_CURVE('',#4640,#4641,#1902,.T.);
#6005=EDGE_CURVE('',#4642,#4640,#3120,.T.);
#6006=EDGE_CURVE('',#4643,#4642,#3121,.T.);
#6007=EDGE_CURVE('',#4644,#4643,#3122,.T.);
#6008=EDGE_CURVE('',#4645,#4644,#3123,.T.);
#6009=EDGE_CURVE('',#4641,#4645,#3124,.T.);
#6010=EDGE_CURVE('',#4562,#4603,#2405,.T.);
#6011=EDGE_CURVE('',#4602,#4563,#2406,.T.);
#6012=EDGE_CURVE('',#4617,#4615,#2407,.T.);
#6013=EDGE_CURVE('',#4616,#4614,#2408,.T.);
#6014=EDGE_CURVE('',#4578,#4619,#2409,.T.);
#6015=EDGE_CURVE('',#4574,#4576,#2410,.T.);
#6016=EDGE_CURVE('',#4577,#4575,#2411,.T.);
#6017=EDGE_CURVE('',#4618,#4579,#2412,.T.);
#6018=EDGE_CURVE('',#4502,#4533,#2413,.T.);
#6019=EDGE_CURVE('',#4532,#4503,#2414,.T.);
#6020=EDGE_CURVE('',#4557,#4555,#2415,.T.);
#6021=EDGE_CURVE('',#4556,#4554,#2416,.T.);
#6022=EDGE_CURVE('',#4528,#4559,#2417,.T.);
#6023=EDGE_CURVE('',#4524,#4526,#2418,.T.);
#6024=EDGE_CURVE('',#4527,#4525,#2419,.T.);
#6025=EDGE_CURVE('',#4558,#4529,#2420,.T.);
#6026=EDGE_CURVE('',#4646,#4646,#1903,.T.);
#6027=EDGE_CURVE('',#4646,#4647,#1904,.T.);
#6028=EDGE_CURVE('',#4647,#4647,#1905,.T.);
#6029=EDGE_CURVE('',#4647,#4648,#3125,.T.);
#6030=EDGE_CURVE('',#4648,#4648,#1906,.T.);
#6031=EDGE_CURVE('',#4648,#4649,#1907,.T.);
#6032=EDGE_CURVE('',#4649,#4649,#1908,.T.);
#6033=EDGE_CURVE('',#4649,#4650,#3126,.T.);
#6034=EDGE_CURVE('',#4650,#4650,#1909,.T.);
#6035=EDGE_CURVE('',#4651,#4651,#1910,.T.);
#6036=EDGE_CURVE('',#4652,#4652,#1911,.T.);
#6037=EDGE_CURVE('',#4653,#4653,#1912,.T.);
#6038=EDGE_CURVE('',#4654,#4654,#1913,.T.);
#6039=EDGE_CURVE('',#4651,#4653,#3127,.T.);
#6040=EDGE_CURVE('',#4654,#4646,#3128,.T.);
#6041=EDGE_CURVE('',#4641,#4655,#3129,.T.);
#6042=EDGE_CURVE('',#4645,#4656,#3130,.T.);
#6043=EDGE_CURVE('',#4655,#4656,#3131,.T.);
#6044=EDGE_CURVE('',#4643,#4657,#3132,.T.);
#6045=EDGE_CURVE('',#4658,#4657,#3133,.T.);
#6046=EDGE_CURVE('',#4644,#4658,#3134,.T.);
#6047=EDGE_CURVE('',#4656,#4658,#3135,.T.);
#6048=EDGE_CURVE('',#4659,#4640,#3136,.T.);
#6049=EDGE_CURVE('',#4660,#4659,#3137,.T.);
#6050=EDGE_CURVE('',#4642,#4660,#3138,.T.);
#6051=EDGE_CURVE('',#4657,#4660,#3139,.T.);
#6052=EDGE_CURVE('',#4659,#4655,#1914,.T.);
#6053=EDGE_CURVE('',#4661,#4661,#1915,.T.);
#6054=EDGE_CURVE('',#4661,#4652,#3140,.T.);
#8081=ORIENTED_EDGE('',*,*,#5810,.T.);
#8082=ORIENTED_EDGE('',*,*,#5811,.T.);
#8083=ORIENTED_EDGE('',*,*,#5812,.T.);
#8084=ORIENTED_EDGE('',*,*,#5813,.T.);
#8085=ORIENTED_EDGE('',*,*,#5814,.T.);
#8086=ORIENTED_EDGE('',*,*,#5815,.T.);
#8087=ORIENTED_EDGE('',*,*,#5814,.F.);
#8088=ORIENTED_EDGE('',*,*,#5816,.T.);
#8089=ORIENTED_EDGE('',*,*,#5817,.T.);
#8090=ORIENTED_EDGE('',*,*,#5818,.T.);
#8091=ORIENTED_EDGE('',*,*,#5810,.F.);
#8092=ORIENTED_EDGE('',*,*,#5819,.T.);
#8093=ORIENTED_EDGE('',*,*,#5820,.T.);
#8094=ORIENTED_EDGE('',*,*,#5821,.T.);
#8095=ORIENTED_EDGE('',*,*,#5817,.F.);
#8096=ORIENTED_EDGE('',*,*,#5822,.T.);
#8097=ORIENTED_EDGE('',*,*,#5823,.T.);
#8098=ORIENTED_EDGE('',*,*,#5824,.T.);
#8099=ORIENTED_EDGE('',*,*,#5820,.F.);
#8100=ORIENTED_EDGE('',*,*,#5825,.T.);
#8101=ORIENTED_EDGE('',*,*,#5826,.T.);
#8102=ORIENTED_EDGE('',*,*,#5827,.T.);
#8103=ORIENTED_EDGE('',*,*,#5823,.F.);
#8104=ORIENTED_EDGE('',*,*,#5828,.T.);
#8105=ORIENTED_EDGE('',*,*,#5829,.T.);
#8106=ORIENTED_EDGE('',*,*,#5830,.T.);
#8107=ORIENTED_EDGE('',*,*,#5826,.F.);
#8108=ORIENTED_EDGE('',*,*,#5831,.T.);
#8109=ORIENTED_EDGE('',*,*,#5832,.T.);
#8110=ORIENTED_EDGE('',*,*,#5833,.T.);
#8111=ORIENTED_EDGE('',*,*,#5829,.F.);
#8112=ORIENTED_EDGE('',*,*,#5834,.T.);
#8113=ORIENTED_EDGE('',*,*,#5835,.T.);
#8114=ORIENTED_EDGE('',*,*,#5836,.T.);
#8115=ORIENTED_EDGE('',*,*,#5832,.F.);
#8116=ORIENTED_EDGE('',*,*,#5837,.T.);
#8117=ORIENTED_EDGE('',*,*,#5838,.T.);
#8118=ORIENTED_EDGE('',*,*,#5839,.T.);
#8119=ORIENTED_EDGE('',*,*,#5835,.F.);
#8120=ORIENTED_EDGE('',*,*,#5840,.T.);
#8121=ORIENTED_EDGE('',*,*,#5841,.T.);
#8122=ORIENTED_EDGE('',*,*,#5842,.T.);
#8123=ORIENTED_EDGE('',*,*,#5838,.F.);
#8124=ORIENTED_EDGE('',*,*,#5843,.T.);
#8125=ORIENTED_EDGE('',*,*,#5844,.T.);
#8126=ORIENTED_EDGE('',*,*,#5845,.T.);
#8127=ORIENTED_EDGE('',*,*,#5841,.F.);
#8128=ORIENTED_EDGE('',*,*,#5846,.T.);
#8129=ORIENTED_EDGE('',*,*,#5847,.F.);
#8130=ORIENTED_EDGE('',*,*,#5848,.T.);
#8131=ORIENTED_EDGE('',*,*,#5849,.F.);
#8132=ORIENTED_EDGE('',*,*,#5850,.T.);
#8133=ORIENTED_EDGE('',*,*,#5851,.T.);
#8134=ORIENTED_EDGE('',*,*,#5852,.T.);
#8135=ORIENTED_EDGE('',*,*,#5853,.F.);
#8136=ORIENTED_EDGE('',*,*,#5854,.F.);
#8137=ORIENTED_EDGE('',*,*,#5855,.T.);
#8138=ORIENTED_EDGE('',*,*,#5856,.T.);
#8139=ORIENTED_EDGE('',*,*,#5851,.F.);
#8140=ORIENTED_EDGE('',*,*,#5857,.F.);
#8141=ORIENTED_EDGE('',*,*,#5858,.T.);
#8142=ORIENTED_EDGE('',*,*,#5859,.T.);
#8143=ORIENTED_EDGE('',*,*,#5855,.F.);
#8144=ORIENTED_EDGE('',*,*,#5860,.F.);
#8145=ORIENTED_EDGE('',*,*,#5861,.T.);
#8146=ORIENTED_EDGE('',*,*,#5862,.T.);
#8147=ORIENTED_EDGE('',*,*,#5858,.F.);
#8148=ORIENTED_EDGE('',*,*,#5863,.F.);
#8149=ORIENTED_EDGE('',*,*,#5864,.T.);
#8150=ORIENTED_EDGE('',*,*,#5865,.T.);
#8151=ORIENTED_EDGE('',*,*,#5861,.F.);
#8152=ORIENTED_EDGE('',*,*,#5866,.F.);
#8153=ORIENTED_EDGE('',*,*,#5867,.T.);
#8154=ORIENTED_EDGE('',*,*,#5868,.T.);
#8155=ORIENTED_EDGE('',*,*,#5864,.F.);
#8156=ORIENTED_EDGE('',*,*,#5869,.F.);
#8157=ORIENTED_EDGE('',*,*,#5870,.T.);
#8158=ORIENTED_EDGE('',*,*,#5871,.T.);
#8159=ORIENTED_EDGE('',*,*,#5867,.F.);
#8160=ORIENTED_EDGE('',*,*,#5872,.F.);
#8161=ORIENTED_EDGE('',*,*,#5873,.T.);
#8162=ORIENTED_EDGE('',*,*,#5874,.T.);
#8163=ORIENTED_EDGE('',*,*,#5870,.F.);
#8164=ORIENTED_EDGE('',*,*,#5875,.F.);
#8165=ORIENTED_EDGE('',*,*,#5876,.T.);
#8166=ORIENTED_EDGE('',*,*,#5877,.T.);
#8167=ORIENTED_EDGE('',*,*,#5873,.F.);
#8168=ORIENTED_EDGE('',*,*,#5878,.F.);
#8169=ORIENTED_EDGE('',*,*,#5879,.T.);
#8170=ORIENTED_EDGE('',*,*,#5880,.T.);
#8171=ORIENTED_EDGE('',*,*,#5876,.F.);
#8172=ORIENTED_EDGE('',*,*,#5881,.F.);
#8173=ORIENTED_EDGE('',*,*,#5882,.T.);
#8174=ORIENTED_EDGE('',*,*,#5883,.T.);
#8175=ORIENTED_EDGE('',*,*,#5879,.F.);
#8176=ORIENTED_EDGE('',*,*,#5884,.F.);
#8177=ORIENTED_EDGE('',*,*,#5885,.T.);
#8178=ORIENTED_EDGE('',*,*,#5886,.T.);
#8179=ORIENTED_EDGE('',*,*,#5882,.F.);
#8180=ORIENTED_EDGE('',*,*,#5887,.F.);
#8181=ORIENTED_EDGE('',*,*,#5888,.F.);
#8182=ORIENTED_EDGE('',*,*,#5889,.F.);
#8183=ORIENTED_EDGE('',*,*,#5890,.F.);
#8184=ORIENTED_EDGE('',*,*,#5891,.T.);
#8185=ORIENTED_EDGE('',*,*,#5892,.T.);
#8186=ORIENTED_EDGE('',*,*,#5893,.T.);
#8187=ORIENTED_EDGE('',*,*,#5894,.F.);
#8188=ORIENTED_EDGE('',*,*,#5895,.T.);
#8189=ORIENTED_EDGE('',*,*,#5896,.T.);
#8190=ORIENTED_EDGE('',*,*,#5897,.T.);
#8191=ORIENTED_EDGE('',*,*,#5892,.F.);
#8192=ORIENTED_EDGE('',*,*,#5898,.T.);
#8193=ORIENTED_EDGE('',*,*,#5899,.T.);
#8194=ORIENTED_EDGE('',*,*,#5900,.T.);
#8195=ORIENTED_EDGE('',*,*,#5896,.F.);
#8196=ORIENTED_EDGE('',*,*,#5901,.T.);
#8197=ORIENTED_EDGE('',*,*,#5902,.T.);
#8198=ORIENTED_EDGE('',*,*,#5903,.T.);
#8199=ORIENTED_EDGE('',*,*,#5899,.F.);
#8200=ORIENTED_EDGE('',*,*,#5904,.T.);
#8201=ORIENTED_EDGE('',*,*,#5905,.T.);
#8202=ORIENTED_EDGE('',*,*,#5906,.T.);
#8203=ORIENTED_EDGE('',*,*,#5902,.F.);
#8204=ORIENTED_EDGE('',*,*,#5907,.T.);
#8205=ORIENTED_EDGE('',*,*,#5908,.T.);
#8206=ORIENTED_EDGE('',*,*,#5909,.T.);
#8207=ORIENTED_EDGE('',*,*,#5905,.F.);
#8208=ORIENTED_EDGE('',*,*,#5910,.T.);
#8209=ORIENTED_EDGE('',*,*,#5911,.T.);
#8210=ORIENTED_EDGE('',*,*,#5912,.T.);
#8211=ORIENTED_EDGE('',*,*,#5908,.F.);
#8212=ORIENTED_EDGE('',*,*,#5913,.T.);
#8213=ORIENTED_EDGE('',*,*,#5914,.F.);
#8214=ORIENTED_EDGE('',*,*,#5915,.T.);
#8215=ORIENTED_EDGE('',*,*,#5916,.F.);
#8216=ORIENTED_EDGE('',*,*,#5917,.T.);
#8217=ORIENTED_EDGE('',*,*,#5918,.T.);
#8218=ORIENTED_EDGE('',*,*,#5919,.T.);
#8219=ORIENTED_EDGE('',*,*,#5920,.F.);
#8220=ORIENTED_EDGE('',*,*,#5921,.T.);
#8221=ORIENTED_EDGE('',*,*,#5922,.T.);
#8222=ORIENTED_EDGE('',*,*,#5923,.T.);
#8223=ORIENTED_EDGE('',*,*,#5918,.F.);
#8224=ORIENTED_EDGE('',*,*,#5924,.T.);
#8225=ORIENTED_EDGE('',*,*,#5925,.T.);
#8226=ORIENTED_EDGE('',*,*,#5926,.T.);
#8227=ORIENTED_EDGE('',*,*,#5922,.F.);
#8228=ORIENTED_EDGE('',*,*,#5927,.T.);
#8229=ORIENTED_EDGE('',*,*,#5928,.T.);
#8230=ORIENTED_EDGE('',*,*,#5929,.T.);
#8231=ORIENTED_EDGE('',*,*,#5925,.F.);
#8232=ORIENTED_EDGE('',*,*,#5930,.T.);
#8233=ORIENTED_EDGE('',*,*,#5931,.T.);
#8234=ORIENTED_EDGE('',*,*,#5932,.T.);
#8235=ORIENTED_EDGE('',*,*,#5928,.F.);
#8236=ORIENTED_EDGE('',*,*,#5933,.T.);
#8237=ORIENTED_EDGE('',*,*,#5934,.T.);
#8238=ORIENTED_EDGE('',*,*,#5935,.T.);
#8239=ORIENTED_EDGE('',*,*,#5931,.F.);
#8240=ORIENTED_EDGE('',*,*,#5936,.T.);
#8241=ORIENTED_EDGE('',*,*,#5937,.T.);
#8242=ORIENTED_EDGE('',*,*,#5938,.T.);
#8243=ORIENTED_EDGE('',*,*,#5934,.F.);
#8244=ORIENTED_EDGE('',*,*,#5939,.T.);
#8245=ORIENTED_EDGE('',*,*,#5940,.F.);
#8246=ORIENTED_EDGE('',*,*,#5941,.T.);
#8247=ORIENTED_EDGE('',*,*,#5942,.F.);
#8248=ORIENTED_EDGE('',*,*,#5943,.T.);
#8249=ORIENTED_EDGE('',*,*,#5944,.T.);
#8250=ORIENTED_EDGE('',*,*,#5945,.T.);
#8251=ORIENTED_EDGE('',*,*,#5946,.F.);
#8252=ORIENTED_EDGE('',*,*,#5947,.F.);
#8253=ORIENTED_EDGE('',*,*,#5948,.T.);
#8254=ORIENTED_EDGE('',*,*,#5949,.T.);
#8255=ORIENTED_EDGE('',*,*,#5944,.F.);
#8256=ORIENTED_EDGE('',*,*,#5950,.F.);
#8257=ORIENTED_EDGE('',*,*,#5951,.T.);
#8258=ORIENTED_EDGE('',*,*,#5952,.T.);
#8259=ORIENTED_EDGE('',*,*,#5948,.F.);
#8260=ORIENTED_EDGE('',*,*,#5953,.F.);
#8261=ORIENTED_EDGE('',*,*,#5954,.T.);
#8262=ORIENTED_EDGE('',*,*,#5955,.T.);
#8263=ORIENTED_EDGE('',*,*,#5951,.F.);
#8264=ORIENTED_EDGE('',*,*,#5956,.F.);
#8265=ORIENTED_EDGE('',*,*,#5957,.T.);
#8266=ORIENTED_EDGE('',*,*,#5958,.T.);
#8267=ORIENTED_EDGE('',*,*,#5954,.F.);
#8268=ORIENTED_EDGE('',*,*,#5959,.F.);
#8269=ORIENTED_EDGE('',*,*,#5960,.T.);
#8270=ORIENTED_EDGE('',*,*,#5961,.T.);
#8271=ORIENTED_EDGE('',*,*,#5957,.F.);
#8272=ORIENTED_EDGE('',*,*,#5962,.F.);
#8273=ORIENTED_EDGE('',*,*,#5963,.T.);
#8274=ORIENTED_EDGE('',*,*,#5964,.T.);
#8275=ORIENTED_EDGE('',*,*,#5960,.F.);
#8276=ORIENTED_EDGE('',*,*,#5965,.F.);
#8277=ORIENTED_EDGE('',*,*,#5966,.F.);
#8278=ORIENTED_EDGE('',*,*,#5967,.F.);
#8279=ORIENTED_EDGE('',*,*,#5968,.F.);
#8280=ORIENTED_EDGE('',*,*,#5969,.T.);
#8281=ORIENTED_EDGE('',*,*,#5970,.T.);
#8282=ORIENTED_EDGE('',*,*,#5971,.T.);
#8283=ORIENTED_EDGE('',*,*,#5972,.F.);
#8284=ORIENTED_EDGE('',*,*,#5973,.F.);
#8285=ORIENTED_EDGE('',*,*,#5974,.T.);
#8286=ORIENTED_EDGE('',*,*,#5975,.T.);
#8287=ORIENTED_EDGE('',*,*,#5970,.F.);
#8288=ORIENTED_EDGE('',*,*,#5976,.F.);
#8289=ORIENTED_EDGE('',*,*,#5977,.T.);
#8290=ORIENTED_EDGE('',*,*,#5978,.T.);
#8291=ORIENTED_EDGE('',*,*,#5974,.F.);
#8292=ORIENTED_EDGE('',*,*,#5979,.F.);
#8293=ORIENTED_EDGE('',*,*,#5980,.T.);
#8294=ORIENTED_EDGE('',*,*,#5981,.T.);
#8295=ORIENTED_EDGE('',*,*,#5977,.F.);
#8296=ORIENTED_EDGE('',*,*,#5982,.F.);
#8297=ORIENTED_EDGE('',*,*,#5983,.T.);
#8298=ORIENTED_EDGE('',*,*,#5984,.T.);
#8299=ORIENTED_EDGE('',*,*,#5980,.F.);
#8300=ORIENTED_EDGE('',*,*,#5985,.F.);
#8301=ORIENTED_EDGE('',*,*,#5986,.T.);
#8302=ORIENTED_EDGE('',*,*,#5987,.T.);
#8303=ORIENTED_EDGE('',*,*,#5983,.F.);
#8304=ORIENTED_EDGE('',*,*,#5988,.F.);
#8305=ORIENTED_EDGE('',*,*,#5989,.T.);
#8306=ORIENTED_EDGE('',*,*,#5990,.T.);
#8307=ORIENTED_EDGE('',*,*,#5986,.F.);
#8308=ORIENTED_EDGE('',*,*,#5991,.F.);
#8309=ORIENTED_EDGE('',*,*,#5992,.F.);
#8310=ORIENTED_EDGE('',*,*,#5993,.F.);
#8311=ORIENTED_EDGE('',*,*,#5994,.F.);
#8312=ORIENTED_EDGE('',*,*,#5995,.T.);
#8313=ORIENTED_EDGE('',*,*,#5992,.T.);
#8314=ORIENTED_EDGE('',*,*,#5996,.T.);
#8315=ORIENTED_EDGE('',*,*,#5989,.F.);
#8316=ORIENTED_EDGE('',*,*,#5997,.F.);
#8317=ORIENTED_EDGE('',*,*,#5998,.F.);
#8318=ORIENTED_EDGE('',*,*,#5971,.F.);
#8319=ORIENTED_EDGE('',*,*,#5975,.F.);
#8320=ORIENTED_EDGE('',*,*,#5978,.F.);
#8321=ORIENTED_EDGE('',*,*,#5981,.F.);
#8322=ORIENTED_EDGE('',*,*,#5984,.F.);
#8323=ORIENTED_EDGE('',*,*,#5987,.F.);
#8324=ORIENTED_EDGE('',*,*,#5990,.F.);
#8325=ORIENTED_EDGE('',*,*,#5996,.F.);
#8326=ORIENTED_EDGE('',*,*,#5995,.F.);
#8327=ORIENTED_EDGE('',*,*,#5999,.F.);
#8328=ORIENTED_EDGE('',*,*,#5941,.F.);
#8329=ORIENTED_EDGE('',*,*,#6000,.F.);
#8330=ORIENTED_EDGE('',*,*,#5939,.F.);
#8331=ORIENTED_EDGE('',*,*,#5936,.F.);
#8332=ORIENTED_EDGE('',*,*,#5933,.F.);
#8333=ORIENTED_EDGE('',*,*,#5930,.F.);
#8334=ORIENTED_EDGE('',*,*,#5927,.F.);
#8335=ORIENTED_EDGE('',*,*,#5924,.F.);
#8336=ORIENTED_EDGE('',*,*,#5921,.F.);
#8337=ORIENTED_EDGE('',*,*,#6001,.F.);
#8338=ORIENTED_EDGE('',*,*,#5919,.F.);
#8339=ORIENTED_EDGE('',*,*,#5923,.F.);
#8340=ORIENTED_EDGE('',*,*,#5926,.F.);
#8341=ORIENTED_EDGE('',*,*,#5929,.F.);
#8342=ORIENTED_EDGE('',*,*,#5932,.F.);
#8343=ORIENTED_EDGE('',*,*,#5935,.F.);
#8344=ORIENTED_EDGE('',*,*,#5938,.F.);
#8345=ORIENTED_EDGE('',*,*,#6002,.F.);
#8346=ORIENTED_EDGE('',*,*,#5943,.F.);
#8347=ORIENTED_EDGE('',*,*,#6003,.F.);
#8348=ORIENTED_EDGE('',*,*,#5993,.T.);
#8349=ORIENTED_EDGE('',*,*,#5997,.T.);
#8350=ORIENTED_EDGE('',*,*,#5991,.T.);
#8351=ORIENTED_EDGE('',*,*,#5988,.T.);
#8352=ORIENTED_EDGE('',*,*,#5985,.T.);
#8353=ORIENTED_EDGE('',*,*,#5982,.T.);
#8354=ORIENTED_EDGE('',*,*,#5979,.T.);
#8355=ORIENTED_EDGE('',*,*,#5976,.T.);
#8356=ORIENTED_EDGE('',*,*,#5973,.T.);
#8357=ORIENTED_EDGE('',*,*,#6004,.F.);
#8358=ORIENTED_EDGE('',*,*,#6005,.F.);
#8359=ORIENTED_EDGE('',*,*,#6006,.F.);
#8360=ORIENTED_EDGE('',*,*,#6007,.F.);
#8361=ORIENTED_EDGE('',*,*,#6008,.F.);
#8362=ORIENTED_EDGE('',*,*,#6009,.F.);
#8363=ORIENTED_EDGE('',*,*,#6001,.T.);
#8364=ORIENTED_EDGE('',*,*,#5972,.T.);
#8365=ORIENTED_EDGE('',*,*,#5998,.T.);
#8366=ORIENTED_EDGE('',*,*,#5920,.T.);
#8367=ORIENTED_EDGE('',*,*,#6010,.T.);
#8368=ORIENTED_EDGE('',*,*,#5946,.T.);
#8369=ORIENTED_EDGE('',*,*,#6011,.T.);
#8370=ORIENTED_EDGE('',*,*,#5894,.T.);
#8371=ORIENTED_EDGE('',*,*,#5966,.T.);
#8372=ORIENTED_EDGE('',*,*,#6012,.T.);
#8373=ORIENTED_EDGE('',*,*,#5963,.F.);
#8374=ORIENTED_EDGE('',*,*,#6013,.F.);
#8375=ORIENTED_EDGE('',*,*,#6011,.F.);
#8376=ORIENTED_EDGE('',*,*,#5945,.F.);
#8377=ORIENTED_EDGE('',*,*,#5949,.F.);
#8378=ORIENTED_EDGE('',*,*,#5952,.F.);
#8379=ORIENTED_EDGE('',*,*,#5955,.F.);
#8380=ORIENTED_EDGE('',*,*,#5958,.F.);
#8381=ORIENTED_EDGE('',*,*,#5961,.F.);
#8382=ORIENTED_EDGE('',*,*,#5964,.F.);
#8383=ORIENTED_EDGE('',*,*,#6012,.F.);
#8384=ORIENTED_EDGE('',*,*,#5969,.F.);
#8385=ORIENTED_EDGE('',*,*,#6014,.F.);
#8386=ORIENTED_EDGE('',*,*,#5915,.F.);
#8387=ORIENTED_EDGE('',*,*,#6015,.F.);
#8388=ORIENTED_EDGE('',*,*,#5913,.F.);
#8389=ORIENTED_EDGE('',*,*,#5910,.F.);
#8390=ORIENTED_EDGE('',*,*,#5907,.F.);
#8391=ORIENTED_EDGE('',*,*,#5904,.F.);
#8392=ORIENTED_EDGE('',*,*,#5901,.F.);
#8393=ORIENTED_EDGE('',*,*,#5898,.F.);
#8394=ORIENTED_EDGE('',*,*,#5895,.F.);
#8395=ORIENTED_EDGE('',*,*,#6010,.F.);
#8396=ORIENTED_EDGE('',*,*,#5893,.F.);
#8397=ORIENTED_EDGE('',*,*,#5897,.F.);
#8398=ORIENTED_EDGE('',*,*,#5900,.F.);
#8399=ORIENTED_EDGE('',*,*,#5903,.F.);
#8400=ORIENTED_EDGE('',*,*,#5906,.F.);
#8401=ORIENTED_EDGE('',*,*,#5909,.F.);
#8402=ORIENTED_EDGE('',*,*,#5912,.F.);
#8403=ORIENTED_EDGE('',*,*,#6016,.F.);
#8404=ORIENTED_EDGE('',*,*,#5917,.F.);
#8405=ORIENTED_EDGE('',*,*,#6017,.F.);
#8406=ORIENTED_EDGE('',*,*,#5967,.T.);
#8407=ORIENTED_EDGE('',*,*,#6013,.T.);
#8408=ORIENTED_EDGE('',*,*,#5965,.T.);
#8409=ORIENTED_EDGE('',*,*,#5962,.T.);
#8410=ORIENTED_EDGE('',*,*,#5959,.T.);
#8411=ORIENTED_EDGE('',*,*,#5956,.T.);
#8412=ORIENTED_EDGE('',*,*,#5953,.T.);
#8413=ORIENTED_EDGE('',*,*,#5950,.T.);
#8414=ORIENTED_EDGE('',*,*,#5947,.T.);
#8415=ORIENTED_EDGE('',*,*,#5940,.T.);
#8416=ORIENTED_EDGE('',*,*,#6002,.T.);
#8417=ORIENTED_EDGE('',*,*,#5937,.F.);
#8418=ORIENTED_EDGE('',*,*,#6000,.T.);
#8419=ORIENTED_EDGE('',*,*,#5914,.T.);
#8420=ORIENTED_EDGE('',*,*,#6016,.T.);
#8421=ORIENTED_EDGE('',*,*,#5911,.F.);
#8422=ORIENTED_EDGE('',*,*,#6015,.T.);
#8423=ORIENTED_EDGE('',*,*,#5812,.F.);
#8424=ORIENTED_EDGE('',*,*,#6018,.T.);
#8425=ORIENTED_EDGE('',*,*,#5853,.T.);
#8426=ORIENTED_EDGE('',*,*,#6019,.T.);
#8427=ORIENTED_EDGE('',*,*,#5888,.T.);
#8428=ORIENTED_EDGE('',*,*,#6020,.T.);
#8429=ORIENTED_EDGE('',*,*,#5885,.F.);
#8430=ORIENTED_EDGE('',*,*,#6021,.F.);
#8431=ORIENTED_EDGE('',*,*,#6019,.F.);
#8432=ORIENTED_EDGE('',*,*,#5852,.F.);
#8433=ORIENTED_EDGE('',*,*,#5856,.F.);
#8434=ORIENTED_EDGE('',*,*,#5859,.F.);
#8435=ORIENTED_EDGE('',*,*,#5862,.F.);
#8436=ORIENTED_EDGE('',*,*,#5865,.F.);
#8437=ORIENTED_EDGE('',*,*,#5868,.F.);
#8438=ORIENTED_EDGE('',*,*,#5871,.F.);
#8439=ORIENTED_EDGE('',*,*,#5874,.F.);
#8440=ORIENTED_EDGE('',*,*,#5877,.F.);
#8441=ORIENTED_EDGE('',*,*,#5880,.F.);
#8442=ORIENTED_EDGE('',*,*,#5883,.F.);
#8443=ORIENTED_EDGE('',*,*,#5886,.F.);
#8444=ORIENTED_EDGE('',*,*,#6020,.F.);
#8445=ORIENTED_EDGE('',*,*,#5891,.F.);
#8446=ORIENTED_EDGE('',*,*,#6022,.F.);
#8447=ORIENTED_EDGE('',*,*,#5848,.F.);
#8448=ORIENTED_EDGE('',*,*,#6023,.F.);
#8449=ORIENTED_EDGE('',*,*,#5846,.F.);
#8450=ORIENTED_EDGE('',*,*,#5843,.F.);
#8451=ORIENTED_EDGE('',*,*,#5840,.F.);
#8452=ORIENTED_EDGE('',*,*,#5837,.F.);
#8453=ORIENTED_EDGE('',*,*,#5834,.F.);
#8454=ORIENTED_EDGE('',*,*,#5831,.F.);
#8455=ORIENTED_EDGE('',*,*,#5828,.F.);
#8456=ORIENTED_EDGE('',*,*,#5825,.F.);
#8457=ORIENTED_EDGE('',*,*,#5822,.F.);
#8458=ORIENTED_EDGE('',*,*,#5819,.F.);
#8459=ORIENTED_EDGE('',*,*,#5816,.F.);
#8460=ORIENTED_EDGE('',*,*,#5813,.F.);
#8461=ORIENTED_EDGE('',*,*,#6018,.F.);
#8462=ORIENTED_EDGE('',*,*,#5811,.F.);
#8463=ORIENTED_EDGE('',*,*,#5818,.F.);
#8464=ORIENTED_EDGE('',*,*,#5821,.F.);
#8465=ORIENTED_EDGE('',*,*,#5824,.F.);
#8466=ORIENTED_EDGE('',*,*,#5827,.F.);
#8467=ORIENTED_EDGE('',*,*,#5830,.F.);
#8468=ORIENTED_EDGE('',*,*,#5833,.F.);
#8469=ORIENTED_EDGE('',*,*,#5836,.F.);
#8470=ORIENTED_EDGE('',*,*,#5839,.F.);
#8471=ORIENTED_EDGE('',*,*,#5842,.F.);
#8472=ORIENTED_EDGE('',*,*,#5845,.F.);
#8473=ORIENTED_EDGE('',*,*,#6024,.F.);
#8474=ORIENTED_EDGE('',*,*,#5850,.F.);
#8475=ORIENTED_EDGE('',*,*,#6025,.F.);
#8476=ORIENTED_EDGE('',*,*,#5889,.T.);
#8477=ORIENTED_EDGE('',*,*,#6021,.T.);
#8478=ORIENTED_EDGE('',*,*,#5887,.T.);
#8479=ORIENTED_EDGE('',*,*,#5884,.T.);
#8480=ORIENTED_EDGE('',*,*,#5881,.T.);
#8481=ORIENTED_EDGE('',*,*,#5878,.T.);
#8482=ORIENTED_EDGE('',*,*,#5875,.T.);
#8483=ORIENTED_EDGE('',*,*,#5872,.T.);
#8484=ORIENTED_EDGE('',*,*,#5869,.T.);
#8485=ORIENTED_EDGE('',*,*,#5866,.T.);
#8486=ORIENTED_EDGE('',*,*,#5863,.T.);
#8487=ORIENTED_EDGE('',*,*,#5860,.T.);
#8488=ORIENTED_EDGE('',*,*,#5857,.T.);
#8489=ORIENTED_EDGE('',*,*,#5854,.T.);
#8490=ORIENTED_EDGE('',*,*,#5847,.T.);
#8491=ORIENTED_EDGE('',*,*,#6024,.T.);
#8492=ORIENTED_EDGE('',*,*,#5844,.F.);
#8493=ORIENTED_EDGE('',*,*,#6023,.T.);
#8494=ORIENTED_EDGE('',*,*,#5815,.F.);
#8495=ORIENTED_EDGE('',*,*,#6026,.F.);
#8496=ORIENTED_EDGE('',*,*,#6027,.T.);
#8497=ORIENTED_EDGE('',*,*,#6028,.F.);
#8498=ORIENTED_EDGE('',*,*,#6027,.F.);
#8499=ORIENTED_EDGE('',*,*,#6028,.T.);
#8500=ORIENTED_EDGE('',*,*,#6029,.T.);
#8501=ORIENTED_EDGE('',*,*,#6030,.T.);
#8502=ORIENTED_EDGE('',*,*,#6029,.F.);
#8503=ORIENTED_EDGE('',*,*,#6030,.F.);
#8504=ORIENTED_EDGE('',*,*,#6031,.T.);
#8505=ORIENTED_EDGE('',*,*,#6032,.F.);
#8506=ORIENTED_EDGE('',*,*,#6031,.F.);
#8507=ORIENTED_EDGE('',*,*,#6032,.T.);
#8508=ORIENTED_EDGE('',*,*,#6033,.T.);
#8509=ORIENTED_EDGE('',*,*,#6034,.F.);
#8510=ORIENTED_EDGE('',*,*,#6033,.F.);
#8511=ORIENTED_EDGE('',*,*,#6035,.T.);
#8512=ORIENTED_EDGE('',*,*,#6036,.F.);
#8513=ORIENTED_EDGE('',*,*,#6037,.F.);
#8514=ORIENTED_EDGE('',*,*,#6038,.F.);
#8515=ORIENTED_EDGE('',*,*,#6035,.F.);
#8516=ORIENTED_EDGE('',*,*,#6039,.T.);
#8517=ORIENTED_EDGE('',*,*,#6037,.T.);
#8518=ORIENTED_EDGE('',*,*,#6039,.F.);
#8519=ORIENTED_EDGE('',*,*,#6038,.T.);
#8520=ORIENTED_EDGE('',*,*,#6040,.T.);
#8521=ORIENTED_EDGE('',*,*,#6026,.T.);
#8522=ORIENTED_EDGE('',*,*,#6040,.F.);
#8523=ORIENTED_EDGE('',*,*,#6041,.F.);
#8524=ORIENTED_EDGE('',*,*,#6009,.T.);
#8525=ORIENTED_EDGE('',*,*,#6042,.T.);
#8526=ORIENTED_EDGE('',*,*,#6043,.F.);
#8527=ORIENTED_EDGE('',*,*,#6007,.T.);
#8528=ORIENTED_EDGE('',*,*,#6044,.T.);
#8529=ORIENTED_EDGE('',*,*,#6045,.F.);
#8530=ORIENTED_EDGE('',*,*,#6046,.F.);
#8531=ORIENTED_EDGE('',*,*,#6008,.T.);
#8532=ORIENTED_EDGE('',*,*,#6046,.T.);
#8533=ORIENTED_EDGE('',*,*,#6047,.F.);
#8534=ORIENTED_EDGE('',*,*,#6042,.F.);
#8535=ORIENTED_EDGE('',*,*,#6048,.F.);
#8536=ORIENTED_EDGE('',*,*,#6049,.F.);
#8537=ORIENTED_EDGE('',*,*,#6050,.F.);
#8538=ORIENTED_EDGE('',*,*,#6005,.T.);
#8539=ORIENTED_EDGE('',*,*,#6006,.T.);
#8540=ORIENTED_EDGE('',*,*,#6050,.T.);
#8541=ORIENTED_EDGE('',*,*,#6051,.F.);
#8542=ORIENTED_EDGE('',*,*,#6044,.F.);
#8543=ORIENTED_EDGE('',*,*,#6048,.T.);
#8544=ORIENTED_EDGE('',*,*,#6004,.T.);
#8545=ORIENTED_EDGE('',*,*,#6041,.T.);
#8546=ORIENTED_EDGE('',*,*,#6052,.F.);
#8547=ORIENTED_EDGE('',*,*,#6053,.F.);
#8548=ORIENTED_EDGE('',*,*,#6054,.T.);
#8549=ORIENTED_EDGE('',*,*,#6036,.T.);
#8550=ORIENTED_EDGE('',*,*,#6054,.F.);
#8551=ORIENTED_EDGE('',*,*,#6053,.T.);
#8552=ORIENTED_EDGE('',*,*,#6025,.T.);
#8553=ORIENTED_EDGE('',*,*,#5849,.T.);
#8554=ORIENTED_EDGE('',*,*,#6022,.T.);
#8555=ORIENTED_EDGE('',*,*,#5890,.T.);
#8556=ORIENTED_EDGE('',*,*,#6052,.T.);
#8557=ORIENTED_EDGE('',*,*,#6043,.T.);
#8558=ORIENTED_EDGE('',*,*,#6047,.T.);
#8559=ORIENTED_EDGE('',*,*,#6045,.T.);
#8560=ORIENTED_EDGE('',*,*,#6051,.T.);
#8561=ORIENTED_EDGE('',*,*,#6049,.T.);
#8562=ORIENTED_EDGE('',*,*,#6003,.T.);
#8563=ORIENTED_EDGE('',*,*,#5942,.T.);
#8564=ORIENTED_EDGE('',*,*,#5999,.T.);
#8565=ORIENTED_EDGE('',*,*,#5994,.T.);
#8566=ORIENTED_EDGE('',*,*,#6017,.T.);
#8567=ORIENTED_EDGE('',*,*,#5916,.T.);
#8568=ORIENTED_EDGE('',*,*,#6014,.T.);
#8569=ORIENTED_EDGE('',*,*,#5968,.T.);
#8570=ORIENTED_EDGE('',*,*,#6034,.T.);
#10338=CYLINDRICAL_SURFACE('',#11741,0.1666);
#10339=CYLINDRICAL_SURFACE('',#11744,0.1666);
#10340=CYLINDRICAL_SURFACE('',#11745,0.1666);
#10341=CYLINDRICAL_SURFACE('',#11746,0.1666);
#10342=CYLINDRICAL_SURFACE('',#11747,0.1666);
#10343=CYLINDRICAL_SURFACE('',#11748,0.1666);
#10344=CYLINDRICAL_SURFACE('',#11749,0.1666);
#10345=CYLINDRICAL_SURFACE('',#11750,0.1666);
#10346=CYLINDRICAL_SURFACE('',#11751,0.1666);
#10347=CYLINDRICAL_SURFACE('',#11752,0.1666);
#10348=CYLINDRICAL_SURFACE('',#11753,0.1666);
#10349=CYLINDRICAL_SURFACE('',#11754,0.1666);
#10350=CYLINDRICAL_SURFACE('',#11756,0.205475);
#10351=CYLINDRICAL_SURFACE('',#11758,0.205475);
#10352=CYLINDRICAL_SURFACE('',#11759,0.205475);
#10353=CYLINDRICAL_SURFACE('',#11760,0.205475);
#10354=CYLINDRICAL_SURFACE('',#11761,0.205475);
#10355=CYLINDRICAL_SURFACE('',#11762,0.205475);
#10356=CYLINDRICAL_SURFACE('',#11763,0.205475);
#10357=CYLINDRICAL_SURFACE('',#11764,0.205475);
#10358=CYLINDRICAL_SURFACE('',#11765,0.205475);
#10359=CYLINDRICAL_SURFACE('',#11766,0.205475);
#10360=CYLINDRICAL_SURFACE('',#11767,0.205475);
#10361=CYLINDRICAL_SURFACE('',#11768,0.205475);
#10362=CYLINDRICAL_SURFACE('',#11769,0.205475);
#10363=CYLINDRICAL_SURFACE('',#11771,0.12645);
#10364=CYLINDRICAL_SURFACE('',#11773,0.12645);
#10365=CYLINDRICAL_SURFACE('',#11774,0.12645);
#10366=CYLINDRICAL_SURFACE('',#11775,0.12645);
#10367=CYLINDRICAL_SURFACE('',#11776,0.12645);
#10368=CYLINDRICAL_SURFACE('',#11777,0.12645);
#10369=CYLINDRICAL_SURFACE('',#11778,0.12645);
#10370=CYLINDRICAL_SURFACE('',#11779,0.12645);
#10371=CYLINDRICAL_SURFACE('',#11781,0.12645);
#10372=CYLINDRICAL_SURFACE('',#11783,0.12645);
#10373=CYLINDRICAL_SURFACE('',#11784,0.12645);
#10374=CYLINDRICAL_SURFACE('',#11785,0.12645);
#10375=CYLINDRICAL_SURFACE('',#11786,0.12645);
#10376=CYLINDRICAL_SURFACE('',#11787,0.12645);
#10377=CYLINDRICAL_SURFACE('',#11788,0.12645);
#10378=CYLINDRICAL_SURFACE('',#11789,0.12645);
#10379=CYLINDRICAL_SURFACE('',#11791,0.1543);
#10380=CYLINDRICAL_SURFACE('',#11793,0.1543);
#10381=CYLINDRICAL_SURFACE('',#11794,0.1543);
#10382=CYLINDRICAL_SURFACE('',#11795,0.1543);
#10383=CYLINDRICAL_SURFACE('',#11796,0.1543);
#10384=CYLINDRICAL_SURFACE('',#11797,0.1543);
#10385=CYLINDRICAL_SURFACE('',#11798,0.1543);
#10386=CYLINDRICAL_SURFACE('',#11799,0.1543);
#10387=CYLINDRICAL_SURFACE('',#11801,0.1543);
#10388=CYLINDRICAL_SURFACE('',#11803,0.1543);
#10389=CYLINDRICAL_SURFACE('',#11804,0.1543);
#10390=CYLINDRICAL_SURFACE('',#11805,0.1543);
#10391=CYLINDRICAL_SURFACE('',#11806,0.1543);
#10392=CYLINDRICAL_SURFACE('',#11807,0.1543);
#10393=CYLINDRICAL_SURFACE('',#11808,0.1543);
#10394=CYLINDRICAL_SURFACE('',#11809,0.1543);
#10395=CYLINDRICAL_SURFACE('',#11811,0.1543);
#10396=CYLINDRICAL_SURFACE('',#11814,0.1543);
#10397=CYLINDRICAL_SURFACE('',#11815,0.12645);
#10398=CYLINDRICAL_SURFACE('',#11816,0.12645);
#10399=CYLINDRICAL_SURFACE('',#11818,0.205475);
#10400=CYLINDRICAL_SURFACE('',#11819,0.1666);
#10401=CYLINDRICAL_SURFACE('',#11825,0.6);
#10402=CYLINDRICAL_SURFACE('',#11830,0.6);
#10403=CYLINDRICAL_SURFACE('',#11838,1.);
#10404=CYLINDRICAL_SURFACE('',#11839,0.6);
#10405=CYLINDRICAL_SURFACE('',#11845,1.);
#10406=CYLINDRICAL_SURFACE('',#11847,0.6);
#10833=ADVANCED_FACE('',(#708),#10338,.F.);
#10834=ADVANCED_FACE('',(#709),#10339,.F.);
#10835=ADVANCED_FACE('',(#710),#10340,.F.);
#10836=ADVANCED_FACE('',(#711),#10341,.F.);
#10837=ADVANCED_FACE('',(#712),#10342,.F.);
#10838=ADVANCED_FACE('',(#713),#10343,.F.);
#10839=ADVANCED_FACE('',(#714),#10344,.F.);
#10840=ADVANCED_FACE('',(#715),#10345,.F.);
#10841=ADVANCED_FACE('',(#716),#10346,.F.);
#10842=ADVANCED_FACE('',(#717),#10347,.F.);
#10843=ADVANCED_FACE('',(#718),#10348,.F.);
#10844=ADVANCED_FACE('',(#719),#10349,.F.);
#10845=ADVANCED_FACE('',(#720),#10350,.F.);
#10846=ADVANCED_FACE('',(#721),#10351,.F.);
#10847=ADVANCED_FACE('',(#722),#10352,.F.);
#10848=ADVANCED_FACE('',(#723),#10353,.F.);
#10849=ADVANCED_FACE('',(#724),#10354,.F.);
#10850=ADVANCED_FACE('',(#725),#10355,.F.);
#10851=ADVANCED_FACE('',(#726),#10356,.F.);
#10852=ADVANCED_FACE('',(#727),#10357,.F.);
#10853=ADVANCED_FACE('',(#728),#10358,.F.);
#10854=ADVANCED_FACE('',(#729),#10359,.F.);
#10855=ADVANCED_FACE('',(#730),#10360,.F.);
#10856=ADVANCED_FACE('',(#731),#10361,.F.);
#10857=ADVANCED_FACE('',(#732),#10362,.F.);
#10858=ADVANCED_FACE('',(#733),#10363,.F.);
#10859=ADVANCED_FACE('',(#734),#10364,.F.);
#10860=ADVANCED_FACE('',(#735),#10365,.F.);
#10861=ADVANCED_FACE('',(#736),#10366,.F.);
#10862=ADVANCED_FACE('',(#737),#10367,.F.);
#10863=ADVANCED_FACE('',(#738),#10368,.F.);
#10864=ADVANCED_FACE('',(#739),#10369,.F.);
#10865=ADVANCED_FACE('',(#740),#10370,.F.);
#10866=ADVANCED_FACE('',(#741),#10371,.F.);
#10867=ADVANCED_FACE('',(#742),#10372,.F.);
#10868=ADVANCED_FACE('',(#743),#10373,.F.);
#10869=ADVANCED_FACE('',(#744),#10374,.F.);
#10870=ADVANCED_FACE('',(#745),#10375,.F.);
#10871=ADVANCED_FACE('',(#746),#10376,.F.);
#10872=ADVANCED_FACE('',(#747),#10377,.F.);
#10873=ADVANCED_FACE('',(#748),#10378,.F.);
#10874=ADVANCED_FACE('',(#749),#10379,.F.);
#10875=ADVANCED_FACE('',(#750),#10380,.F.);
#10876=ADVANCED_FACE('',(#751),#10381,.F.);
#10877=ADVANCED_FACE('',(#752),#10382,.F.);
#10878=ADVANCED_FACE('',(#753),#10383,.F.);
#10879=ADVANCED_FACE('',(#754),#10384,.F.);
#10880=ADVANCED_FACE('',(#755),#10385,.F.);
#10881=ADVANCED_FACE('',(#756),#10386,.F.);
#10882=ADVANCED_FACE('',(#757),#10387,.F.);
#10883=ADVANCED_FACE('',(#758),#10388,.F.);
#10884=ADVANCED_FACE('',(#759),#10389,.F.);
#10885=ADVANCED_FACE('',(#760),#10390,.F.);
#10886=ADVANCED_FACE('',(#761),#10391,.F.);
#10887=ADVANCED_FACE('',(#762),#10392,.F.);
#10888=ADVANCED_FACE('',(#763),#10393,.F.);
#10889=ADVANCED_FACE('',(#764),#10394,.F.);
#10890=ADVANCED_FACE('',(#765),#10395,.F.);
#10891=ADVANCED_FACE('',(#766),#236,.F.);
#10892=ADVANCED_FACE('',(#767),#237,.F.);
#10893=ADVANCED_FACE('',(#768,#298,#299),#388,.F.);
#10894=ADVANCED_FACE('',(#769),#10396,.F.);
#10895=ADVANCED_FACE('',(#770),#238,.F.);
#10896=ADVANCED_FACE('',(#771),#239,.F.);
#10897=ADVANCED_FACE('',(#772),#10397,.F.);
#10898=ADVANCED_FACE('',(#773),#10398,.F.);
#10899=ADVANCED_FACE('',(#774),#389,.T.);
#10900=ADVANCED_FACE('',(#775),#10399,.F.);
#10901=ADVANCED_FACE('',(#776),#240,.F.);
#10902=ADVANCED_FACE('',(#777),#241,.F.);
#10903=ADVANCED_FACE('',(#778),#10400,.F.);
#10904=ADVANCED_FACE('',(#779),#390,.F.);
#10905=ADVANCED_FACE('',(#780),#152,.F.);
#10906=ADVANCED_FACE('',(#781),#10401,.T.);
#10907=ADVANCED_FACE('',(#782),#153,.F.);
#10908=ADVANCED_FACE('',(#783),#10402,.T.);
#10909=ADVANCED_FACE('',(#784,#300),#391,.T.);
#10910=ADVANCED_FACE('',(#785,#301),#392,.F.);
#10911=ADVANCED_FACE('',(#786),#10403,.T.);
#10912=ADVANCED_FACE('',(#787),#10404,.T.);
#10913=ADVANCED_FACE('',(#788),#393,.T.);
#10914=ADVANCED_FACE('',(#789),#394,.T.);
#10915=ADVANCED_FACE('',(#790),#395,.T.);
#10916=ADVANCED_FACE('',(#791),#396,.T.);
#10917=ADVANCED_FACE('',(#792),#397,.T.);
#10918=ADVANCED_FACE('',(#793),#10405,.T.);
#10919=ADVANCED_FACE('',(#794),#10406,.T.);
#10920=ADVANCED_FACE('',(#795,#302),#398,.T.);
#10921=ADVANCED_FACE('',(#796,#303,#304,#305),#399,.T.);
#11234=CLOSED_SHELL('',(#10833,#10834,#10835,#10836,#10837,#10838,#10839,
#10840,#10841,#10842,#10843,#10844,#10845,#10846,#10847,#10848,#10849,#10850,
#10851,#10852,#10853,#10854,#10855,#10856,#10857,#10858,#10859,#10860,#10861,
#10862,#10863,#10864,#10865,#10866,#10867,#10868,#10869,#10870,#10871,#10872,
#10873,#10874,#10875,#10876,#10877,#10878,#10879,#10880,#10881,#10882,#10883,
#10884,#10885,#10886,#10887,#10888,#10889,#10890,#10891,#10892,#10893,#10894,
#10895,#10896,#10897,#10898,#10899,#10900,#10901,#10902,#10903,#10904,#10905,
#10906,#10907,#10908,#10909,#10910,#10911,#10912,#10913,#10914,#10915,#10916,
#10917,#10918,#10919,#10920,#10921));
#11740=AXIS2_PLACEMENT_3D('',#24815,#13107,#13108);
#11741=AXIS2_PLACEMENT_3D('',#24816,#13109,#13110);
#11742=AXIS2_PLACEMENT_3D('',#24844,#13112,#13113);
#11743=AXIS2_PLACEMENT_3D('',#24855,#13115,#13116);
#11744=AXIS2_PLACEMENT_3D('',#24878,#13117,#13118);
#11745=AXIS2_PLACEMENT_3D('',#24929,#13120,#13121);
#11746=AXIS2_PLACEMENT_3D('',#24977,#13123,#13124);
#11747=AXIS2_PLACEMENT_3D('',#25025,#13126,#13127);
#11748=AXIS2_PLACEMENT_3D('',#25076,#13129,#13130);
#11749=AXIS2_PLACEMENT_3D('',#25124,#13132,#13133);
#11750=AXIS2_PLACEMENT_3D('',#25172,#13135,#13136);
#11751=AXIS2_PLACEMENT_3D('',#25223,#13138,#13139);
#11752=AXIS2_PLACEMENT_3D('',#25274,#13141,#13142);
#11753=AXIS2_PLACEMENT_3D('',#25322,#13144,#13145);
#11754=AXIS2_PLACEMENT_3D('',#25373,#13147,#13148);
#11755=AXIS2_PLACEMENT_3D('',#25392,#13150,#13151);
#11756=AXIS2_PLACEMENT_3D('',#25412,#13152,#13153);
#11757=AXIS2_PLACEMENT_3D('',#25425,#13155,#13156);
#11758=AXIS2_PLACEMENT_3D('',#25434,#13157,#13158);
#11759=AXIS2_PLACEMENT_3D('',#25458,#13160,#13161);
#11760=AXIS2_PLACEMENT_3D('',#25483,#13163,#13164);
#11761=AXIS2_PLACEMENT_3D('',#25508,#13166,#13167);
#11762=AXIS2_PLACEMENT_3D('',#25532,#13169,#13170);
#11763=AXIS2_PLACEMENT_3D('',#25557,#13172,#13173);
#11764=AXIS2_PLACEMENT_3D('',#25581,#13175,#13176);
#11765=AXIS2_PLACEMENT_3D('',#25606,#13178,#13179);
#11766=AXIS2_PLACEMENT_3D('',#25630,#13181,#13182);
#11767=AXIS2_PLACEMENT_3D('',#25655,#13184,#13185);
#11768=AXIS2_PLACEMENT_3D('',#25680,#13187,#13188);
#11769=AXIS2_PLACEMENT_3D('',#25704,#13190,#13191);
#11770=AXIS2_PLACEMENT_3D('',#25715,#13193,#13194);
#11771=AXIS2_PLACEMENT_3D('',#25721,#13195,#13196);
#11772=AXIS2_PLACEMENT_3D('',#25731,#13198,#13199);
#11773=AXIS2_PLACEMENT_3D('',#25742,#13200,#13201);
#11774=AXIS2_PLACEMENT_3D('',#25793,#13203,#13204);
#11775=AXIS2_PLACEMENT_3D('',#25844,#13206,#13207);
#11776=AXIS2_PLACEMENT_3D('',#25892,#13209,#13210);
#11777=AXIS2_PLACEMENT_3D('',#25943,#13212,#13213);
#11778=AXIS2_PLACEMENT_3D('',#25994,#13215,#13216);
#11779=AXIS2_PLACEMENT_3D('',#26042,#13218,#13219);
#11780=AXIS2_PLACEMENT_3D('',#26061,#13221,#13222);
#11781=AXIS2_PLACEMENT_3D('',#26081,#13223,#13224);
#11782=AXIS2_PLACEMENT_3D('',#26091,#13226,#13227);
#11783=AXIS2_PLACEMENT_3D('',#26102,#13228,#13229);
#11784=AXIS2_PLACEMENT_3D('',#26153,#13231,#13232);
#11785=AXIS2_PLACEMENT_3D('',#26204,#13234,#13235);
#11786=AXIS2_PLACEMENT_3D('',#26252,#13237,#13238);
#11787=AXIS2_PLACEMENT_3D('',#26303,#13240,#13241);
#11788=AXIS2_PLACEMENT_3D('',#26354,#13243,#13244);
#11789=AXIS2_PLACEMENT_3D('',#26402,#13246,#13247);
#11790=AXIS2_PLACEMENT_3D('',#26421,#13249,#13250);
#11791=AXIS2_PLACEMENT_3D('',#26441,#13251,#13252);
#11792=AXIS2_PLACEMENT_3D('',#26455,#13254,#13255);
#11793=AXIS2_PLACEMENT_3D('',#26465,#13256,#13257);
#11794=AXIS2_PLACEMENT_3D('',#26489,#13259,#13260);
#11795=AXIS2_PLACEMENT_3D('',#26514,#13262,#13263);
#11796=AXIS2_PLACEMENT_3D('',#26539,#13265,#13266);
#11797=AXIS2_PLACEMENT_3D('',#26563,#13268,#13269);
#11798=AXIS2_PLACEMENT_3D('',#26588,#13271,#13272);
#11799=AXIS2_PLACEMENT_3D('',#26613,#13274,#13275);
#11800=AXIS2_PLACEMENT_3D('',#26624,#13277,#13278);
#11801=AXIS2_PLACEMENT_3D('',#26630,#13279,#13280);
#11802=AXIS2_PLACEMENT_3D('',#26644,#13282,#13283);
#11803=AXIS2_PLACEMENT_3D('',#26654,#13284,#13285);
#11804=AXIS2_PLACEMENT_3D('',#26678,#13287,#13288);
#11805=AXIS2_PLACEMENT_3D('',#26703,#13290,#13291);
#11806=AXIS2_PLACEMENT_3D('',#26728,#13293,#13294);
#11807=AXIS2_PLACEMENT_3D('',#26752,#13296,#13297);
#11808=AXIS2_PLACEMENT_3D('',#26777,#13299,#13300);
#11809=AXIS2_PLACEMENT_3D('',#26802,#13302,#13303);
#11810=AXIS2_PLACEMENT_3D('',#26813,#13305,#13306);
#11811=AXIS2_PLACEMENT_3D('',#26819,#13307,#13308);
#11812=AXIS2_PLACEMENT_3D('',#27541,#13309,#13310);
#11813=AXIS2_PLACEMENT_3D('',#27544,#13311,#13312);
#11814=AXIS2_PLACEMENT_3D('',#27655,#13318,#13319);
#11815=AXIS2_PLACEMENT_3D('',#28276,#13320,#13321);
#11816=AXIS2_PLACEMENT_3D('',#28277,#13322,#13323);
#11817=AXIS2_PLACEMENT_3D('',#28278,#13324,#13325);
#11818=AXIS2_PLACEMENT_3D('',#28389,#13326,#13327);
#11819=AXIS2_PLACEMENT_3D('',#29250,#13328,#13329);
#11820=AXIS2_PLACEMENT_3D('',#29251,#13330,#13331);
#11821=AXIS2_PLACEMENT_3D('',#29252,#13332,#13333);
#11822=AXIS2_PLACEMENT_3D('',#29254,#13334,#13335);
#11823=AXIS2_PLACEMENT_3D('',#29256,#13336,#13337);
#11824=AXIS2_PLACEMENT_3D('',#29257,#13338,#13339);
#11825=AXIS2_PLACEMENT_3D('',#29258,#13340,#13341);
#11826=AXIS2_PLACEMENT_3D('',#29261,#13343,#13344);
#11827=AXIS2_PLACEMENT_3D('',#29262,#13345,#13346);
#11828=AXIS2_PLACEMENT_3D('',#29264,#13347,#13348);
#11829=AXIS2_PLACEMENT_3D('',#29265,#13349,#13350);
#11830=AXIS2_PLACEMENT_3D('',#29266,#13351,#13352);
#11831=AXIS2_PLACEMENT_3D('',#29269,#13354,#13355);
#11832=AXIS2_PLACEMENT_3D('',#29270,#13356,#13357);
#11833=AXIS2_PLACEMENT_3D('',#29272,#13358,#13359);
#11834=AXIS2_PLACEMENT_3D('',#29274,#13360,#13361);
#11835=AXIS2_PLACEMENT_3D('',#29275,#13362,#13363);
#11836=AXIS2_PLACEMENT_3D('',#29277,#13364,#13365);
#11837=AXIS2_PLACEMENT_3D('',#29279,#13366,#13367);
#11838=AXIS2_PLACEMENT_3D('',#29280,#13368,#13369);
#11839=AXIS2_PLACEMENT_3D('',#29282,#13371,#13372);
#11840=AXIS2_PLACEMENT_3D('',#29284,#13374,#13375);
#11841=AXIS2_PLACEMENT_3D('',#29290,#13379,#13380);
#11842=AXIS2_PLACEMENT_3D('',#29296,#13384,#13385);
#11843=AXIS2_PLACEMENT_3D('',#29298,#13387,#13388);
#11844=AXIS2_PLACEMENT_3D('',#29304,#13392,#13393);
#11845=AXIS2_PLACEMENT_3D('',#29306,#13395,#13396);
#11846=AXIS2_PLACEMENT_3D('',#29307,#13397,#13398);
#11847=AXIS2_PLACEMENT_3D('',#29308,#13399,#13400);
#11848=AXIS2_PLACEMENT_3D('',#29310,#13401,#13402);
#11849=AXIS2_PLACEMENT_3D('',#29312,#13404,#13405);
#11850=AXIS2_PLACEMENT_3D('',#29313,#13406,#13407);
#13107=DIRECTION('axis',(0.,0.,1.));
#13108=DIRECTION('refdir',(1.,0.,0.));
#13109=DIRECTION('center_axis',(0.,0.,-1.));
#13110=DIRECTION('ref_axis',(1.,0.,0.));
#13111=DIRECTION('',(0.,0.,-1.));
#13112=DIRECTION('center_axis',(0.,0.,1.));
#13113=DIRECTION('ref_axis',(1.,0.,0.));
#13114=DIRECTION('',(0.,0.,-1.));
#13115=DIRECTION('center_axis',(0.,0.,1.));
#13116=DIRECTION('ref_axis',(1.,0.,0.));
#13117=DIRECTION('center_axis',(0.,0.,-1.));
#13118=DIRECTION('ref_axis',(1.,0.,0.));
#13119=DIRECTION('',(0.,0.,-1.));
#13120=DIRECTION('center_axis',(0.,0.,-1.));
#13121=DIRECTION('ref_axis',(1.,0.,0.));
#13122=DIRECTION('',(0.,0.,-1.));
#13123=DIRECTION('center_axis',(0.,0.,-1.));
#13124=DIRECTION('ref_axis',(1.,0.,0.));
#13125=DIRECTION('',(0.,0.,-1.));
#13126=DIRECTION('center_axis',(0.,0.,-1.));
#13127=DIRECTION('ref_axis',(1.,0.,0.));
#13128=DIRECTION('',(0.,0.,-1.));
#13129=DIRECTION('center_axis',(0.,0.,-1.));
#13130=DIRECTION('ref_axis',(1.,0.,0.));
#13131=DIRECTION('',(0.,0.,-1.));
#13132=DIRECTION('center_axis',(0.,0.,-1.));
#13133=DIRECTION('ref_axis',(1.,0.,0.));
#13134=DIRECTION('',(0.,0.,-1.));
#13135=DIRECTION('center_axis',(0.,0.,-1.));
#13136=DIRECTION('ref_axis',(1.,0.,0.));
#13137=DIRECTION('',(0.,0.,-1.));
#13138=DIRECTION('center_axis',(0.,0.,-1.));
#13139=DIRECTION('ref_axis',(1.,0.,0.));
#13140=DIRECTION('',(0.,0.,-1.));
#13141=DIRECTION('center_axis',(0.,0.,-1.));
#13142=DIRECTION('ref_axis',(1.,0.,0.));
#13143=DIRECTION('',(0.,0.,-1.));
#13144=DIRECTION('center_axis',(0.,0.,-1.));
#13145=DIRECTION('ref_axis',(1.,0.,0.));
#13146=DIRECTION('',(0.,0.,-1.));
#13147=DIRECTION('center_axis',(0.,0.,-1.));
#13148=DIRECTION('ref_axis',(0.938437868794217,-0.345448066158965,0.));
#13149=DIRECTION('',(0.,0.,-1.));
#13150=DIRECTION('center_axis',(0.,0.,-1.));
#13151=DIRECTION('ref_axis',(1.,0.,0.));
#13152=DIRECTION('center_axis',(0.,0.,-1.));
#13153=DIRECTION('ref_axis',(0.45014995938304,0.892952974163504,0.));
#13154=DIRECTION('',(1.22464679914735E-16,-8.10900634611207E-30,-1.));
#13155=DIRECTION('center_axis',(0.,0.,1.));
#13156=DIRECTION('ref_axis',(1.,-6.60925970975535E-14,0.));
#13157=DIRECTION('center_axis',(0.,0.,-1.));
#13158=DIRECTION('ref_axis',(1.,-6.60925970975535E-14,0.));
#13159=DIRECTION('',(1.22464679914735E-16,-8.10900634611207E-30,-1.));
#13160=DIRECTION('center_axis',(0.,0.,-1.));
#13161=DIRECTION('ref_axis',(1.,-6.60925970975535E-14,0.));
#13162=DIRECTION('',(1.22464679914735E-16,-8.10900634611207E-30,-1.));
#13163=DIRECTION('center_axis',(0.,0.,-1.));
#13164=DIRECTION('ref_axis',(1.,-6.60925970975535E-14,0.));
#13165=DIRECTION('',(1.22464679914735E-16,-8.10900634611207E-30,-1.));
#13166=DIRECTION('center_axis',(0.,0.,-1.));
#13167=DIRECTION('ref_axis',(1.,-6.60925970975535E-14,0.));
#13168=DIRECTION('',(1.22464679914735E-16,-8.10900634611207E-30,-1.));
#13169=DIRECTION('center_axis',(0.,0.,-1.));
#13170=DIRECTION('ref_axis',(1.,-6.60925970975535E-14,0.));
#13171=DIRECTION('',(1.22464679914735E-16,-8.10900634611207E-30,-1.));
#13172=DIRECTION('center_axis',(0.,0.,-1.));
#13173=DIRECTION('ref_axis',(1.,-6.60925970975535E-14,0.));
#13174=DIRECTION('',(1.22464679914735E-16,-8.10900634611207E-30,-1.));
#13175=DIRECTION('center_axis',(0.,0.,-1.));
#13176=DIRECTION('ref_axis',(1.,-6.60925970975535E-14,0.));
#13177=DIRECTION('',(1.22464679914735E-16,-8.10900634611207E-30,-1.));
#13178=DIRECTION('center_axis',(0.,0.,-1.));
#13179=DIRECTION('ref_axis',(1.,-6.60925970975535E-14,0.));
#13180=DIRECTION('',(1.22464679914735E-16,-8.10900634611207E-30,-1.));
#13181=DIRECTION('center_axis',(0.,0.,-1.));
#13182=DIRECTION('ref_axis',(1.,-6.60925970975535E-14,0.));
#13183=DIRECTION('',(1.22464679914735E-16,-8.10900634611207E-30,-1.));
#13184=DIRECTION('center_axis',(0.,0.,-1.));
#13185=DIRECTION('ref_axis',(1.,-6.60925970975535E-14,0.));
#13186=DIRECTION('',(1.22464679914735E-16,-8.10900634611207E-30,-1.));
#13187=DIRECTION('center_axis',(0.,0.,-1.));
#13188=DIRECTION('ref_axis',(1.,-6.60925970975535E-14,0.));
#13189=DIRECTION('',(1.22464679914735E-16,-8.10900634611207E-30,-1.));
#13190=DIRECTION('center_axis',(0.,0.,-1.));
#13191=DIRECTION('ref_axis',(-0.609343205350381,-0.792906588504171,0.));
#13192=DIRECTION('',(1.22464679914735E-16,-8.10900634611207E-30,-1.));
#13193=DIRECTION('center_axis',(0.,0.,-1.));
#13194=DIRECTION('ref_axis',(1.,-6.60925970975535E-14,0.));
#13195=DIRECTION('center_axis',(0.,0.,-1.));
#13196=DIRECTION('ref_axis',(-0.348549200809368,0.937290485716755,0.));
#13197=DIRECTION('',(0.,0.,-1.));
#13198=DIRECTION('center_axis',(0.,0.,-1.));
#13199=DIRECTION('ref_axis',(1.,0.,0.));
#13200=DIRECTION('center_axis',(0.,0.,-1.));
#13201=DIRECTION('ref_axis',(1.,0.,0.));
#13202=DIRECTION('',(0.,0.,-1.));
#13203=DIRECTION('center_axis',(0.,0.,-1.));
#13204=DIRECTION('ref_axis',(1.,0.,0.));
#13205=DIRECTION('',(0.,0.,-1.));
#13206=DIRECTION('center_axis',(0.,0.,-1.));
#13207=DIRECTION('ref_axis',(1.,0.,0.));
#13208=DIRECTION('',(0.,0.,-1.));
#13209=DIRECTION('center_axis',(0.,0.,-1.));
#13210=DIRECTION('ref_axis',(1.,0.,0.));
#13211=DIRECTION('',(0.,0.,-1.));
#13212=DIRECTION('center_axis',(0.,0.,-1.));
#13213=DIRECTION('ref_axis',(1.,0.,0.));
#13214=DIRECTION('',(0.,0.,-1.));
#13215=DIRECTION('center_axis',(0.,0.,-1.));
#13216=DIRECTION('ref_axis',(1.,0.,0.));
#13217=DIRECTION('',(0.,0.,-1.));
#13218=DIRECTION('center_axis',(0.,0.,-1.));
#13219=DIRECTION('ref_axis',(0.93737235570927,-0.348328963412538,0.));
#13220=DIRECTION('',(0.,0.,-1.));
#13221=DIRECTION('center_axis',(0.,0.,-1.));
#13222=DIRECTION('ref_axis',(1.,0.,0.));
#13223=DIRECTION('center_axis',(0.,0.,-1.));
#13224=DIRECTION('ref_axis',(-0.348549399150009,0.937290411960011,0.));
#13225=DIRECTION('',(0.,0.,-1.));
#13226=DIRECTION('center_axis',(0.,0.,-1.));
#13227=DIRECTION('ref_axis',(1.,0.,0.));
#13228=DIRECTION('center_axis',(0.,0.,-1.));
#13229=DIRECTION('ref_axis',(1.,0.,0.));
#13230=DIRECTION('',(0.,0.,-1.));
#13231=DIRECTION('center_axis',(0.,0.,-1.));
#13232=DIRECTION('ref_axis',(1.,0.,0.));
#13233=DIRECTION('',(0.,0.,-1.));
#13234=DIRECTION('center_axis',(0.,0.,-1.));
#13235=DIRECTION('ref_axis',(1.,0.,0.));
#13236=DIRECTION('',(0.,0.,-1.));
#13237=DIRECTION('center_axis',(0.,0.,-1.));
#13238=DIRECTION('ref_axis',(1.,0.,0.));
#13239=DIRECTION('',(0.,0.,-1.));
#13240=DIRECTION('center_axis',(0.,0.,-1.));
#13241=DIRECTION('ref_axis',(1.,0.,0.));
#13242=DIRECTION('',(0.,0.,-1.));
#13243=DIRECTION('center_axis',(0.,0.,-1.));
#13244=DIRECTION('ref_axis',(1.,0.,0.));
#13245=DIRECTION('',(0.,0.,-1.));
#13246=DIRECTION('center_axis',(0.,0.,-1.));
#13247=DIRECTION('ref_axis',(0.937372370252713,-0.348328924275332,0.));
#13248=DIRECTION('',(0.,0.,-1.));
#13249=DIRECTION('center_axis',(0.,0.,-1.));
#13250=DIRECTION('ref_axis',(1.,0.,0.));
#13251=DIRECTION('center_axis',(0.,0.,-1.));
#13252=DIRECTION('ref_axis',(0.793241641674985,0.608906969834288,0.));
#13253=DIRECTION('',(1.22464679914735E-16,-2.74659599554882E-30,-1.));
#13254=DIRECTION('center_axis',(0.,0.,1.));
#13255=DIRECTION('ref_axis',(1.,-2.23051936250031E-14,0.));
#13256=DIRECTION('center_axis',(0.,0.,-1.));
#13257=DIRECTION('ref_axis',(1.,-2.23051936250031E-14,0.));
#13258=DIRECTION('',(1.22464679914735E-16,-2.74659599554882E-30,-1.));
#13259=DIRECTION('center_axis',(0.,0.,-1.));
#13260=DIRECTION('ref_axis',(1.,-2.23051936250031E-14,0.));
#13261=DIRECTION('',(1.22464679914735E-16,-2.74659599554882E-30,-1.));
#13262=DIRECTION('center_axis',(0.,0.,-1.));
#13263=DIRECTION('ref_axis',(1.,-2.23051936250031E-14,0.));
#13264=DIRECTION('',(1.22464679914735E-16,-2.74659599554882E-30,-1.));
#13265=DIRECTION('center_axis',(0.,0.,-1.));
#13266=DIRECTION('ref_axis',(1.,-2.23051936250031E-14,0.));
#13267=DIRECTION('',(1.22464679914735E-16,-2.74659599554882E-30,-1.));
#13268=DIRECTION('center_axis',(0.,0.,-1.));
#13269=DIRECTION('ref_axis',(1.,-2.23051936250031E-14,0.));
#13270=DIRECTION('',(1.22464679914735E-16,-2.74659599554882E-30,-1.));
#13271=DIRECTION('center_axis',(0.,0.,-1.));
#13272=DIRECTION('ref_axis',(1.,-2.23051936250031E-14,0.));
#13273=DIRECTION('',(1.22464679914735E-16,-2.74659599554882E-30,-1.));
#13274=DIRECTION('center_axis',(0.,0.,-1.));
#13275=DIRECTION('ref_axis',(-0.609084174586186,-0.793105584565299,0.));
#13276=DIRECTION('',(1.22464679914735E-16,-2.74659599554882E-30,-1.));
#13277=DIRECTION('center_axis',(0.,0.,-1.));
#13278=DIRECTION('ref_axis',(1.,-2.23051936250031E-14,0.));
#13279=DIRECTION('center_axis',(0.,0.,-1.));
#13280=DIRECTION('ref_axis',(0.793241683023816,0.608906915967904,0.));
#13281=DIRECTION('',(1.22464679914735E-16,-2.65847991820295E-30,-1.));
#13282=DIRECTION('center_axis',(0.,0.,1.));
#13283=DIRECTION('ref_axis',(1.,-2.15856712500031E-14,0.));
#13284=DIRECTION('center_axis',(0.,0.,-1.));
#13285=DIRECTION('ref_axis',(1.,-2.15856712500031E-14,0.));
#13286=DIRECTION('',(1.22464679914735E-16,-2.65847991820295E-30,-1.));
#13287=DIRECTION('center_axis',(0.,0.,-1.));
#13288=DIRECTION('ref_axis',(1.,-2.15856712500031E-14,0.));
#13289=DIRECTION('',(1.22464679914735E-16,-2.65847991820295E-30,-1.));
#13290=DIRECTION('center_axis',(0.,0.,-1.));
#13291=DIRECTION('ref_axis',(1.,-2.15856712500031E-14,0.));
#13292=DIRECTION('',(1.22464679914735E-16,-2.65847991820295E-30,-1.));
#13293=DIRECTION('center_axis',(0.,0.,-1.));
#13294=DIRECTION('ref_axis',(1.,-2.15856712500031E-14,0.));
#13295=DIRECTION('',(1.22464679914735E-16,-2.65847991820295E-30,-1.));
#13296=DIRECTION('center_axis',(0.,0.,-1.));
#13297=DIRECTION('ref_axis',(1.,-2.15856712500031E-14,0.));
#13298=DIRECTION('',(1.22464679914735E-16,-2.65847991820295E-30,-1.));
#13299=DIRECTION('center_axis',(0.,0.,-1.));
#13300=DIRECTION('ref_axis',(1.,-2.15856712500031E-14,0.));
#13301=DIRECTION('',(1.22464679914735E-16,-2.65847991820295E-30,-1.));
#13302=DIRECTION('center_axis',(0.,0.,-1.));
#13303=DIRECTION('ref_axis',(-0.609084235810543,-0.793105537546604,0.));
#13304=DIRECTION('',(1.22464679914735E-16,-2.65847991820295E-30,-1.));
#13305=DIRECTION('center_axis',(0.,0.,-1.));
#13306=DIRECTION('ref_axis',(1.,-2.15856712500031E-14,0.));
#13307=DIRECTION('center_axis',(0.,0.,-1.));
#13308=DIRECTION('ref_axis',(1.,-2.15856712500031E-14,0.));
#13309=DIRECTION('center_axis',(0.,0.,1.));
#13310=DIRECTION('ref_axis',(1.,0.,0.));
#13311=DIRECTION('center_axis',(0.,0.,1.));
#13312=DIRECTION('ref_axis',(1.,0.,0.));
#13313=DIRECTION('',(1.,0.,0.));
#13314=DIRECTION('',(0.,-1.,0.));
#13315=DIRECTION('',(-1.,0.,0.));
#13316=DIRECTION('',(0.,1.,0.));
#13317=DIRECTION('',(1.,0.,0.));
#13318=DIRECTION('center_axis',(0.,0.,-1.));
#13319=DIRECTION('ref_axis',(1.,-2.23051936250031E-14,0.));
#13320=DIRECTION('center_axis',(0.,0.,-1.));
#13321=DIRECTION('ref_axis',(1.,0.,0.));
#13322=DIRECTION('center_axis',(0.,0.,-1.));
#13323=DIRECTION('ref_axis',(1.,0.,0.));
#13324=DIRECTION('center_axis',(0.,0.,1.));
#13325=DIRECTION('ref_axis',(1.,0.,0.));
#13326=DIRECTION('center_axis',(0.,0.,-1.));
#13327=DIRECTION('ref_axis',(1.,-6.60925970975535E-14,0.));
#13328=DIRECTION('center_axis',(0.,0.,-1.));
#13329=DIRECTION('ref_axis',(1.,0.,0.));
#13330=DIRECTION('center_axis',(0.,0.,-1.));
#13331=DIRECTION('ref_axis',(1.,0.,0.));
#13332=DIRECTION('center_axis',(0.,0.,1.));
#13333=DIRECTION('ref_axis',(1.,0.,0.));
#13334=DIRECTION('center_axis',(0.,0.,1.));
#13335=DIRECTION('ref_axis',(1.,0.,0.));
#13336=DIRECTION('center_axis',(-1.22464679914735E-16,1.,0.));
#13337=DIRECTION('ref_axis',(-1.,-1.22464679914735E-16,0.));
#13338=DIRECTION('center_axis',(0.,0.,-1.));
#13339=DIRECTION('ref_axis',(1.,0.,0.));
#13340=DIRECTION('center_axis',(0.,0.,1.));
#13341=DIRECTION('ref_axis',(1.,0.,0.));
#13342=DIRECTION('',(0.,0.,-1.));
#13343=DIRECTION('center_axis',(0.,0.,1.));
#13344=DIRECTION('ref_axis',(1.,0.,0.));
#13345=DIRECTION('center_axis',(0.,0.,1.));
#13346=DIRECTION('ref_axis',(1.,0.,0.));
#13347=DIRECTION('center_axis',(-1.22464679914735E-16,1.,0.));
#13348=DIRECTION('ref_axis',(-1.,-1.22464679914735E-16,0.));
#13349=DIRECTION('center_axis',(0.,0.,-1.));
#13350=DIRECTION('ref_axis',(1.,0.,0.));
#13351=DIRECTION('center_axis',(0.,0.,1.));
#13352=DIRECTION('ref_axis',(1.,0.,0.));
#13353=DIRECTION('',(0.,0.,-1.));
#13354=DIRECTION('center_axis',(0.,0.,-1.));
#13355=DIRECTION('ref_axis',(1.,0.,0.));
#13356=DIRECTION('center_axis',(0.,0.,1.));
#13357=DIRECTION('ref_axis',(1.,0.,0.));
#13358=DIRECTION('center_axis',(0.,0.,1.));
#13359=DIRECTION('ref_axis',(1.,0.,0.));
#13360=DIRECTION('center_axis',(0.,0.,1.));
#13361=DIRECTION('ref_axis',(1.,0.,0.));
#13362=DIRECTION('center_axis',(0.,0.,1.));
#13363=DIRECTION('ref_axis',(1.,0.,0.));
#13364=DIRECTION('center_axis',(0.,0.,1.));
#13365=DIRECTION('ref_axis',(1.,0.,0.));
#13366=DIRECTION('center_axis',(0.,0.,-1.));
#13367=DIRECTION('ref_axis',(1.,0.,0.));
#13368=DIRECTION('center_axis',(0.,0.,1.));
#13369=DIRECTION('ref_axis',(1.,0.,0.));
#13370=DIRECTION('',(0.,0.,-1.));
#13371=DIRECTION('center_axis',(0.,0.,1.));
#13372=DIRECTION('ref_axis',(1.,0.,0.));
#13373=DIRECTION('',(0.,0.,-1.));
#13374=DIRECTION('center_axis',(0.,-1.,0.));
#13375=DIRECTION('ref_axis',(1.,0.,0.));
#13376=DIRECTION('',(0.,0.,1.));
#13377=DIRECTION('',(0.,0.,1.));
#13378=DIRECTION('',(1.,0.,0.));
#13379=DIRECTION('center_axis',(0.,1.,0.));
#13380=DIRECTION('ref_axis',(-1.,0.,0.));
#13381=DIRECTION('',(0.,0.,1.));
#13382=DIRECTION('',(-1.,0.,0.));
#13383=DIRECTION('',(0.,0.,1.));
#13384=DIRECTION('center_axis',(1.,0.,0.));
#13385=DIRECTION('ref_axis',(0.,1.,0.));
#13386=DIRECTION('',(0.,1.,0.));
#13387=DIRECTION('center_axis',(0.,-1.,0.));
#13388=DIRECTION('ref_axis',(1.,0.,0.));
#13389=DIRECTION('',(0.,0.,-1.));
#13390=DIRECTION('',(1.,0.,0.));
#13391=DIRECTION('',(0.,0.,1.));
#13392=DIRECTION('center_axis',(-1.,0.,0.));
#13393=DIRECTION('ref_axis',(0.,-1.,0.));
#13394=DIRECTION('',(0.,-1.,0.));
#13395=DIRECTION('center_axis',(0.,0.,1.));
#13396=DIRECTION('ref_axis',(-1.83697019872103E-16,-1.,0.));
#13397=DIRECTION('center_axis',(0.,0.,1.));
#13398=DIRECTION('ref_axis',(1.,0.,0.));
#13399=DIRECTION('center_axis',(0.,0.,1.));
#13400=DIRECTION('ref_axis',(1.,0.,0.));
#13401=DIRECTION('center_axis',(0.,0.,1.));
#13402=DIRECTION('ref_axis',(1.,0.,0.));
#13403=DIRECTION('',(0.,0.,-1.));
#13404=DIRECTION('center_axis',(0.,0.,1.));
#13405=DIRECTION('ref_axis',(1.,0.,0.));
#13406=DIRECTION('center_axis',(0.,0.,1.));
#13407=DIRECTION('ref_axis',(1.,0.,0.));
#24815=CARTESIAN_POINT('',(0.,0.,0.));
#24816=CARTESIAN_POINT('Origin',(0.,0.,8.1));
#24817=CARTESIAN_POINT('',(-0.166755106676391,-0.000121435635125306,7.78714803633902));
#24818=CARTESIAN_POINT('',(-0.166799883948055,9.68813611086832E-5,7.76785196366098));
#24819=CARTESIAN_POINT('',(-0.1666,2.04026156737949E-17,8.1));
#24820=CARTESIAN_POINT('',(-0.163512932725147,-0.0319230454628249,7.7));
#24821=CARTESIAN_POINT('Ctrl Pts',(-0.166799883948055,9.68813611086832E-5,
7.76785196366098));
#24822=CARTESIAN_POINT('Ctrl Pts',(-0.166840645338411,0.00590548551433283,
7.76746222055426));
#24823=CARTESIAN_POINT('Ctrl Pts',(-0.166563633223871,0.0117101988552057,
7.76707247744754));
#24824=CARTESIAN_POINT('Ctrl Pts',(-0.165956013515963,0.0174801248594044,
7.76668273434082));
#24825=CARTESIAN_POINT('Ctrl Pts',(-0.16018045080637,0.0723245761391249,
7.76297813798855));
#24826=CARTESIAN_POINT('Ctrl Pts',(-0.124534715755048,0.124026015090588,
7.75927354163629));
#24827=CARTESIAN_POINT('Ctrl Pts',(-0.0753218907600186,0.148913777527237,
7.75556894528402));
#24828=CARTESIAN_POINT('Ctrl Pts',(-0.0261090657649881,0.173801539963886,
7.75186434893175));
#24829=CARTESIAN_POINT('Ctrl Pts',(0.0366708491737493,0.17187562588572,
7.74815975257948));
#24830=CARTESIAN_POINT('Ctrl Pts',(0.0842656460541181,0.144035707307694,
7.74445515622722));
#24831=CARTESIAN_POINT('Ctrl Pts',(0.131860442934486,0.116195788729669,
7.74075055987495));
#24832=CARTESIAN_POINT('Ctrl Pts',(0.164270121756485,0.0624418656517862,
7.73704596352268));
#24833=CARTESIAN_POINT('Ctrl Pts',(0.166703321037463,0.0073384302242929,
7.73334136717041));
#24834=CARTESIAN_POINT('Ctrl Pts',(0.169136520318441,-0.0477650052032019,
7.72963677081815));
#24835=CARTESIAN_POINT('Ctrl Pts',(0.141593240058396,-0.104217952980307,
7.72593217446588));
#24836=CARTESIAN_POINT('Ctrl Pts',(0.0965948053937569,-0.136111577080138,
7.72222757811361));
#24837=CARTESIAN_POINT('Ctrl Pts',(0.0515963707291191,-0.168005201179968,
7.71852298176134));
#24838=CARTESIAN_POINT('Ctrl Pts',(-0.0108572183401114,-0.175339501602526,
7.71481838540907));
#24839=CARTESIAN_POINT('Ctrl Pts',(-0.0619807511793317,-0.154911947739832,
7.7111137890568));
#24840=CARTESIAN_POINT('Ctrl Pts',(-0.113104284018553,-0.134484393877138,
7.70740919270453));
#24841=CARTESIAN_POINT('Ctrl Pts',(-0.152897760627764,-0.0862949857291892,
7.70370459635227));
#24842=CARTESIAN_POINT('Ctrl Pts',(-0.163512932725147,-0.0319230454628249,
7.7));
#24843=CARTESIAN_POINT('',(-0.00525765170773282,0.166819768394696,7.7));
#24844=CARTESIAN_POINT('Origin',(0.,0.,7.7));
#24845=CARTESIAN_POINT('',(-0.166344373414692,-6.51389168225824E-5,7.71714803633902));
#24846=CARTESIAN_POINT('Ctrl Pts',(-0.00525764907570514,0.166819936918742,
7.7));
#24847=CARTESIAN_POINT('Ctrl Pts',(-0.0593082520320288,0.165047155780287,
7.70363229181855));
#24848=CARTESIAN_POINT('Ctrl Pts',(-0.11251659993028,0.134577229369471,
7.70726458363711));
#24849=CARTESIAN_POINT('Ctrl Pts',(-0.141284856726116,0.0887831345736904,
7.71089687545566));
#24850=CARTESIAN_POINT('Ctrl Pts',(-0.157788211499337,0.0625126449052761,
7.71298059575011));
#24851=CARTESIAN_POINT('Ctrl Pts',(-0.166248526827595,0.0311990933978105,
7.71506431604457));
#24852=CARTESIAN_POINT('Ctrl Pts',(-0.166344373414692,-6.51389168225825E-5,
7.71714803633902));
#24853=CARTESIAN_POINT('',(-0.1666,-2.04026156737949E-17,7.6));
#24854=CARTESIAN_POINT('',(-0.1666,2.04026156737949E-17,8.1));
#24855=CARTESIAN_POINT('Origin',(0.,0.,7.6));
#24856=CARTESIAN_POINT('Ctrl Pts',(-0.166344373414692,-6.51389168225825E-5,
7.71714803633902));
#24857=CARTESIAN_POINT('Ctrl Pts',(-0.166418930176779,-0.0243848356437411,
7.71876891239684));
#24858=CARTESIAN_POINT('Ctrl Pts',(-0.161432221274225,-0.0486746897655862,
7.72038978845465));
#24859=CARTESIAN_POINT('Ctrl Pts',(-0.151232954480441,-0.0705377895071834,
7.72201066451247));
#24860=CARTESIAN_POINT('Ctrl Pts',(-0.127922000889724,-0.120507038643429,
7.72571526086474));
#24861=CARTESIAN_POINT('Ctrl Pts',(-0.0773819611304395,-0.157799535692006,
7.72941985721701));
#24862=CARTESIAN_POINT('Ctrl Pts',(-0.0227493309511543,-0.165321415232451,
7.73312445356928));
#24863=CARTESIAN_POINT('Ctrl Pts',(0.0318832992281324,-0.172843294772896,
7.73682904992154));
#24864=CARTESIAN_POINT('Ctrl Pts',(0.0906085198274197,-0.150594556805206,
7.74053364627381));
#24865=CARTESIAN_POINT('Ctrl Pts',(0.126553702502437,-0.10877093791917,
7.74423824262608));
#24866=CARTESIAN_POINT('Ctrl Pts',(0.162498885177452,-0.0669473190331356,
7.74794283897834));
#24867=CARTESIAN_POINT('Ctrl Pts',(0.175664029928199,-0.00554881922875591,
7.75164743533061));
#24868=CARTESIAN_POINT('Ctrl Pts',(0.160022369379138,0.0473319831645365,
7.75535203168288));
#24869=CARTESIAN_POINT('Ctrl Pts',(0.144380708830077,0.10021278555783,7.75905662803515));
#24870=CARTESIAN_POINT('Ctrl Pts',(0.0999322429812069,0.144575890540035,
7.76276122438742));
#24871=CARTESIAN_POINT('Ctrl Pts',(0.0470199032740834,0.160114846699796,
7.76646582073968));
#24872=CARTESIAN_POINT('Ctrl Pts',(-0.00589243643303862,0.175653802859556,
7.77017041709195));
#24873=CARTESIAN_POINT('Ctrl Pts',(-0.0672686499984137,0.162368610196872,
7.77387501344422));
#24874=CARTESIAN_POINT('Ctrl Pts',(-0.109019988249582,0.126341039149064,
7.77757960979649));
#24875=CARTESIAN_POINT('Ctrl Pts',(-0.144965839935877,0.0953230699114976,
7.78076908531066));
#24876=CARTESIAN_POINT('Ctrl Pts',(-0.166365019120212,0.0474476213275738,
7.78395856082484));
#24877=CARTESIAN_POINT('Ctrl Pts',(-0.166755106676391,-0.000121435635125306,
7.78714803633902));
#24878=CARTESIAN_POINT('Origin',(0.,0.,8.1));
#24879=CARTESIAN_POINT('',(-0.166723919921104,0.000132477254470589,7.85714803633902));
#24880=CARTESIAN_POINT('',(-0.16637029761803,8.32303651922684E-5,7.83785196366098));
#24881=CARTESIAN_POINT('',(-0.1666,2.04026156737949E-17,8.1));
#24882=CARTESIAN_POINT('Ctrl Pts',(-0.16637029761803,8.32303651922683E-5,
7.83785196366098));
#24883=CARTESIAN_POINT('Ctrl Pts',(-0.166471779784318,0.0225194758640918,
7.83635646533454));
#24884=CARTESIAN_POINT('Ctrl Pts',(-0.162250862274583,0.0449191273246156,
7.83486096700809));
#24885=CARTESIAN_POINT('Ctrl Pts',(-0.153526177634359,0.0654002352708428,
7.83336546868165));
#24886=CARTESIAN_POINT('Ctrl Pts',(-0.131913692804807,0.116135322329401,
7.82966087232938));
#24887=CARTESIAN_POINT('Ctrl Pts',(-0.0826645290024911,0.155097560201121,
7.82595627597712));
#24888=CARTESIAN_POINT('Ctrl Pts',(-0.0283176745893541,0.164455508498786,
7.82225167962485));
#24889=CARTESIAN_POINT('Ctrl Pts',(0.0260291798237814,0.173813456796451,
7.81854708327258));
#24890=CARTESIAN_POINT('Ctrl Pts',(0.085473724847738,0.153567115520063,
7.81484248692031));
#24891=CARTESIAN_POINT('Ctrl Pts',(0.12281048880676,0.112982637616973,7.81113789056804));
#24892=CARTESIAN_POINT('Ctrl Pts',(0.160147252765783,0.0723981597138804,
7.80743329421577));
#24893=CARTESIAN_POINT('Ctrl Pts',(0.175376235659869,0.0114755451840856,
7.8037286978635));
#24894=CARTESIAN_POINT('Ctrl Pts',(0.161528478593592,-0.0419042210738496,
7.80002410151124));
#24895=CARTESIAN_POINT('Ctrl Pts',(0.147680721527315,-0.0952839873317826,
7.79631950515897));
#24896=CARTESIAN_POINT('Ctrl Pts',(0.104756224500674,-0.141120905317855,
7.7926149088067));
#24897=CARTESIAN_POINT('Ctrl Pts',(0.0523982952481369,-0.158436269366283,
7.78891031245443));
#24898=CARTESIAN_POINT('Ctrl Pts',(4.03659955982363E-5,-0.175751633414712,
7.78520571610217));
#24899=CARTESIAN_POINT('Ctrl Pts',(-0.0617509954828385,-0.164545443525494,
7.7815011197499));
#24900=CARTESIAN_POINT('Ctrl Pts',(-0.104693981038127,-0.129948616776896,
7.77779652339763));
#24901=CARTESIAN_POINT('Ctrl Pts',(-0.143119137655905,-0.098991558968666,
7.77448167015208));
#24902=CARTESIAN_POINT('Ctrl Pts',(-0.166453199106715,-0.0493066103172041,
7.77116681690653));
#24903=CARTESIAN_POINT('Ctrl Pts',(-0.166799883948055,9.68813611086832E-5,
7.76785196366098));
#24904=CARTESIAN_POINT('Ctrl Pts',(-0.166755106676391,-0.000121435635125306,
7.78714803633902));
#24905=CARTESIAN_POINT('Ctrl Pts',(-0.166818108329162,-0.00780414471406952,
7.78766315717711));
#24906=CARTESIAN_POINT('Ctrl Pts',(-0.166333101894556,-0.0154788617727347,
7.7881782780152));
#24907=CARTESIAN_POINT('Ctrl Pts',(-0.165272862574954,-0.0230732790724375,
7.78869339885329));
#24908=CARTESIAN_POINT('Ctrl Pts',(-0.157647935712195,-0.0776900768131957,
7.79239799520556));
#24909=CARTESIAN_POINT('Ctrl Pts',(-0.120271619049716,-0.128153722861778,
7.79610259155783));
#24910=CARTESIAN_POINT('Ctrl Pts',(-0.0702495033623604,-0.151368804567472,
7.7998071879101));
#24911=CARTESIAN_POINT('Ctrl Pts',(-0.0202273876750051,-0.174583886273165,
7.80351178426237));
#24912=CARTESIAN_POINT('Ctrl Pts',(0.0424405270372255,-0.17055040363597,
7.80721638061463));
#24913=CARTESIAN_POINT('Ctrl Pts',(0.0890739684606603,-0.1411145241273,
7.8109209769669));
#24914=CARTESIAN_POINT('Ctrl Pts',(0.135707409884095,-0.111678644618631,
7.81462557331917));
#24915=CARTESIAN_POINT('Ctrl Pts',(0.166306378018734,-0.0568403682384865,
7.81833016967144));
#24916=CARTESIAN_POINT('Ctrl Pts',(0.166867054261352,-0.00169663156977216,
7.82203476602371));
#24917=CARTESIAN_POINT('Ctrl Pts',(0.16742773050397,0.0534471050989422,
7.82573936237597));
#24918=CARTESIAN_POINT('Ctrl Pts',(0.137950114854567,0.108896302056227,
7.82944395872824));
#24919=CARTESIAN_POINT('Ctrl Pts',(0.0919248190425322,0.139274263653544,
7.83314855508051));
#24920=CARTESIAN_POINT('Ctrl Pts',(0.0458995232304963,0.169652225250862,
7.83685315143278));
#24921=CARTESIAN_POINT('Ctrl Pts',(-0.0166734527441725,0.174958951488212,
7.84055774778505));
#24922=CARTESIAN_POINT('Ctrl Pts',(-0.0671572385601096,0.152765817367363,
7.84426234413731));
#24923=CARTESIAN_POINT('Ctrl Pts',(-0.117641024376046,0.130572683246515,
7.84796694048958));
#24924=CARTESIAN_POINT('Ctrl Pts',(-0.156035620033251,0.0808796887674675,
7.85167153684185));
#24925=CARTESIAN_POINT('Ctrl Pts',(-0.16476951761495,0.0264291003362266,
7.85537613319412));
#24926=CARTESIAN_POINT('Ctrl Pts',(-0.166161987861879,0.0177478874402586,
7.85596676757575));
#24927=CARTESIAN_POINT('Ctrl Pts',(-0.166800517689049,0.00894574204390801,
7.85655740195739));
#24928=CARTESIAN_POINT('Ctrl Pts',(-0.166723919921104,0.000132477254470589,
7.85714803633902));
#24929=CARTESIAN_POINT('Origin',(0.,0.,8.1));
#24930=CARTESIAN_POINT('',(-0.166337147585101,3.80246141342272E-5,7.92714803633902));
#24931=CARTESIAN_POINT('',(-0.166497798286919,-0.000143128711388071,7.90785196366098));
#24932=CARTESIAN_POINT('',(-0.1666,2.04026156737949E-17,8.1));
#24933=CARTESIAN_POINT('Ctrl Pts',(-0.166497798286919,-0.000143128711388071,
7.90785196366098));
#24934=CARTESIAN_POINT('Ctrl Pts',(-0.166178683426007,0.0388071044866986,
7.90525071011481));
#24935=CARTESIAN_POINT('Ctrl Pts',(-0.1525429547553,0.077958624681208,7.90264945656864));
#24936=CARTESIAN_POINT('Ctrl Pts',(-0.127583662987733,0.107563455699431,
7.90004820302248));
#24937=CARTESIAN_POINT('Ctrl Pts',(-0.0920376850212504,0.149725416097789,
7.89634360667021));
#24938=CARTESIAN_POINT('Ctrl Pts',(-0.0335249580924989,0.172524530026611,
7.89263901031793));
#24939=CARTESIAN_POINT('Ctrl Pts',(0.0211758393351308,0.165526651230438,
7.88893441396567));
#24940=CARTESIAN_POINT('Ctrl Pts',(0.075876636762759,0.158528772434265,
7.8852298176134));
#24941=CARTESIAN_POINT('Ctrl Pts',(0.126765504689265,0.121733900913099,
7.88152522126114));
#24942=CARTESIAN_POINT('Ctrl Pts',(0.150552858584944,0.0719814231904523,
7.87782062490887));
#24943=CARTESIAN_POINT('Ctrl Pts',(0.174340212480624,0.0222289454678044,
7.8741160285566));
#24944=CARTESIAN_POINT('Ctrl Pts',(0.171026052345475,-0.0404811384563263,
7.87041143220433));
#24945=CARTESIAN_POINT('Ctrl Pts',(0.142127133392108,-0.087449212862691,
7.86670683585206));
#24946=CARTESIAN_POINT('Ctrl Pts',(0.113228214438741,-0.134417287269055,
7.86300223949979));
#24947=CARTESIAN_POINT('Ctrl Pts',(0.0587445366671569,-0.165643352157655,
7.85929764314753));
#24948=CARTESIAN_POINT('Ctrl Pts',(0.00361084226918911,-0.166836602473997,
7.85559304679526));
#24949=CARTESIAN_POINT('Ctrl Pts',(-0.051522852128781,-0.168029852790339,
7.85188845044299));
#24950=CARTESIAN_POINT('Ctrl Pts',(-0.107306563153134,-0.139190288534421,
7.84818385409072));
#24951=CARTESIAN_POINT('Ctrl Pts',(-0.138210515736916,-0.0935165382837624,
7.84447925773845));
#24952=CARTESIAN_POINT('Ctrl Pts',(-0.156638936582612,-0.0662806988247655,
7.84227015971263));
#24953=CARTESIAN_POINT('Ctrl Pts',(-0.166220391697549,-0.0330588098244754,
7.8400610616868));
#24954=CARTESIAN_POINT('Ctrl Pts',(-0.16637029761803,8.32303651922683E-5,
7.83785196366098));
#24955=CARTESIAN_POINT('Ctrl Pts',(-0.166723919921104,0.000132477254470589,
7.85714803633902));
#24956=CARTESIAN_POINT('Ctrl Pts',(-0.166320078655114,-0.0463331066073077,
7.86026199830966));
#24957=CARTESIAN_POINT('Ctrl Pts',(-0.146038236890536,-0.0931077699995557,
7.86337596028029));
#24958=CARTESIAN_POINT('Ctrl Pts',(-0.111566386808172,-0.124098479205671,
7.86648992225092));
#24959=CARTESIAN_POINT('Ctrl Pts',(-0.0705561589135018,-0.160967287932896,
7.87019451860319));
#24960=CARTESIAN_POINT('Ctrl Pts',(-0.00946250361796861,-0.17549672300391,
7.87389911495546));
#24961=CARTESIAN_POINT('Ctrl Pts',(0.043754722198001,-0.161037309704663,
7.87760371130772));
#24962=CARTESIAN_POINT('Ctrl Pts',(0.0969719480139703,-0.146577896405417,
7.88130830765999));
#24963=CARTESIAN_POINT('Ctrl Pts',(0.142312744350376,-0.10312963473591,
7.88501290401226));
#24964=CARTESIAN_POINT('Ctrl Pts',(0.159026638215273,-0.0505768661856178,
7.88871750036453));
#24965=CARTESIAN_POINT('Ctrl Pts',(0.17574053208017,0.00197590236467367,
7.8924220967168));
#24966=CARTESIAN_POINT('Ctrl Pts',(0.16382752347356,0.0636331777957509,
7.89612669306907));
#24967=CARTESIAN_POINT('Ctrl Pts',(0.128739668561873,0.106177157462437,
7.89983128942133));
#24968=CARTESIAN_POINT('Ctrl Pts',(0.0936518136501853,0.148721137129124,
7.9035358857736));
#24969=CARTESIAN_POINT('Ctrl Pts',(0.0353891124334194,0.17215182103142,
7.90724048212587));
#24970=CARTESIAN_POINT('Ctrl Pts',(-0.0193841796186578,0.165746024286076,
7.91094507847814));
#24971=CARTESIAN_POINT('Ctrl Pts',(-0.0741574716707353,0.159340227540732,
7.91464967483041));
#24972=CARTESIAN_POINT('Ctrl Pts',(-0.125441354558124,0.123097950147749,
7.91835427118268));
#24973=CARTESIAN_POINT('Ctrl Pts',(-0.149765468420507,0.0736056756289514,
7.92205886753494));
#24974=CARTESIAN_POINT('Ctrl Pts',(-0.160903840835397,0.0509424292566785,
7.9237552571363));
#24975=CARTESIAN_POINT('Ctrl Pts',(-0.166389127400799,0.0255008441238536,
7.92545164673766));
#24976=CARTESIAN_POINT('Ctrl Pts',(-0.166337147585101,3.80246141342272E-5,
7.92714803633902));
#24977=CARTESIAN_POINT('Origin',(0.,0.,8.1));
#24978=CARTESIAN_POINT('',(-0.166584472654422,-0.000152342595601075,7.99714803633902));
#24979=CARTESIAN_POINT('',(-0.166875664957045,6.71117862603047E-7,7.97785196366098));
#24980=CARTESIAN_POINT('',(-0.1666,2.04026156737949E-17,8.1));
#24981=CARTESIAN_POINT('Ctrl Pts',(-0.166875663578624,6.71114506779717E-7,
7.97785196366098));
#24982=CARTESIAN_POINT('Ctrl Pts',(-0.166878959491358,0.055183185010619,
7.97414495489508));
#24983=CARTESIAN_POINT('Ctrl Pts',(-0.136794342365432,0.110362609757235,
7.97043794612919));
#24984=CARTESIAN_POINT('Ctrl Pts',(-0.0904129758162234,0.140260407963621,
7.9667309373633));
#24985=CARTESIAN_POINT('Ctrl Pts',(-0.0440617929130959,0.170138749551395,
7.96302634101103));
#24986=CARTESIAN_POINT('Ctrl Pts',(0.0185649237682023,0.174768358996025,
7.95932174465876));
#24987=CARTESIAN_POINT('Ctrl Pts',(0.0688057022669373,0.152030469242651,
7.95561714830649));
#24988=CARTESIAN_POINT('Ctrl Pts',(0.119046480765674,0.129292579489277,
7.95191255195423));
#24989=CARTESIAN_POINT('Ctrl Pts',(0.156901321081846,0.0791871905378969,
7.94820795560196));
#24990=CARTESIAN_POINT('Ctrl Pts',(0.165045740801789,0.0246453178400153,
7.94450335924969));
#24991=CARTESIAN_POINT('Ctrl Pts',(0.173190160521732,-0.0298965548578656,
7.94079876289742));
#24992=CARTESIAN_POINT('Ctrl Pts',(0.151624159645446,-0.088874911302248,
7.93709416654516));
#24993=CARTESIAN_POINT('Ctrl Pts',(0.110217540942827,-0.125297972397028,
7.93338957019289));
#24994=CARTESIAN_POINT('Ctrl Pts',(0.0688109222402075,-0.161721033491808,
7.92968497384062));
#24995=CARTESIAN_POINT('Ctrl Pts',(0.00756368571125483,-0.175588799236986,
7.92598037748835));
#24996=CARTESIAN_POINT('Ctrl Pts',(-0.0454940239107126,-0.160554607684999,
7.92227578113608));
#24997=CARTESIAN_POINT('Ctrl Pts',(-0.0985517335326801,-0.145520416133013,
7.91857118478381));
#24998=CARTESIAN_POINT('Ctrl Pts',(-0.143419916247662,-0.101584267283862,
7.91486658843155));
#24999=CARTESIAN_POINT('Ctrl Pts',(-0.159564393103046,-0.0488537894253407,
7.91116199207928));
#25000=CARTESIAN_POINT('Ctrl Pts',(-0.164372715171855,-0.0331490302896252,
7.91005864927318));
#25001=CARTESIAN_POINT('Ctrl Pts',(-0.166633153445445,-0.0166641862831651,
7.90895530646708));
#25002=CARTESIAN_POINT('Ctrl Pts',(-0.166497798286919,-0.000143128711388071,
7.90785196366098));
#25003=CARTESIAN_POINT('Ctrl Pts',(-0.166337147585101,3.80246141342272E-5,
7.92714803633902));
#25004=CARTESIAN_POINT('Ctrl Pts',(-0.166275613243749,-0.0301051724413385,
7.92915624308993));
#25005=CARTESIAN_POINT('Ctrl Pts',(-0.158454090740355,-0.0602781275943973,
7.93116444984084));
#25006=CARTESIAN_POINT('Ctrl Pts',(-0.143064725491982,-0.085906782795492,
7.93317265659175));
#25007=CARTESIAN_POINT('Ctrl Pts',(-0.114675523863702,-0.133184695056525,
7.93687725294402));
#25008=CARTESIAN_POINT('Ctrl Pts',(-0.0605327757697651,-0.164998247933979,
7.94058184929628));
#25009=CARTESIAN_POINT('Ctrl Pts',(-0.00541521687100755,-0.166787788618045,
7.94428644564855));
#25010=CARTESIAN_POINT('Ctrl Pts',(0.04970234202775,-0.168577329302111,
7.94799104200082));
#25011=CARTESIAN_POINT('Ctrl Pts',(0.105794711731329,-0.140342857792789,
7.95169563835309));
#25012=CARTESIAN_POINT('Ctrl Pts',(0.137190901172147,-0.0950060400465786,
7.95540023470536));
#25013=CARTESIAN_POINT('Ctrl Pts',(0.168587090612965,-0.0496692223003677,
7.95910483105762));
#25014=CARTESIAN_POINT('Ctrl Pts',(0.175287099791022,0.0127699416827313,
7.9628094274099));
#25015=CARTESIAN_POINT('Ctrl Pts',(0.154224631518061,0.0637358144365465,
7.96651402376216));
#25016=CARTESIAN_POINT('Ctrl Pts',(0.133162163245099,0.114701687190362,
7.97021862011443));
#25017=CARTESIAN_POINT('Ctrl Pts',(0.0843372175211171,0.154194268714893,
7.9739232164667));
#25018=CARTESIAN_POINT('Ctrl Pts',(0.0300948076110954,0.164139555144915,
7.97762781281897));
#25019=CARTESIAN_POINT('Ctrl Pts',(-0.0241476022989255,0.174084841574938,
7.98133240917123));
#25020=CARTESIAN_POINT('Ctrl Pts',(-0.0838074763949865,0.154482832910453,
7.9850370055235));
#25021=CARTESIAN_POINT('Ctrl Pts',(-0.121581135001586,0.114304499563856,
7.98874160187577));
#25022=CARTESIAN_POINT('Ctrl Pts',(-0.150153009444279,0.083913736846075,
7.99154374669685));
#25023=CARTESIAN_POINT('Ctrl Pts',(-0.16620298954139,0.041750515622899,
7.99434589151794));
#25024=CARTESIAN_POINT('Ctrl Pts',(-0.166584472654422,-0.000152342595601075,
7.99714803633902));
#25025=CARTESIAN_POINT('Origin',(0.,0.,8.1));
#25026=CARTESIAN_POINT('',(-0.166853498321983,5.50350387731602E-5,8.06714803633902));
#25027=CARTESIAN_POINT('',(-0.166495840369714,0.000142706802959736,8.04785196366098));
#25028=CARTESIAN_POINT('',(-0.1666,2.04026156737949E-17,8.1));
#25029=CARTESIAN_POINT('Ctrl Pts',(-0.166495840369714,0.000142706802959736,
8.04785196366098));
#25030=CARTESIAN_POINT('Ctrl Pts',(-0.166631270248863,0.0167365034787871,
8.04674379602763));
#25031=CARTESIAN_POINT('Ctrl Pts',(-0.164350623819369,0.0332939115131789,
8.04563562839428));
#25032=CARTESIAN_POINT('Ctrl Pts',(-0.159500786113399,0.0490610585913692,
8.04452746076093));
#25033=CARTESIAN_POINT('Ctrl Pts',(-0.143287813875328,0.101770516793988,
8.04082286440866));
#25034=CARTESIAN_POINT('Ctrl Pts',(-0.0983625864380453,0.145648334294652,
8.03711826805639));
#25035=CARTESIAN_POINT('Ctrl Pts',(-0.0452853888819718,0.160613579110374,
8.03341367170412));
#25036=CARTESIAN_POINT('Ctrl Pts',(0.00779180867410008,0.175578823926095,
8.02970907535185));
#25037=CARTESIAN_POINT('Ctrl Pts',(0.0690209763489626,0.161631496056876,
8.02600447899959));
#25038=CARTESIAN_POINT('Ctrl Pts',(0.110380238363978,0.12515466918812,8.02229988264732));
#25039=CARTESIAN_POINT('Ctrl Pts',(0.151739500378994,0.0886778423193637,
8.01859528629505));
#25040=CARTESIAN_POINT('Ctrl Pts',(0.173228856734163,0.0296715164510714,
8.01489068994278));
#25041=CARTESIAN_POINT('Ctrl Pts',(0.1650135816391,-0.0248597287931786,
8.01118609359052));
#25042=CARTESIAN_POINT('Ctrl Pts',(0.156798306544038,-0.0793909740374281,
8.00748149723825));
#25043=CARTESIAN_POINT('Ctrl Pts',(0.118878399998744,-0.129447138657635,
8.00377690088598));
#25044=CARTESIAN_POINT('Ctrl Pts',(0.0686081222571477,-0.152119735080243,
8.00007230453371));
#25045=CARTESIAN_POINT('Ctrl Pts',(0.0183378445155504,-0.174792331502851,
7.99636770818144));
#25046=CARTESIAN_POINT('Ctrl Pts',(-0.0442828044223508,-0.17008135972786,
7.99266311182918));
#25047=CARTESIAN_POINT('Ctrl Pts',(-0.0905951294928038,-0.140142822695884,
7.98895851547691));
#25048=CARTESIAN_POINT('Ctrl Pts',(-0.136877296221191,-0.110223781481477,
7.98525633153827));
#25049=CARTESIAN_POINT('Ctrl Pts',(-0.166872371955659,-0.0551100204273624,
7.98155414759962));
#25050=CARTESIAN_POINT('Ctrl Pts',(-0.166875663578624,6.71114506779717E-7,
7.97785196366098));
#25051=CARTESIAN_POINT('Ctrl Pts',(-0.166584472654422,-0.000152342595601075,
7.99714803633902));
#25052=CARTESIAN_POINT('Ctrl Pts',(-0.16670733212153,-0.013647468998692,
7.99805048787021));
#25053=CARTESIAN_POINT('Ctrl Pts',(-0.165205039699776,-0.0271155902953411,
7.99895293940139));
#25054=CARTESIAN_POINT('Ctrl Pts',(-0.161972485922986,-0.0401547607711461,
7.99985539093257));
#25055=CARTESIAN_POINT('Ctrl Pts',(-0.148702735120651,-0.0936810297308429,
8.00355998728484));
#25056=CARTESIAN_POINT('Ctrl Pts',(-0.106275790398842,-0.139978909621527,
8.00726458363711));
#25057=CARTESIAN_POINT('Ctrl Pts',(-0.0541085835863948,-0.157859913185374,
8.01096917998938));
#25058=CARTESIAN_POINT('Ctrl Pts',(-0.00194137677394735,-0.17574091674922,
8.01467377634165));
#25059=CARTESIAN_POINT('Ctrl Pts',(0.0599660921291386,-0.165205043986227,
8.01837837269392));
#25060=CARTESIAN_POINT('Ctrl Pts',(0.10328151894002,-0.131074096808347,
8.02208296904618));
#25061=CARTESIAN_POINT('Ctrl Pts',(0.146596945750902,-0.0969431496304671,
8.02578756539845));
#25062=CARTESIAN_POINT('Ctrl Pts',(0.171320330469579,-0.0392171280376997,
8.02949216175071));
#25063=CARTESIAN_POINT('Ctrl Pts',(0.166136875888483,0.0156853268589705,
8.03319675810298));
#25064=CARTESIAN_POINT('Ctrl Pts',(0.160953421307388,0.0705877817556402,
8.03690135445525));
#25065=CARTESIAN_POINT('Ctrl Pts',(0.125863127426521,0.122666669956213,
8.04060595080752));
#25066=CARTESIAN_POINT('Ctrl Pts',(0.0769252662159289,0.14808779296844,
8.04431054715979));
#25067=CARTESIAN_POINT('Ctrl Pts',(0.0279874050053375,0.173508915980668,
8.04801514351206));
#25068=CARTESIAN_POINT('Ctrl Pts',(-0.0347980235349782,0.172272273804551,
8.05171973986432));
#25069=CARTESIAN_POINT('Ctrl Pts',(-0.0826969120159334,0.144943822744164,
8.05542433621659));
#25070=CARTESIAN_POINT('Ctrl Pts',(-0.13059580049689,0.117615371683777,
8.05912893256886));
#25071=CARTESIAN_POINT('Ctrl Pts',(-0.163608148918485,0.0641951117391189,
8.06283352892113));
#25072=CARTESIAN_POINT('Ctrl Pts',(-0.166625668832836,0.0091311277873714,
8.0665381252734));
#25073=CARTESIAN_POINT('Ctrl Pts',(-0.166791266612054,0.00610928411571916,
8.06674142896194));
#25074=CARTESIAN_POINT('Ctrl Pts',(-0.166866529586575,0.00308249007446834,
8.06694473265048));
#25075=CARTESIAN_POINT('Ctrl Pts',(-0.166853498321983,5.50350387731602E-5,
8.06714803633902));
#25076=CARTESIAN_POINT('Origin',(0.,0.,8.1));
#25077=CARTESIAN_POINT('',(-0.166421992115154,0.00011764607293073,8.13714803633902));
#25078=CARTESIAN_POINT('',(-0.1663714196928,-8.42509827993143E-5,8.11785196366098));
#25079=CARTESIAN_POINT('',(-0.1666,2.04026156737949E-17,8.1));
#25080=CARTESIAN_POINT('Ctrl Pts',(-0.1663714196928,-8.42509827993143E-5,
8.11785196366098));
#25081=CARTESIAN_POINT('Ctrl Pts',(-0.166219315065703,0.033129634461824,
8.1156380408079));
#25082=CARTESIAN_POINT('Ctrl Pts',(-0.156593011917271,0.0664247241004012,
8.11342411795482));
#25083=CARTESIAN_POINT('Ctrl Pts',(-0.138088887731799,0.0936960368738783,
8.11121019510175));
#25084=CARTESIAN_POINT('Ctrl Pts',(-0.107125608743007,0.139329607927122,
8.10750559874948));
#25085=CARTESIAN_POINT('Ctrl Pts',(-0.0513045000135449,0.168096650686574,
8.10380100239722));
#25086=CARTESIAN_POINT('Ctrl Pts',(0.00382759151932898,0.166831764913151,
8.10009640604495));
#25087=CARTESIAN_POINT('Ctrl Pts',(0.0589596830522032,0.165566879139728,
8.09639180969269));
#25088=CARTESIAN_POINT('Ctrl Pts',(0.113402757388489,0.134270064833428,
8.09268721334042));
#25089=CARTESIAN_POINT('Ctrl Pts',(0.142240632844969,0.0872644865265266,
8.08898261698814));
#25090=CARTESIAN_POINT('Ctrl Pts',(0.17107850830145,0.0402589082196249,
8.08527802063588));
#25091=CARTESIAN_POINT('Ctrl Pts',(0.174311184878124,-0.0224554340878791,
8.08157342428361));
#25092=CARTESIAN_POINT('Ctrl Pts',(0.15045920980913,-0.0721769660244263,
8.07786882793134));
#25093=CARTESIAN_POINT('Ctrl Pts',(0.126607234740136,-0.121898497960974,
8.07416423157907));
#25094=CARTESIAN_POINT('Ctrl Pts',(0.0756706080254739,-0.158627219526564,
8.07045963522681));
#25095=CARTESIAN_POINT('Ctrl Pts',(0.0209607657114752,-0.165554023030732,
8.06675503887454));
#25096=CARTESIAN_POINT('Ctrl Pts',(-0.0337490766025232,-0.1724808265349,
8.06305044252227));
#25097=CARTESIAN_POINT('Ctrl Pts',(-0.0922321345158577,-0.149605711977646,
8.05934584617));
#25098=CARTESIAN_POINT('Ctrl Pts',(-0.127723304953095,-0.107397605246734,
8.05564124981773));
#25099=CARTESIAN_POINT('Ctrl Pts',(-0.152597889234011,-0.0778153430873971,
8.05304482109881));
#25100=CARTESIAN_POINT('Ctrl Pts',(-0.166178529146176,-0.0387364383267161,
8.0504483923799));
#25101=CARTESIAN_POINT('Ctrl Pts',(-0.166495840369714,0.000142706802959736,
8.04785196366098));
#25102=CARTESIAN_POINT('Ctrl Pts',(-0.166853498321983,5.50350387731602E-5,
8.06714803633902));
#25103=CARTESIAN_POINT('Ctrl Pts',(-0.166629074104989,-0.05208374405736,
8.07064932900275));
#25104=CARTESIAN_POINT('Ctrl Pts',(-0.14021687013706,-0.10441857192293,
8.07415062166647));
#25105=CARTESIAN_POINT('Ctrl Pts',(-0.0980400613034392,-0.135039391987217,
8.0776519143302));
#25106=CARTESIAN_POINT('Ctrl Pts',(-0.0534142424525818,-0.167438219851223,
8.08135651068247));
#25107=CARTESIAN_POINT('Ctrl Pts',(0.0088600866562422,-0.175528167620399,
8.08506110703474));
#25108=CARTESIAN_POINT('Ctrl Pts',(0.060282726186914,-0.15560682482505,
8.08876570338701));
#25109=CARTESIAN_POINT('Ctrl Pts',(0.111705365717586,-0.1356854820297,8.09247029973928));
#25110=CARTESIAN_POINT('Ctrl Pts',(0.152276315670106,-0.0877528486698254,
8.09617489609155));
#25111=CARTESIAN_POINT('Ctrl Pts',(0.163428050745771,-0.033745566199093,
8.09987949244381));
#25112=CARTESIAN_POINT('Ctrl Pts',(0.174579785821436,0.0202617162716397,
8.10358408879608));
#25113=CARTESIAN_POINT('Ctrl Pts',(0.156312306020247,0.0803436478532293,
8.10728868514834));
#25114=CARTESIAN_POINT('Ctrl Pts',(0.116985827056872,0.119003391869641,
8.11099328150061));
#25115=CARTESIAN_POINT('Ctrl Pts',(0.077659348093497,0.157663135886053,
8.11469787785288));
#25116=CARTESIAN_POINT('Ctrl Pts',(0.0172738699679364,0.174900692337286,
8.11840247420515));
#25117=CARTESIAN_POINT('Ctrl Pts',(-0.0365348508466968,0.162827195769839,
8.12210707055742));
#25118=CARTESIAN_POINT('Ctrl Pts',(-0.0903435716613295,0.150753699202392,
8.12581166690969));
#25119=CARTESIAN_POINT('Ctrl Pts',(-0.137575535165035,0.109369149616266,
8.12951626326196));
#25120=CARTESIAN_POINT('Ctrl Pts',(-0.156614765436894,0.0576134207959084,
8.13322085961422));
#25121=CARTESIAN_POINT('Ctrl Pts',(-0.163342481933899,0.0393249781631264,
8.13452991852249));
#25122=CARTESIAN_POINT('Ctrl Pts',(-0.166549946273643,0.0197415505506192,
8.13583897743075));
#25123=CARTESIAN_POINT('Ctrl Pts',(-0.166421992115154,0.00011764607293073,
8.13714803633902));
#25124=CARTESIAN_POINT('Origin',(0.,0.,8.1));
#25125=CARTESIAN_POINT('',(-0.166428342743546,-0.000120644360202635,8.20714803633902));
#25126=CARTESIAN_POINT('',(-0.166803308618304,-9.74733517731731E-5,8.18785196366097));
#25127=CARTESIAN_POINT('',(-0.1666,2.04026156737949E-17,8.1));
#25128=CARTESIAN_POINT('Ctrl Pts',(-0.166803308618304,-9.74733517731731E-5,
8.18785196366097));
#25129=CARTESIAN_POINT('Ctrl Pts',(-0.166459413794316,0.0493761805259084,
8.18453228558818));
#25130=CARTESIAN_POINT('Ctrl Pts',(-0.143046299360482,0.0991325150909699,
8.18121260751538));
#25131=CARTESIAN_POINT('Ctrl Pts',(-0.104524315745128,0.130085186162334,
8.17789292944259));
#25132=CARTESIAN_POINT('Ctrl Pts',(-0.0615356894825779,0.164626834427408,
8.17418833309032));
#25133=CARTESIAN_POINT('Ctrl Pts',(0.000268698766544943,0.175751425299081,
8.17048373673804));
#25134=CARTESIAN_POINT('Ctrl Pts',(0.0526037202653142,0.15836772668421,
8.16677914038577));
#25135=CARTESIAN_POINT('Ctrl Pts',(0.104938741764083,0.14098402806934,8.1630745440335));
#25136=CARTESIAN_POINT('Ctrl Pts',(0.147804396512497,0.0950920399679271,
8.15936994768124));
#25137=CARTESIAN_POINT('Ctrl Pts',(0.161582974550151,0.0416944909598549,
8.15566535132897));
#25138=CARTESIAN_POINT('Ctrl Pts',(0.175361552587805,-0.0117030580482178,
8.1519607549767));
#25139=CARTESIAN_POINT('Ctrl Pts',(0.160053053914698,-0.0726061679629504,
8.14825615862444));
#25140=CARTESIAN_POINT('Ctrl Pts',(0.12266349975367,-0.113142185187744,
8.14455156227217));
#25141=CARTESIAN_POINT('Ctrl Pts',(0.085273945592641,-0.153678202412537,
8.1408469659199));
#25142=CARTESIAN_POINT('Ctrl Pts',(0.0258033359436895,-0.173847126947391,
8.13714236956763));
#25143=CARTESIAN_POINT('Ctrl Pts',(-0.0285312674660481,-0.16441853611335,
8.13343777321536));
#25144=CARTESIAN_POINT('Ctrl Pts',(-0.0828658708757854,-0.154989945279309,
8.12973317686309));
#25145=CARTESIAN_POINT('Ctrl Pts',(-0.132064468046309,-0.115963839076372,
8.12602858051083));
#25146=CARTESIAN_POINT('Ctrl Pts',(-0.15361104200751,-0.0652007363013865,
8.12232398415856));
#25147=CARTESIAN_POINT('Ctrl Pts',(-0.162281057239455,-0.0447744320976445,
8.12083331065937));
#25148=CARTESIAN_POINT('Ctrl Pts',(-0.166473834434309,-0.0224477487753186,
8.11934263716017));
#25149=CARTESIAN_POINT('Ctrl Pts',(-0.1663714196928,-8.42509827993143E-5,
8.11785196366098));
#25150=CARTESIAN_POINT('Ctrl Pts',(-0.166421992115154,0.00011764607293073,
8.13714803633902));
#25151=CARTESIAN_POINT('Ctrl Pts',(-0.16618783994993,-0.0357934941187008,
8.13954357378302));
#25152=CARTESIAN_POINT('Ctrl Pts',(-0.154784081132574,-0.0718401827168746,
8.14193911122702));
#25153=CARTESIAN_POINT('Ctrl Pts',(-0.133343409090461,-0.100334571613147,
8.14433464867103));
#25154=CARTESIAN_POINT('Ctrl Pts',(-0.100186325432156,-0.144399927147257,
8.1480392450233));
#25155=CARTESIAN_POINT('Ctrl Pts',(-0.0430256610755357,-0.170403730160887,
8.15174384137557));
#25156=CARTESIAN_POINT('Ctrl Pts',(0.0119786818135821,-0.166445192753257,
8.15544843772784));
#25157=CARTESIAN_POINT('Ctrl Pts',(0.0669830247027004,-0.162486655345627,
8.1591530340801));
#25158=CARTESIAN_POINT('Ctrl Pts',(0.119831046124316,-0.128565777516737,
8.16285763043236));
#25159=CARTESIAN_POINT('Ctrl Pts',(0.146336549406162,-0.0802066413494387,
8.16656222678463));
#25160=CARTESIAN_POINT('Ctrl Pts',(0.172842052688009,-0.0318475051821409,
8.1702668231369));
#25161=CARTESIAN_POINT('Ctrl Pts',(0.173005037830088,0.0309498893235645,
8.17397141948917));
#25162=CARTESIAN_POINT('Ctrl Pts',(0.146750913757937,0.0794459584866981,
8.17767601584144));
#25163=CARTESIAN_POINT('Ctrl Pts',(0.120496789685787,0.127942027649832,
8.18138061219371));
#25164=CARTESIAN_POINT('Ctrl Pts',(0.0678255563994073,0.162136771470394,
8.18508520854597));
#25165=CARTESIAN_POINT('Ctrl Pts',(0.0128425024785167,0.166380771541514,
8.18878980489824));
#25166=CARTESIAN_POINT('Ctrl Pts',(-0.0421405514423743,0.170624771612635,
8.19249440125051));
#25167=CARTESIAN_POINT('Ctrl Pts',(-0.0994354259977765,0.144918027934313,
8.19619899760278));
#25168=CARTESIAN_POINT('Ctrl Pts',(-0.132820796963375,0.101025377518093,
8.19990359395505));
#25169=CARTESIAN_POINT('Ctrl Pts',(-0.154582807668421,0.0724142732947816,
8.20231840808304));
#25170=CARTESIAN_POINT('Ctrl Pts',(-0.166185696135255,0.0360759969505965,
8.20473322221103));
#25171=CARTESIAN_POINT('Ctrl Pts',(-0.166428342743546,-0.000120644360202635,
8.20714803633902));
#25172=CARTESIAN_POINT('Origin',(0.,0.,8.1));
#25173=CARTESIAN_POINT('',(-0.166857329749817,-5.00571843092702E-5,8.27714803633902));
#25174=CARTESIAN_POINT('',(-0.166666727468001,0.000145874381161297,8.25785196366098));
#25175=CARTESIAN_POINT('',(-0.1666,2.04026156737949E-17,8.1));
#25176=CARTESIAN_POINT('Ctrl Pts',(-0.166666727468001,0.000145874381161297,
8.25785196366098));
#25177=CARTESIAN_POINT('Ctrl Pts',(-0.166765391649288,0.0109115262509472,
8.25713112672072));
#25178=CARTESIAN_POINT('Ctrl Pts',(-0.165811590519144,0.021659769778576,
8.25641028978047));
#25179=CARTESIAN_POINT('Ctrl Pts',(-0.163741809565622,0.0321886321711107,
8.25568945284021));
#25180=CARTESIAN_POINT('Ctrl Pts',(-0.153104586995315,0.0862996010110572,
8.25198485648794));
#25181=CARTESIAN_POINT('Ctrl Pts',(-0.11299166880269,0.134616189497655,
8.24828026013567));
#25182=CARTESIAN_POINT('Ctrl Pts',(-0.0617609594542789,0.155026036936271,
8.2445756637834));
#25183=CARTESIAN_POINT('Ctrl Pts',(-0.0105302501058676,0.175435884374887,
8.24087106743114));
#25184=CARTESIAN_POINT('Ctrl Pts',(0.05181825039833,0.16793899076552,8.23716647107887));
#25185=CARTESIAN_POINT('Ctrl Pts',(0.0967503972625045,0.135966351978801,
8.2334618747266));
#25186=CARTESIAN_POINT('Ctrl Pts',(0.141682544126679,0.103993713192083,
8.22975727837434));
#25187=CARTESIAN_POINT('Ctrl Pts',(0.16919833735083,0.0475453292280127,
8.22605268202206));
#25188=CARTESIAN_POINT('Ctrl Pts',(0.166705018140776,-0.0075448769081583,
8.2223480856698));
#25189=CARTESIAN_POINT('Ctrl Pts',(0.164211698930722,-0.0626350830443292,
8.21864348931753));
#25190=CARTESIAN_POINT('Ctrl Pts',(0.131709267286462,-0.116367111352601,
8.21493889296526));
#25191=CARTESIAN_POINT('Ctrl Pts',(0.0840726453513101,-0.144150194396363,
8.21123429661299));
#25192=CARTESIAN_POINT('Ctrl Pts',(0.0364360234161577,-0.171933277440126,
8.20752970026072));
#25193=CARTESIAN_POINT('Ctrl Pts',(-0.0263347888098876,-0.173767415219379,
8.20382510390846));
#25194=CARTESIAN_POINT('Ctrl Pts',(-0.0755123731768594,-0.148813204179182,
8.20012050755619));
#25195=CARTESIAN_POINT('Ctrl Pts',(-0.124689957543831,-0.123858993138985,
8.19641591120392));
#25196=CARTESIAN_POINT('Ctrl Pts',(-0.160274314051729,-0.0721164332793377,
8.19271131485164));
#25197=CARTESIAN_POINT('Ctrl Pts',(-0.16598006016769,-0.0172658005202765,
8.18900671849938));
#25198=CARTESIAN_POINT('Ctrl Pts',(-0.166572903697511,-0.0115666610778814,
8.18862180021991));
#25199=CARTESIAN_POINT('Ctrl Pts',(-0.166843183389611,-0.00583396746716338,
8.18823688194044));
#25200=CARTESIAN_POINT('Ctrl Pts',(-0.166803308618304,-9.74733517731731E-5,
8.18785196366097));
#25201=CARTESIAN_POINT('Ctrl Pts',(-0.166428342743546,-0.000120644360202635,
8.20714803633902));
#25202=CARTESIAN_POINT('Ctrl Pts',(-0.166557943311361,-0.0194537201444082,
8.2084378185633));
#25203=CARTESIAN_POINT('Ctrl Pts',(-0.163446738612952,-0.0387463908414866,
8.20972760078757));
#25204=CARTESIAN_POINT('Ctrl Pts',(-0.156911714654403,-0.0567996902533336,
8.21101738301185));
#25205=CARTESIAN_POINT('Ctrl Pts',(-0.138141394004038,-0.108653550454424,
8.21472197936412));
#25206=CARTESIAN_POINT('Ctrl Pts',(-0.0911248853275137,-0.150282713702488,
8.21842657571639));
#25207=CARTESIAN_POINT('Ctrl Pts',(-0.0373795604223798,-0.162635357383603,
8.22213117206866));
#25208=CARTESIAN_POINT('Ctrl Pts',(0.0163657644827538,-0.174988001064719,
8.22583576842093));
#25209=CARTESIAN_POINT('Ctrl Pts',(0.0768399056164966,-0.158064125178888,
8.22954036477319));
#25210=CARTESIAN_POINT('Ctrl Pts',(0.116366529377292,-0.119609037490229,
8.23324496112546));
#25211=CARTESIAN_POINT('Ctrl Pts',(0.155893153138087,-0.0811539498015699,
8.23694955747773));
#25212=CARTESIAN_POINT('Ctrl Pts',(0.174472259525936,-0.0211676503100823,
8.24065415383));
#25213=CARTESIAN_POINT('Ctrl Pts',(0.163601015151732,0.0328967908766299,
8.24435875018226));
#25214=CARTESIAN_POINT('Ctrl Pts',(0.152729770777529,0.0869612320633426,
8.24806334653453));
#25215=CARTESIAN_POINT('Ctrl Pts',(0.112408175641274,0.13510381494528,8.2517679428868));
#25216=CARTESIAN_POINT('Ctrl Pts',(0.0610896363960827,0.155291813479256,
8.25547253923907));
#25217=CARTESIAN_POINT('Ctrl Pts',(0.00977109715089173,0.175479812013233,
8.25917713559134));
#25218=CARTESIAN_POINT('Ctrl Pts',(-0.0525443862032349,0.167713226199247,
8.2628817319436));
#25219=CARTESIAN_POINT('Ctrl Pts',(-0.0973377793564846,0.135546478075116,
8.26658632829587));
#25220=CARTESIAN_POINT('Ctrl Pts',(-0.139906046427994,0.104977623416454,
8.27010689764359));
#25221=CARTESIAN_POINT('Ctrl Pts',(-0.166649815966412,0.052372567376715,
8.2736274669913));
#25222=CARTESIAN_POINT('Ctrl Pts',(-0.166857329749817,-5.00571843092702E-5,
8.27714803633902));
#25223=CARTESIAN_POINT('Origin',(0.,0.,8.1));
#25224=CARTESIAN_POINT('',(-0.166575830380064,0.000152189730136115,8.34714803633902));
#25225=CARTESIAN_POINT('',(-0.166329361973163,6.33250651713839E-6,8.32785196366098));
#25226=CARTESIAN_POINT('',(-0.1666,2.04026156737949E-17,8.1));
#25227=CARTESIAN_POINT('Ctrl Pts',(-0.166329361973163,6.33250651713839E-6,
8.32785196366098));
#25228=CARTESIAN_POINT('Ctrl Pts',(-0.16633865860321,0.0274266906163063,
8.326025371501));
#25229=CARTESIAN_POINT('Ctrl Pts',(-0.159934576682436,0.0548429606931825,
8.32419877934102));
#25230=CARTESIAN_POINT('Ctrl Pts',(-0.147093270055154,0.0788102667487975,
8.32237218718103));
#25231=CARTESIAN_POINT('Ctrl Pts',(-0.121049219975437,0.127419472751415,
8.31866759082877));
#25232=CARTESIAN_POINT('Ctrl Pts',(-0.0685264320130064,0.161841786350919,
8.3149629944765));
#25233=CARTESIAN_POINT('Ctrl Pts',(-0.013562257900901,0.166323640537549,
8.31125839812423));
#25234=CARTESIAN_POINT('Ctrl Pts',(0.0414019162112044,0.170805494724179,
8.30755380177196));
#25235=CARTESIAN_POINT('Ctrl Pts',(0.0988074764729849,0.145346889497936,
8.30384920541969));
#25236=CARTESIAN_POINT('Ctrl Pts',(0.132382442717744,0.10159909990231,8.30014460906742));
#25237=CARTESIAN_POINT('Ctrl Pts',(0.165957408962504,0.0578513103066831,
8.29644001271515));
#25238=CARTESIAN_POINT('Ctrl Pts',(0.175701781190243,-0.00418566365832695,
8.29273541636288));
#25239=CARTESIAN_POINT('Ctrl Pts',(0.157155992197206,-0.0561202490848672,
8.28903082001062));
#25240=CARTESIAN_POINT('Ctrl Pts',(0.138610203204169,-0.108054834511407,
8.28532622365835));
#25241=CARTESIAN_POINT('Ctrl Pts',(0.0917742529903561,-0.149887031399478,
8.28162162730609));
#25242=CARTESIAN_POINT('Ctrl Pts',(0.0380828797487078,-0.162472097638159,
8.27791703095382));
#25243=CARTESIAN_POINT('Ctrl Pts',(-0.0156084934929406,-0.175057163876841,
8.27421243460156));
#25244=CARTESIAN_POINT('Ctrl Pts',(-0.0761552897624244,-0.158395099466134,
8.27050783824928));
#25245=CARTESIAN_POINT('Ctrl Pts',(-0.115847924423172,-0.120111392664133,
8.26680324189701));
#25246=CARTESIAN_POINT('Ctrl Pts',(-0.147817202853201,-0.0892768942100117,
8.263819482485));
#25247=CARTESIAN_POINT('Ctrl Pts',(-0.166258326950347,-0.0444163744423642,
8.26083572307299));
#25248=CARTESIAN_POINT('Ctrl Pts',(-0.166666727468001,0.000145874381161297,
8.25785196366098));
#25249=CARTESIAN_POINT('Ctrl Pts',(-0.166857329749817,-5.00571843092702E-5,
8.27714803633902));
#25250=CARTESIAN_POINT('Ctrl Pts',(-0.166868176898728,-0.00279028969102808,
8.27733206334357));
#25251=CARTESIAN_POINT('Ctrl Pts',(-0.166806517545971,-0.00553002372997369,
8.27751609034812));
#25252=CARTESIAN_POINT('Ctrl Pts',(-0.166670821778591,-0.00826608591227963,
8.27770011735268));
#25253=CARTESIAN_POINT('Ctrl Pts',(-0.163939168095075,-0.0633449913412659,
8.28140471370495));
#25254=CARTESIAN_POINT('Ctrl Pts',(-0.131204557775671,-0.116935891764961,
8.28510931005722));
#25255=CARTESIAN_POINT('Ctrl Pts',(-0.0834481708510229,-0.144512607721388,
8.28881390640949));
#25256=CARTESIAN_POINT('Ctrl Pts',(-0.0356917839263749,-0.172089323677816,
8.29251850276175));
#25257=CARTESIAN_POINT('Ctrl Pts',(0.0270863796035167,-0.173651855166976,
8.29622309911402));
#25258=CARTESIAN_POINT('Ctrl Pts',(0.0761555372230057,-0.148485100796662,
8.29992769546628));
#25259=CARTESIAN_POINT('Ctrl Pts',(0.125224694842494,-0.123318346426348,
8.30363229181855));
#25260=CARTESIAN_POINT('Ctrl Pts',(0.160584846551581,-0.0714223061965609,
8.30733688817082));
#25261=CARTESIAN_POINT('Ctrl Pts',(0.166053218414492,-0.016547497181162,
8.31104148452309));
#25262=CARTESIAN_POINT('Ctrl Pts',(0.171521590277403,0.0383273118342368,
8.31474608087536));
#25263=CARTESIAN_POINT('Ctrl Pts',(0.14709818229414,0.0961808896352466,
8.31845067722763));
#25264=CARTESIAN_POINT('Ctrl Pts',(0.103960505619201,0.130536218273543,
8.3221552735799));
#25265=CARTESIAN_POINT('Ctrl Pts',(0.0608228289442621,0.164891546911839,
8.32585986993216));
#25266=CARTESIAN_POINT('Ctrl Pts',(-0.00102911642235214,0.175748626387421,
8.32956446628443));
#25267=CARTESIAN_POINT('Ctrl Pts',(-0.0532884369608459,0.158138652745392,
8.3332690626367));
#25268=CARTESIAN_POINT('Ctrl Pts',(-0.105547757499339,0.140528679103364,
8.33697365898897));
#25269=CARTESIAN_POINT('Ctrl Pts',(-0.148214453209713,0.0944516523437251,
8.34067825534123));
#25270=CARTESIAN_POINT('Ctrl Pts',(-0.16176186886028,0.0409949849761845,
8.3443828516935));
#25271=CARTESIAN_POINT('Ctrl Pts',(-0.165132555990647,0.027694610544955,
8.34530457990867));
#25272=CARTESIAN_POINT('Ctrl Pts',(-0.166700621367384,0.0139374013064621,
8.34622630812385));
#25273=CARTESIAN_POINT('Ctrl Pts',(-0.166575830380064,0.000152189730136115,
8.34714803633902));
#25274=CARTESIAN_POINT('Origin',(0.,0.,8.1));
#25275=CARTESIAN_POINT('',(-0.166339236432839,-4.26122283673641E-5,8.41714803633902));
#25276=CARTESIAN_POINT('',(-0.166643482566988,-0.000149162233397024,8.39785196366098));
#25277=CARTESIAN_POINT('',(-0.1666,2.04026156737949E-17,8.1));
#25278=CARTESIAN_POINT('Ctrl Pts',(-0.166643482566988,-0.000149162233397024,
8.39785196366098));
#25279=CARTESIAN_POINT('Ctrl Pts',(-0.166239168982283,0.043660968966674,
8.39491961628127));
#25280=CARTESIAN_POINT('Ctrl Pts',(-0.148495522651441,0.0877608658755926,
8.39198726890156));
#25281=CARTESIAN_POINT('Ctrl Pts',(-0.117499615731863,0.118496111839818,
8.38905492152186));
#25282=CARTESIAN_POINT('Ctrl Pts',(-0.0783407751033059,0.157325645091268,
8.38535032516959));
#25283=CARTESIAN_POINT('Ctrl Pts',(-0.0180304466584345,0.17482430805586,
8.38164572881733));
#25284=CARTESIAN_POINT('Ctrl Pts',(0.0358300059551043,0.162983738211835,
8.37794113246506));
#25285=CARTESIAN_POINT('Ctrl Pts',(0.0896904585686423,0.151143168367811,
8.37423653611279));
#25286=CARTESIAN_POINT('Ctrl Pts',(0.137101035350848,0.109963365715171,
8.37053193976051));
#25287=CARTESIAN_POINT('Ctrl Pts',(0.15636401692648,0.0582905005399897,
8.36682734340825));
#25288=CARTESIAN_POINT('Ctrl Pts',(0.175626998502113,0.00661763536480815,
8.36312274705598));
#25289=CARTESIAN_POINT('Ctrl Pts',(0.166742384871172,-0.0555482923329149,
8.35941815070372));
#25290=CARTESIAN_POINT('Ctrl Pts',(0.133776269878663,-0.0997566932863041,
8.35571355435145));
#25291=CARTESIAN_POINT('Ctrl Pts',(0.100810154886153,-0.143965094239693,
8.35200895799918));
#25292=CARTESIAN_POINT('Ctrl Pts',(0.043762538532075,-0.170215968448749,
8.34830436164691));
#25293=CARTESIAN_POINT('Ctrl Pts',(-0.0112584140961097,-0.166495454454524,
8.34459976529464));
#25294=CARTESIAN_POINT('Ctrl Pts',(-0.0662793667242941,-0.162774940460298,
8.34089516894237));
#25295=CARTESIAN_POINT('Ctrl Pts',(-0.119273655626585,-0.129083038262791,
8.3371905725901));
#25296=CARTESIAN_POINT('Ctrl Pts',(-0.145988143979229,-0.080839037961172,
8.33348597623784));
#25297=CARTESIAN_POINT('Ctrl Pts',(-0.159530758707101,-0.0563822750094863,
8.33160797204555));
#25298=CARTESIAN_POINT('Ctrl Pts',(-0.166319803676251,-0.0281858105522191,
8.32972996785327));
#25299=CARTESIAN_POINT('Ctrl Pts',(-0.166329361973163,6.33250651713839E-6,
8.32785196366098));
#25300=CARTESIAN_POINT('Ctrl Pts',(-0.166575830380064,0.000152189730136115,
8.34714803633902));
#25301=CARTESIAN_POINT('Ctrl Pts',(-0.16619906328463,-0.0414679163135104,
8.34993090447612));
#25302=CARTESIAN_POINT('Ctrl Pts',(-0.150391099631022,-0.0833432770783291,
8.35271377261321));
#25303=CARTESIAN_POINT('Ctrl Pts',(-0.122172827684305,-0.113671857518162,
8.35549664075031));
#25304=CARTESIAN_POINT('Ctrl Pts',(-0.0846082352669996,-0.154045724669524,
8.35920123710257));
#25305=CARTESIAN_POINT('Ctrl Pts',(-0.0250509148416262,-0.173957150996807,
8.36290583345484));
#25306=CARTESIAN_POINT('Ctrl Pts',(0.0292423881988082,-0.164293559577237,
8.36661042980711));
#25307=CARTESIAN_POINT('Ctrl Pts',(0.0835356912392426,-0.154629968157667,
8.37031502615938));
#25308=CARTESIAN_POINT('Ctrl Pts',(0.132564976894738,-0.115391358991245,
8.37401962251165));
#25309=CARTESIAN_POINT('Ctrl Pts',(0.153891714545025,-0.064535503582266,
8.37772421886392));
#25310=CARTESIAN_POINT('Ctrl Pts',(0.175218452195312,-0.0136796481732867,
8.38142881521619));
#25311=CARTESIAN_POINT('Ctrl Pts',(0.168842641840389,0.0487934534782495,
8.38513341156845));
#25312=CARTESIAN_POINT('Ctrl Pts',(0.137682209292225,0.0942926312053136,
8.38883800792072));
#25313=CARTESIAN_POINT('Ctrl Pts',(0.106521776744061,0.139791808932377,
8.39254260427298));
#25314=CARTESIAN_POINT('Ctrl Pts',(0.0505767220026555,0.168317062734969,
8.39624720062525));
#25315=CARTESIAN_POINT('Ctrl Pts',(-0.0045493834981962,0.166813650344707,
8.39995179697752));
#25316=CARTESIAN_POINT('Ctrl Pts',(-0.0596754889990479,0.165310237954446,
8.40365639332979));
#25317=CARTESIAN_POINT('Ctrl Pts',(-0.113982645259346,0.133778159371331,
8.40736098968206));
#25318=CARTESIAN_POINT('Ctrl Pts',(-0.142616874078383,0.0866482454219461,
8.41106558603433));
#25319=CARTESIAN_POINT('Ctrl Pts',(-0.158288061727777,0.0608545797336438,
8.41309306946923));
#25320=CARTESIAN_POINT('Ctrl Pts',(-0.166269569984901,0.0303889749587513,
8.41512055290413));
#25321=CARTESIAN_POINT('Ctrl Pts',(-0.166339236432839,-4.26122283673641E-5,
8.41714803633902));
#25322=CARTESIAN_POINT('Origin',(0.,0.,8.1));
#25323=CARTESIAN_POINT('',(-0.166732044643443,-0.000130047968060085,8.48714803633902));
#25324=CARTESIAN_POINT('',(-0.16681984310415,8.64016909114964E-5,8.46785196366098));
#25325=CARTESIAN_POINT('',(-0.1666,2.04026156737949E-17,8.1));
#25326=CARTESIAN_POINT('Ctrl Pts',(-0.16681984310415,8.64016909114964E-5,
8.46785196366098));
#25327=CARTESIAN_POINT('Ctrl Pts',(-0.166851207378176,0.00505539796551705,
8.46751845741382));
#25328=CARTESIAN_POINT('Ctrl Pts',(-0.166648433574087,0.010021798785139,
8.46718495116665));
#25329=CARTESIAN_POINT('Ctrl Pts',(-0.166203182979447,0.0149663647710484,
8.46685144491949));
#25330=CARTESIAN_POINT('Ctrl Pts',(-0.161257327413684,0.0698907365654406,
8.46314684856722));
#25331=CARTESIAN_POINT('Ctrl Pts',(-0.126392682383394,0.122120946203704,
8.45944225221496));
#25332=CARTESIAN_POINT('Ctrl Pts',(-0.0775652682414317,0.147753565233456,
8.45573765586268));
#25333=CARTESIAN_POINT('Ctrl Pts',(-0.0287378540994696,0.173386184263208,
8.45203305951042));
#25334=CARTESIAN_POINT('Ctrl Pts',(0.0340523291541647,0.172421212684449,
8.44832846315814));
#25335=CARTESIAN_POINT('Ctrl Pts',(0.0820690071135884,0.145300263537307,
8.44462386680588));
#25336=CARTESIAN_POINT('Ctrl Pts',(0.130085685073012,0.118179314390165,
8.44091927045361));
#25337=CARTESIAN_POINT('Ctrl Pts',(0.163328857738225,0.0649023876746406,
8.43721467410134));
#25338=CARTESIAN_POINT('Ctrl Pts',(0.166584594097058,0.00985197688937799,
8.43351007774908));
#25339=CARTESIAN_POINT('Ctrl Pts',(0.16984033045589,-0.045198433895885,
8.42980548139681));
#25340=CARTESIAN_POINT('Ctrl Pts',(0.143108630508342,-0.102022328750885,
8.42610088504454));
#25341=CARTESIAN_POINT('Ctrl Pts',(0.0986234106037675,-0.134613932949943,
8.42239628869227));
#25342=CARTESIAN_POINT('Ctrl Pts',(0.0541381906991934,-0.167205537149,8.41869169234));
#25343=CARTESIAN_POINT('Ctrl Pts',(-0.0081005491624063,-0.175564850692113,
8.41498709598773));
#25344=CARTESIAN_POINT('Ctrl Pts',(-0.059608897920023,-0.155866184839173,
8.41128249963547));
#25345=CARTESIAN_POINT('Ctrl Pts',(-0.11111724667764,-0.136167518986233,
8.4075779032832));
#25346=CARTESIAN_POINT('Ctrl Pts',(-0.151895204331274,-0.0884108737372401,
8.40387330693093));
#25347=CARTESIAN_POINT('Ctrl Pts',(-0.163280506751969,-0.0344523493435898,
8.40016871057866));
#25348=CARTESIAN_POINT('Ctrl Pts',(-0.165653852525874,-0.0232043182326152,
8.3993964616061));
#25349=CARTESIAN_POINT('Ctrl Pts',(-0.16674996065773,-0.0116867887237509,
8.39862421263354));
#25350=CARTESIAN_POINT('Ctrl Pts',(-0.166643482566988,-0.000149162233397024,
8.39785196366098));
#25351=CARTESIAN_POINT('Ctrl Pts',(-0.166339236432839,-4.26122283673641E-5,
8.41714803633902));
#25352=CARTESIAN_POINT('Ctrl Pts',(-0.166396863783936,-0.0252153002460154,
8.41882514925639));
#25353=CARTESIAN_POINT('Ctrl Pts',(-0.161040873551955,-0.0503647119879558,
8.42050226217376));
#25354=CARTESIAN_POINT('Ctrl Pts',(-0.150145522232543,-0.0728272849498228,
8.42217937509113));
#25355=CARTESIAN_POINT('Ctrl Pts',(-0.126078640189889,-0.122445152056552,
8.4258839714434));
#25356=CARTESIAN_POINT('Ctrl Pts',(-0.0749835747268059,-0.158953136954354,
8.42958856779567));
#25357=CARTESIAN_POINT('Ctrl Pts',(-0.0202442715114259,-0.165643168038739,
8.43329316414793));
#25358=CARTESIAN_POINT('Ctrl Pts',(0.0344950317039542,-0.172333199123123,
8.4369977605002));
#25359=CARTESIAN_POINT('Ctrl Pts',(0.0928785726716311,-0.149205276394089,
8.44070235685247));
#25360=CARTESIAN_POINT('Ctrl Pts',(0.128186791283717,-0.106843995678858,
8.44440695320474));
#25361=CARTESIAN_POINT('Ctrl Pts',(0.163495009895803,-0.0644827149636277,
8.44811154955701));
#25362=CARTESIAN_POINT('Ctrl Pts',(0.175727906152299,-0.00288807626219958,
8.45181614590928));
#25363=CARTESIAN_POINT('Ctrl Pts',(0.159287028744638,0.0497507269318684,
8.45552074226155));
#25364=CARTESIAN_POINT('Ctrl Pts',(0.142846151336978,0.102389530125936,
8.45922533861382));
#25365=CARTESIAN_POINT('Ctrl Pts',(0.0977315002651613,0.146072497812644,
8.46292993496608));
#25366=CARTESIAN_POINT('Ctrl Pts',(0.0445900454027681,0.160807986828964,
8.46663453131835));
#25367=CARTESIAN_POINT('Ctrl Pts',(-0.00855140945962513,0.175543475845283,
8.47033912767062));
#25368=CARTESIAN_POINT('Ctrl Pts',(-0.0697196681125948,0.161331486191215,
8.47404372402289));
#25369=CARTESIAN_POINT('Ctrl Pts',(-0.110920718221372,0.124675988017335,
8.47774832037516));
#25370=CARTESIAN_POINT('Ctrl Pts',(-0.145767354814535,0.0936738455808142,
8.48088155902978));
#25371=CARTESIAN_POINT('Ctrl Pts',(-0.166330890122557,0.0466172354067069,
8.4840147976844));
#25372=CARTESIAN_POINT('Ctrl Pts',(-0.166732044643443,-0.000130047968060085,
8.48714803633902));
#25373=CARTESIAN_POINT('Origin',(0.,0.,8.1));
#25374=CARTESIAN_POINT('',(-0.166747144031447,0.000121296159821427,8.55714803633902));
#25375=CARTESIAN_POINT('',(-0.166383640089184,9.41837290711752E-5,8.53785196366098));
#25376=CARTESIAN_POINT('',(-0.1666,2.04026156737949E-17,8.1));
#25377=CARTESIAN_POINT('',(0.126907087985233,0.107935865304857,8.6));
#25378=CARTESIAN_POINT('Ctrl Pts',(-0.166747144031447,0.000121296159821427,
8.55714803633902));
#25379=CARTESIAN_POINT('Ctrl Pts',(-0.16635329561639,-0.0471552430000254,
8.56031823516921));
#25380=CARTESIAN_POINT('Ctrl Pts',(-0.14524398945692,-0.0947301254344308,
8.5634884339994));
#25381=CARTESIAN_POINT('Ctrl Pts',(-0.109675246818716,-0.12575848265665,
8.56665863282959));
#25382=CARTESIAN_POINT('Ctrl Pts',(-0.0681107137120021,-0.162017261723657,
8.57036322918185));
#25383=CARTESIAN_POINT('Ctrl Pts',(-0.00680104346501744,-0.175680871885562,
8.57406782553412));
#25384=CARTESIAN_POINT('Ctrl Pts',(0.0461904511917562,-0.160385037585203,
8.57777242188639));
#25385=CARTESIAN_POINT('Ctrl Pts',(0.0991819458485301,-0.145089203284843,
8.58147701823866));
#25386=CARTESIAN_POINT('Ctrl Pts',(0.143855264915093,-0.10083392452222,
8.58518161459093));
#25387=CARTESIAN_POINT('Ctrl Pts',(0.159759361228124,-0.0481275638750195,
8.5888862109432));
#25388=CARTESIAN_POINT('Ctrl Pts',(0.175663457541156,0.00457879677218119,
8.59259080729547));
#25389=CARTESIAN_POINT('Ctrl Pts',(0.162798331100656,0.0657362393039593,
8.59629540364773));
#25390=CARTESIAN_POINT('Ctrl Pts',(0.126907087985233,0.107935865304858,
8.6));
#25391=CARTESIAN_POINT('',(-0.127146846929917,0.108121031306322,8.59999999999999));
#25392=CARTESIAN_POINT('Origin',(0.,0.,8.6));
#25393=CARTESIAN_POINT('Ctrl Pts',(-0.127146980098748,0.108121134152685,
8.6));
#25394=CARTESIAN_POINT('Ctrl Pts',(-0.0920609617982474,0.149274297422621,
8.59636770818144));
#25395=CARTESIAN_POINT('Ctrl Pts',(-0.0350637580639813,0.171876538765403,
8.59273541636288));
#25396=CARTESIAN_POINT('Ctrl Pts',(0.0186762172371964,0.165816310153089,
8.58910312454433));
#25397=CARTESIAN_POINT('Ctrl Pts',(0.0734859424511011,0.159635446408496,
8.58539852819206));
#25398=CARTESIAN_POINT('Ctrl Pts',(0.124907471537698,0.123639642847462,
8.5816939318398));
#25399=CARTESIAN_POINT('Ctrl Pts',(0.149440861098049,0.0742590945192524,
8.57798933548753));
#25400=CARTESIAN_POINT('Ctrl Pts',(0.173974250658401,0.0248785461910427,
8.57428473913527));
#25401=CARTESIAN_POINT('Ctrl Pts',(0.171619500692506,-0.0378867469043425,
8.57058014278299));
#25402=CARTESIAN_POINT('Ctrl Pts',(0.143437456560707,-0.0852900722270229,
8.56687554643073));
#25403=CARTESIAN_POINT('Ctrl Pts',(0.115255412428908,-0.132693397549703,
8.56317095007846));
#25404=CARTESIAN_POINT('Ctrl Pts',(0.0612460741312054,-0.164734755099679,
8.55946635372619));
#25405=CARTESIAN_POINT('Ctrl Pts',(0.00613559996277483,-0.166761229307977,
8.55576175737392));
#25406=CARTESIAN_POINT('Ctrl Pts',(-0.0489748742056557,-0.168787703516275,
8.55205716102165));
#25407=CARTESIAN_POINT('Ctrl Pts',(-0.105186484244814,-0.140799294382895,
8.54835256466938));
#25408=CARTESIAN_POINT('Ctrl Pts',(-0.136777942839038,-0.0955995137046261,
8.54464796831711));
#25409=CARTESIAN_POINT('Ctrl Pts',(-0.1560958998925,-0.0679601624108457,
8.54238263343174));
#25410=CARTESIAN_POINT('Ctrl Pts',(-0.166207797888661,-0.033885070733673,
8.54011729854636));
#25411=CARTESIAN_POINT('Ctrl Pts',(-0.166383640089184,9.41837290711752E-5,
8.53785196366098));
#25412=CARTESIAN_POINT('Origin',(0.,0.,8.75459252805377));
#25413=CARTESIAN_POINT('',(-0.205721525535574,0.000119487981252803,7.74540747194623));
#25414=CARTESIAN_POINT('',(-0.205159724654165,-8.03386490614408E-5,7.73959252805377));
#25415=CARTESIAN_POINT('',(-0.205475,1.36055398187253E-14,8.75459252805377));
#25416=CARTESIAN_POINT('',(0.18826275096637,-0.0823232180103198,7.7));
#25417=CARTESIAN_POINT('Ctrl Pts',(-0.205159724654165,-8.03386490614358E-5,
7.73959252805377));
#25418=CARTESIAN_POINT('Ctrl Pts',(-0.205041512904561,0.0384791939730818,
7.73750880775931));
#25419=CARTESIAN_POINT('Ctrl Pts',(-0.176055839029368,0.14576176638949,
7.7317204911126));
#25420=CARTESIAN_POINT('Ctrl Pts',(-0.00298040876483471,0.242992688549725,
7.7222275781136));
#25421=CARTESIAN_POINT('Ctrl Pts',(0.202514421274951,0.133877006738626,
7.7111137890568));
#25422=CARTESIAN_POINT('Ctrl Pts',(0.215637179506012,-0.0197213743559677,
7.70370459635227));
#25423=CARTESIAN_POINT('Ctrl Pts',(0.188262750966369,-0.0823232180103224,
7.7));
#25424=CARTESIAN_POINT('',(0.122359307443305,-0.165534545134462,7.7));
#25425=CARTESIAN_POINT('Origin',(0.,0.,7.7));
#25426=CARTESIAN_POINT('Ctrl Pts',(-0.205721525535573,0.000119487981252853,
7.74540747194623));
#25427=CARTESIAN_POINT('Ctrl Pts',(-0.205771798324789,0.00728349121284206,
7.74501772883951));
#25428=CARTESIAN_POINT('Ctrl Pts',(-0.202182676839297,0.0824925534713558,
7.74092338938052));
#25429=CARTESIAN_POINT('Ctrl Pts',(-0.109630632113431,0.216732284629596,
7.73312445356927));
#25430=CARTESIAN_POINT('Ctrl Pts',(0.122656937311001,0.209606344739839,
7.72201066451247));
#25431=CARTESIAN_POINT('Ctrl Pts',(0.241793562216327,0.0120091699547426,
7.71096917998937));
#25432=CARTESIAN_POINT('Ctrl Pts',(0.175945028483479,-0.125819303453627,
7.70363229181856));
#25433=CARTESIAN_POINT('Ctrl Pts',(0.122359422806364,-0.165534717635809,
7.7));
#25434=CARTESIAN_POINT('Origin',(0.,0.,8.75459252805377));
#25435=CARTESIAN_POINT('',(-0.205191698097627,0.000102651616370908,7.81540747194623));
#25436=CARTESIAN_POINT('',(-0.205666299785903,-0.000149771831496819,7.80959252805377));
#25437=CARTESIAN_POINT('',(-0.205475,1.36055398187253E-14,8.75459252805377));
#25438=CARTESIAN_POINT('Ctrl Pts',(-0.205666299785903,-0.000149771831496818,
7.80959252805377));
#25439=CARTESIAN_POINT('Ctrl Pts',(-0.205185187897512,0.0585192076367542,
7.80640305253959));
#25440=CARTESIAN_POINT('Ctrl Pts',(-0.148137553353403,0.186149387791063,
7.79950898067314));
#25441=CARTESIAN_POINT('Ctrl Pts',(0.0684305468563471,0.233026651290108,
7.78891031245443));
#25442=CARTESIAN_POINT('Ctrl Pts',(0.232891204484732,0.0688818314302299,
7.77779652339763));
#25443=CARTESIAN_POINT('Ctrl Pts',(0.184179773794582,-0.158294460538047,
7.76668273434082));
#25444=CARTESIAN_POINT('Ctrl Pts',(-0.0331053048843776,-0.240615458747729,
7.75556894528403));
#25445=CARTESIAN_POINT('Ctrl Pts',(-0.18504446938345,-0.128502550435188,
7.74653887652167));
#25446=CARTESIAN_POINT('Ctrl Pts',(-0.205251678739939,-0.0300748745732145,
7.74121340411158));
#25447=CARTESIAN_POINT('Ctrl Pts',(-0.205159724654165,-8.03386490614358E-5,
7.73959252805377));
#25448=CARTESIAN_POINT('Ctrl Pts',(-0.205191698097627,0.000102651616370887,
7.81540747194623));
#25449=CARTESIAN_POINT('Ctrl Pts',(-0.205316860451277,0.0277742455172506,
7.81391197361979));
#25450=CARTESIAN_POINT('Ctrl Pts',(-0.187215293273578,0.12383601283077,
7.80871187894108));
#25451=CARTESIAN_POINT('Ctrl Pts',(-0.0412126180342513,0.239342358997698,
7.7998071879101));
#25452=CARTESIAN_POINT('Ctrl Pts',(0.178733982604362,0.164430288641772,
7.7886933988533));
#25453=CARTESIAN_POINT('Ctrl Pts',(0.23508167636479,-0.0609852135282689,
7.77757960979648));
#25454=CARTESIAN_POINT('Ctrl Pts',(0.0762597491160078,-0.230583185734543,
7.76646582073969));
#25455=CARTESIAN_POINT('Ctrl Pts',(-0.14435245202745,-0.190573997415322,
7.75574177478959));
#25456=CARTESIAN_POINT('Ctrl Pts',(-0.205293944096357,-0.060811979321282,
7.74872232519178));
#25457=CARTESIAN_POINT('Ctrl Pts',(-0.205721525535573,0.000119487981252853,
7.74540747194623));
#25458=CARTESIAN_POINT('Origin',(0.,0.,8.75459252805377));
#25459=CARTESIAN_POINT('',(-0.205348950198108,-0.000176526842551344,7.88540747194623));
#25460=CARTESIAN_POINT('',(-0.205627835809057,0.000163389939152625,7.87959252805377));
#25461=CARTESIAN_POINT('',(-0.205475,1.36055398187253E-14,8.75459252805377));
#25462=CARTESIAN_POINT('Ctrl Pts',(-0.205627835809057,0.000163389939152636,
7.87959252805377));
#25463=CARTESIAN_POINT('Ctrl Pts',(-0.205722307155807,0.0110331713473729,
7.87900189367214));
#25464=CARTESIAN_POINT('Ctrl Pts',(-0.199995231038606,0.0899810208205928,
7.87470666293823));
#25465=CARTESIAN_POINT('Ctrl Pts',(-0.0977380548679695,0.222329472572989,
7.86670683585206));
#25466=CARTESIAN_POINT('Ctrl Pts',(0.133783834178758,0.2026944262293,7.85559304679526));
#25467=CARTESIAN_POINT('Ctrl Pts',(0.242851896763891,-0.00246926665421919,
7.84447925773846));
#25468=CARTESIAN_POINT('Ctrl Pts',(0.129634796329349,-0.205372535067366,
7.83336546868165));
#25469=CARTESIAN_POINT('Ctrl Pts',(-0.102238368895662,-0.220296541877889,
7.82225167962484));
#25470=CARTESIAN_POINT('Ctrl Pts',(-0.200843893701057,-0.0871642606221136,
7.81432736608222));
#25471=CARTESIAN_POINT('Ctrl Pts',(-0.20574400245459,-0.00962518988669528,
7.81010764889186));
#25472=CARTESIAN_POINT('Ctrl Pts',(-0.205666299785903,-0.000149771831496818,
7.80959252805377));
#25473=CARTESIAN_POINT('Ctrl Pts',(-0.205348950198108,-0.00017652684255136,
7.88540747194623));
#25474=CARTESIAN_POINT('Ctrl Pts',(-0.204955372010552,0.047862483759944,
7.88280621840006));
#25475=CARTESIAN_POINT('Ctrl Pts',(-0.164187007775315,0.164918452985973,
7.87650036850162));
#25476=CARTESIAN_POINT('Ctrl Pts',(0.0308184982090563,0.240901114896414,
7.86648992225093));
#25477=CARTESIAN_POINT('Ctrl Pts',(0.21910883681408,0.104758985980235,7.85537613319412));
#25478=CARTESIAN_POINT('Ctrl Pts',(0.206846344849442,-0.12727020659438,
7.84426234413731));
#25479=CARTESIAN_POINT('Ctrl Pts',(0.00525510193017616,-0.242807583839013,
7.83314855508051));
#25480=CARTESIAN_POINT('Ctrl Pts',(-0.173372430949953,-0.150459116557522,
7.82353026435015));
#25481=CARTESIAN_POINT('Ctrl Pts',(-0.205006812629375,-0.0407728628372422,
7.81761656997206));
#25482=CARTESIAN_POINT('Ctrl Pts',(-0.205191698097627,0.000102651616370887,
7.81540747194623));
#25483=CARTESIAN_POINT('Origin',(0.,0.,8.75459252805377));
#25484=CARTESIAN_POINT('',(-0.205814989538108,8.27718761863166E-7,7.95540747194623));
#25485=CARTESIAN_POINT('',(-0.205150812725382,4.68974045001175E-5,7.94959252805377));
#25486=CARTESIAN_POINT('',(-0.205475,1.36055398187253E-14,8.75459252805377));
#25487=CARTESIAN_POINT('Ctrl Pts',(-0.205150812725382,4.6897404500125E-5,
7.94959252805377));
#25488=CARTESIAN_POINT('Ctrl Pts',(-0.205214921684749,0.0314512961965735,
7.94789613845241));
#25489=CARTESIAN_POINT('Ctrl Pts',(-0.183675662640219,0.131353623293904,
7.94249515249879));
#25490=CARTESIAN_POINT('Ctrl Pts',(-0.0282109883268786,0.241220379359275,
7.93338957019289));
#25491=CARTESIAN_POINT('Ctrl Pts',(0.187362754755622,0.154526145718984,
7.92227578113608));
#25492=CARTESIAN_POINT('Ctrl Pts',(0.23144124413335,-0.0736076238344533,
7.91116199207928));
#25493=CARTESIAN_POINT('Ctrl Pts',(0.0636789369204538,-0.234367495981061,
7.90004820302247));
#25494=CARTESIAN_POINT('Ctrl Pts',(-0.150356242673218,-0.183465152197969,
7.8895250483473));
#25495=CARTESIAN_POINT('Ctrl Pts',(-0.205129760874308,-0.057144628332151,
7.8827064900244));
#25496=CARTESIAN_POINT('Ctrl Pts',(-0.205627835809057,0.000163389939152636,
7.87959252805377));
#25497=CARTESIAN_POINT('Ctrl Pts',(-0.205814987838042,8.27714623007834E-7,
7.95540747194623));
#25498=CARTESIAN_POINT('Ctrl Pts',(-0.205814990483421,4.51185256548844E-5,
7.9554050595326));
#25499=CARTESIAN_POINT('Ctrl Pts',(-0.205794920564842,0.0681041019067216,
7.95169805076671));
#25500=CARTESIAN_POINT('Ctrl Pts',(-0.131583562478442,0.204129595218713,
7.94428644564855));
#25501=CARTESIAN_POINT('Ctrl Pts',(0.100137168795687,0.221259289107705,
7.93317265659175));
#25502=CARTESIAN_POINT('Ctrl Pts',(0.240201214065173,0.035867846224428,
7.92205886753494));
#25503=CARTESIAN_POINT('Ctrl Pts',(0.160406363583993,-0.182353842678505,
7.91094507847815));
#25504=CARTESIAN_POINT('Ctrl Pts',(-0.0662102497254891,-0.233664992135114,
7.89983128942133));
#25505=CARTESIAN_POINT('Ctrl Pts',(-0.19336732015938,-0.109149318984397,
7.8913187539107));
#25506=CARTESIAN_POINT('Ctrl Pts',(-0.205515889581051,-0.0205526631244362,
7.88651081475233));
#25507=CARTESIAN_POINT('Ctrl Pts',(-0.205348950198108,-0.00017652684255136,
7.88540747194623));
#25508=CARTESIAN_POINT('Origin',(0.,0.,8.75459252805377));
#25509=CARTESIAN_POINT('',(-0.205346535413967,0.000176006484619851,8.02540747194623));
#25510=CARTESIAN_POINT('',(-0.205455849451785,-0.000187890725276845,8.01959252805377));
#25511=CARTESIAN_POINT('',(-0.205475,1.36055398187253E-14,8.75459252805377));
#25512=CARTESIAN_POINT('Ctrl Pts',(-0.205455849451785,-0.000187890725276842,
8.01959252805376));
#25513=CARTESIAN_POINT('Ctrl Pts',(-0.204985349796021,0.0514927202738006,
8.01679038323268));
#25514=CARTESIAN_POINT('Ctrl Pts',(-0.159019907330079,0.172243718567035,
8.01028364205933));
#25515=CARTESIAN_POINT('Ctrl Pts',(0.043798823814624,0.238882386272181,
8.00007230453372));
#25516=CARTESIAN_POINT('Ctrl Pts',(0.224452588327861,0.0927586493798742,
7.98895851547691));
#25517=CARTESIAN_POINT('Ctrl Pts',(0.199662353288342,-0.138268131282085,
7.9778447264201));
#25518=CARTESIAN_POINT('Ctrl Pts',(-0.00788109805936929,-0.242736523239671,
7.96673093736331));
#25519=CARTESIAN_POINT('Ctrl Pts',(-0.17763289672451,-0.142992642240008,
7.95731353790785));
#25520=CARTESIAN_POINT('Ctrl Pts',(-0.205074919755458,-0.0371300138498422,
7.95160073480467));
#25521=CARTESIAN_POINT('Ctrl Pts',(-0.205150812725382,4.6897404500125E-5,
7.94959252805377));
#25522=CARTESIAN_POINT('Ctrl Pts',(-0.205346535413967,0.000176006484619816,
8.02540747194623));
#25523=CARTESIAN_POINT('Ctrl Pts',(-0.205513566953093,0.0206418550558431,
8.02429930431288));
#25524=CARTESIAN_POINT('Ctrl Pts',(-0.193297509774496,0.109329974644086,
8.01948654032727));
#25525=CARTESIAN_POINT('Ctrl Pts',(-0.0659066106883685,0.233750816567481,
8.01096917998937));
#25526=CARTESIAN_POINT('Ctrl Pts',(0.160643147318701,0.182145284864098,
7.99985539093258));
#25527=CARTESIAN_POINT('Ctrl Pts',(0.240154410771491,-0.0361798917467206,
7.98874160187577));
#25528=CARTESIAN_POINT('Ctrl Pts',(0.0998496185014871,-0.221389203127338,
7.97762781281897));
#25529=CARTESIAN_POINT('Ctrl Pts',(-0.131798368373502,-0.203962249775518,
7.96651643617579));
#25530=CARTESIAN_POINT('Ctrl Pts',(-0.205810928136795,-0.067969576514468,
7.95910965588487));
#25531=CARTESIAN_POINT('Ctrl Pts',(-0.205814987838042,8.27714623007834E-7,
7.95540747194623));
#25532=CARTESIAN_POINT('Origin',(0.,0.,8.75459252805377));
#25533=CARTESIAN_POINT('',(-0.205193082001069,-0.000103910388300932,8.09540747194623));
#25534=CARTESIAN_POINT('',(-0.205787650466444,6.7877098390864E-5,8.08959252805377));
#25535=CARTESIAN_POINT('',(-0.205475,1.36055398187253E-14,8.75459252805377));
#25536=CARTESIAN_POINT('Ctrl Pts',(-0.205787650466444,6.7877098390855E-5,
8.08959252805377));
#25537=CARTESIAN_POINT('Ctrl Pts',(-0.205803722489804,0.00380176859574709,
8.08938922436523));
#25538=CARTESIAN_POINT('Ctrl Pts',(-0.204019440224857,0.0755588970087965,
8.08548132432442));
#25539=CARTESIAN_POINT('Ctrl Pts',(-0.120353900451207,0.210945656715802,
8.07786882793134));
#25540=CARTESIAN_POINT('Ctrl Pts',(0.111954069464546,0.215521269881544,
8.06675503887454));
#25541=CARTESIAN_POINT('Ctrl Pts',(0.241789209953822,0.0228278205475825,
8.05564124981773));
#25542=CARTESIAN_POINT('Ctrl Pts',(0.150311944496376,-0.190760191819292,
8.04452746076093));
#25543=CARTESIAN_POINT('Ctrl Pts',(-0.0787475484122947,-0.229743237245029,
8.03341367170412));
#25544=CARTESIAN_POINT('Ctrl Pts',(-0.196148549788041,-0.101630843190257,
8.0251020274684));
#25545=CARTESIAN_POINT('Ctrl Pts',(-0.205607377356971,-0.0168320149610218,
8.02049497958495));
#25546=CARTESIAN_POINT('Ctrl Pts',(-0.205455849451785,-0.000187890725276842,
8.01959252805376));
#25547=CARTESIAN_POINT('Ctrl Pts',(-0.205193082001069,-0.000103910388300946,
8.09540747194623));
#25548=CARTESIAN_POINT('Ctrl Pts',(-0.205005484772661,0.0408602139318314,
8.09319354909315));
#25549=CARTESIAN_POINT('Ctrl Pts',(-0.17326642156507,0.150638073432689,
8.08727502988781));
#25550=CARTESIAN_POINT('Ctrl Pts',(0.00557052926712743,0.242800524674804,
8.0776519143302));
#25551=CARTESIAN_POINT('Ctrl Pts',(0.207011538257192,0.127001372461354,
8.06653812527341));
#25552=CARTESIAN_POINT('Ctrl Pts',(0.218972538609993,-0.105043576259552,
8.05542433621658));
#25553=CARTESIAN_POINT('Ctrl Pts',(0.0305054910554562,-0.240940948354804,
8.0443105471598));
#25554=CARTESIAN_POINT('Ctrl Pts',(-0.164307195981861,-0.164741743111656,
8.03430492573633));
#25555=CARTESIAN_POINT('Ctrl Pts',(-0.204955181730555,-0.0477753281223429,
8.02800390066515));
#25556=CARTESIAN_POINT('Ctrl Pts',(-0.205346535413967,0.000176006484619816,
8.02540747194623));
#25557=CARTESIAN_POINT('Origin',(0.,0.,8.75459252805377));
#25558=CARTESIAN_POINT('',(-0.205725749329808,-0.000120218108977228,8.16540747194623));
#25559=CARTESIAN_POINT('',(-0.205255455161232,0.000145098000214199,8.15959252805377));
#25560=CARTESIAN_POINT('',(-0.205475,1.36055398187253E-14,8.75459252805377));
#25561=CARTESIAN_POINT('Ctrl Pts',(-0.205255455161232,0.000145098000214217,
8.15959252805377));
#25562=CARTESIAN_POINT('Ctrl Pts',(-0.205413266570088,0.024348109840268,
8.1582834691455));
#25563=CARTESIAN_POINT('Ctrl Pts',(-0.190262273248928,0.116853699781198,
8.15326981388497));
#25564=CARTESIAN_POINT('Ctrl Pts',(-0.0531714146829997,0.236972428990521,
8.14455156227216));
#25565=CARTESIAN_POINT('Ctrl Pts',(0.170256666670833,0.173192952787333,
8.13343777321537));
#25566=CARTESIAN_POINT('Ctrl Pts',(0.237846890178926,-0.0491119972437703,
8.12232398415856));
#25567=CARTESIAN_POINT('Ctrl Pts',(0.0877331577390571,-0.22646417922973,
8.11121019510175));
#25568=CARTESIAN_POINT('Ctrl Pts',(-0.138468730552596,-0.19707869266157,
8.10029970973349));
#25569=CARTESIAN_POINT('Ctrl Pts',(-0.205510858353677,-0.064237138716603,
8.0930938207175));
#25570=CARTESIAN_POINT('Ctrl Pts',(-0.205787650466444,6.7877098390855E-5,
8.08959252805377));
#25571=CARTESIAN_POINT('Ctrl Pts',(-0.205725749329808,-0.000120218108977229,
8.16540747194622));
#25572=CARTESIAN_POINT('Ctrl Pts',(-0.205301608939898,0.060897783274676,
8.16208779387343));
#25573=CARTESIAN_POINT('Ctrl Pts',(-0.144200557987511,0.190746562771969,
8.15506351944837));
#25574=CARTESIAN_POINT('Ctrl Pts',(0.0765574282985869,0.230482289451893,
8.14433464867103));
#25575=CARTESIAN_POINT('Ctrl Pts',(0.235161637351955,0.0606805561660993,
8.13322085961422));
#25576=CARTESIAN_POINT('Ctrl Pts',(0.178519732822726,-0.164662778342839,
8.12210707055743));
#25577=CARTESIAN_POINT('Ctrl Pts',(-0.0415233077106159,-0.239288404431658,
8.1109932815006));
#25578=CARTESIAN_POINT('Ctrl Pts',(-0.18729704716622,-0.123655403395563,
8.10209341529689));
#25579=CARTESIAN_POINT('Ctrl Pts',(-0.205319394540154,-0.0276857813902086,
8.09689814544542));
#25580=CARTESIAN_POINT('Ctrl Pts',(-0.205193082001069,-0.000103910388300946,
8.09540747194623));
#25581=CARTESIAN_POINT('Origin',(0.,0.,8.75459252805377));
#25582=CARTESIAN_POINT('',(-0.205557297878076,0.000179913196093145,8.23540747194623));
#25583=CARTESIAN_POINT('',(-0.205263287666448,-0.000148795917841437,8.22959252805377));
#25584=CARTESIAN_POINT('',(-0.205475,1.36055398187253E-14,8.75459252805377));
#25585=CARTESIAN_POINT('Ctrl Pts',(-0.205263287666448,-0.000148795917841445,
8.22959252805377));
#25586=CARTESIAN_POINT('Ctrl Pts',(-0.204964021088784,0.0444940904767351,
8.22717771392578));
#25587=CARTESIAN_POINT('Ctrl Pts',(-0.16869999758381,0.158066853952189,
8.22105830344552));
#25588=CARTESIAN_POINT('Ctrl Pts',(0.0186904834432735,0.242144166292971,
8.21123429661299));
#25589=CARTESIAN_POINT('Ctrl Pts',(0.213575627372185,0.115622587904077,
8.20012050755619));
#25590=CARTESIAN_POINT('Ctrl Pts',(0.212972577454982,-0.11672965644274,
8.18900671849938));
#25591=CARTESIAN_POINT('Ctrl Pts',(0.0174333121199337,-0.24223792244318,
8.17789292944259));
#25592=CARTESIAN_POINT('Ctrl Pts',(-0.169151380035818,-0.157355921249033,
8.16808819929403));
#25593=CARTESIAN_POINT('Ctrl Pts',(-0.204966665148331,-0.0441456674912357,
8.16198806549777));
#25594=CARTESIAN_POINT('Ctrl Pts',(-0.205255455161232,0.000145098000214217,
8.15959252805377));
#25595=CARTESIAN_POINT('Ctrl Pts',(-0.205557297878076,0.000179913196093175,
8.23540747194624));
#25596=CARTESIAN_POINT('Ctrl Pts',(-0.2056789846887,0.013457658201761,8.23468663500598));
#25597=CARTESIAN_POINT('Ctrl Pts',(-0.198456933057522,0.0948418873117451,
8.23026120171346));
#25598=CARTESIAN_POINT('Ctrl Pts',(-0.0898845214982184,0.22561892290705,
8.22213117206865));
#25599=CARTESIAN_POINT('Ctrl Pts',(0.14080680157081,0.197880191555585,8.21101738301186));
#25600=CARTESIAN_POINT('Ctrl Pts',(0.242616062304287,-0.0109805232406446,
8.19990359395504));
#25601=CARTESIAN_POINT('Ctrl Pts',(0.122356089757392,-0.209790640587143,
8.18878980489824));
#25602=CARTESIAN_POINT('Ctrl Pts',(-0.109897799356892,-0.21657700541653,
8.17767601584145));
#25603=CARTESIAN_POINT('Ctrl Pts',(-0.202233319405892,-0.0823136199806689,
8.16988190485743));
#25604=CARTESIAN_POINT('Ctrl Pts',(-0.205774928613328,-0.00719528490585479,
8.16579239022569));
#25605=CARTESIAN_POINT('Ctrl Pts',(-0.205725749329808,-0.000120218108977229,
8.16540747194622));
#25606=CARTESIAN_POINT('Origin',(0.,0.,8.75459252805377));
#25607=CARTESIAN_POINT('',(-0.205141210392772,7.81015472149649E-6,8.30540747194623));
#25608=CARTESIAN_POINT('',(-0.205792375932435,-6.17376947855616E-5,8.29959252805377));
#25609=CARTESIAN_POINT('',(-0.205475,1.36055398187253E-14,8.75459252805377));
#25610=CARTESIAN_POINT('Ctrl Pts',(-0.205792375932435,-6.17376947855664E-5,
8.29959252805376));
#25611=CARTESIAN_POINT('Ctrl Pts',(-0.205536440190278,0.0645933570331749,
8.29607195870605));
#25612=CARTESIAN_POINT('Ctrl Pts',(-0.137843789364693,0.197744956512954,
8.28884679300607));
#25613=CARTESIAN_POINT('Ctrl Pts',(0.088907503777123,0.226005723850825,
8.27791703095381));
#25614=CARTESIAN_POINT('Ctrl Pts',(0.238098615913173,0.0478767223322276,
8.26680324189701));
#25615=CARTESIAN_POINT('Ctrl Pts',(0.169355364681906,-0.174074386095383,
8.2556894528402));
#25616=CARTESIAN_POINT('Ctrl Pts',(-0.0544007724631579,-0.236693234792403,
8.24457566378341));
#25617=CARTESIAN_POINT('Ctrl Pts',(-0.190564537929879,-0.116131675020199,
8.23587668885459));
#25618=CARTESIAN_POINT('Ctrl Pts',(-0.205423129663277,-0.0239931161264832,
8.23088231027804));
#25619=CARTESIAN_POINT('Ctrl Pts',(-0.205263287666448,-0.000148795917841445,
8.22959252805377));
#25620=CARTESIAN_POINT('Ctrl Pts',(-0.205141210392772,7.81015472149649E-6,
8.30540747194623));
#25621=CARTESIAN_POINT('Ctrl Pts',(-0.2051526763295,0.0338265261367679,
8.30358087978625));
#25622=CARTESIAN_POINT('Ctrl Pts',(-0.181235068435874,0.136219282150282,
8.298049691274));
#25623=CARTESIAN_POINT('Ctrl Pts',(-0.0197379877628579,0.242061020031891,
8.28881390640948));
#25624=CARTESIAN_POINT('Ctrl Pts',(0.19266430806168,0.147863416631009,8.27770011735268));
#25625=CARTESIAN_POINT('Ctrl Pts',(0.22871877775246,-0.0816752488934883,
8.26658632829587));
#25626=CARTESIAN_POINT('Ctrl Pts',(0.0554243563205898,-0.236455632847443,
8.25547253923908));
#25627=CARTESIAN_POINT('Ctrl Pts',(-0.154070416783098,-0.178804103481232,
8.24507958712251));
#25628=CARTESIAN_POINT('Ctrl Pts',(-0.205053599820663,-0.0547806394870636,
8.23839123135824));
#25629=CARTESIAN_POINT('Ctrl Pts',(-0.205557297878076,0.000179913196093175,
8.23540747194624));
#25630=CARTESIAN_POINT('Origin',(0.,0.,8.75459252805377));
#25631=CARTESIAN_POINT('',(-0.205528628934285,-0.000183968246708688,8.37540747194623));
#25632=CARTESIAN_POINT('',(-0.205445190560286,0.000187702189675683,8.36959252805377));
#25633=CARTESIAN_POINT('',(-0.205475,1.36055398187253E-14,8.75459252805377));
#25634=CARTESIAN_POINT('Ctrl Pts',(-0.205445190560286,0.000187702189675667,
8.36959252805377));
#25635=CARTESIAN_POINT('Ctrl Pts',(-0.205599100693057,0.0171896010410893,
8.3686707998386));
#25636=CARTESIAN_POINT('Ctrl Pts',(-0.195892182403793,0.102351934160262,
8.36404447527116));
#25637=CARTESIAN_POINT('Ctrl Pts',(-0.0775539386019673,0.230148904034816,
8.35571355435145));
#25638=CARTESIAN_POINT('Ctrl Pts',(0.151300115555386,0.189977384132442,
8.34459976529464));
#25639=CARTESIAN_POINT('Ctrl Pts',(0.241667458088899,-0.0240825900331494,
8.33348597623784));
#25640=CARTESIAN_POINT('Ctrl Pts',(0.110833835536237,-0.216099496387572,
8.32237218718103));
#25641=CARTESIAN_POINT('Ctrl Pts',(-0.121447253622906,-0.210318082982978,
8.31125839812424));
#25642=CARTESIAN_POINT('Ctrl Pts',(-0.204198823013731,-0.0748427841522689,
8.30366517841514));
#25643=CARTESIAN_POINT('Ctrl Pts',(-0.205805754191272,-0.00344138519968516,
8.29977655505832));
#25644=CARTESIAN_POINT('Ctrl Pts',(-0.205792375932435,-6.17376947855664E-5,
8.29959252805376));
#25645=CARTESIAN_POINT('Ctrl Pts',(-0.205528628934285,-0.000183968246708686,
8.37540747194623));
#25646=CARTESIAN_POINT('Ctrl Pts',(-0.205029971468385,0.0538489651766571,
8.37247512456652));
#25647=CARTESIAN_POINT('Ctrl Pts',(-0.155498687892329,0.176953566042901,
8.36583818083455));
#25648=CARTESIAN_POINT('Ctrl Pts',(0.05214561050461,0.237200254924533,8.35549664075031));
#25649=CARTESIAN_POINT('Ctrl Pts',(0.22756616748523,0.0848337492213278,
8.3443828516935));
#25650=CARTESIAN_POINT('Ctrl Pts',(0.19469283040568,-0.145182048984365,
8.3332690626367));
#25651=CARTESIAN_POINT('Ctrl Pts',(-0.016385062217743,-0.242311071399234,
8.3221552735799));
#25652=CARTESIAN_POINT('Ctrl Pts',(-0.180238976017125,-0.138138524644507,
8.31286807668307));
#25653=CARTESIAN_POINT('Ctrl Pts',(-0.205129421730959,-0.0347627816519641,
8.30728547613852));
#25654=CARTESIAN_POINT('Ctrl Pts',(-0.205141210392772,7.81015472149649E-6,
8.30540747194623));
#25655=CARTESIAN_POINT('Origin',(0.,0.,8.75459252805377));
#25656=CARTESIAN_POINT('',(-0.205746142027763,0.000106562949819478,8.44540747194623));
#25657=CARTESIAN_POINT('',(-0.205153388991823,-5.25555079458241E-5,8.43959252805377));
#25658=CARTESIAN_POINT('',(-0.205475,1.36055398187253E-14,8.75459252805377));
#25659=CARTESIAN_POINT('Ctrl Pts',(-0.205153388991823,-5.25555079458132E-5,
8.43959252805377));
#25660=CARTESIAN_POINT('Ctrl Pts',(-0.205067466342422,0.0374800397938141,
8.43756504461887));
#25661=CARTESIAN_POINT('Ctrl Pts',(-0.177236782892462,0.143710413212875,
8.43183296483171));
#25662=CARTESIAN_POINT('Ctrl Pts',(-0.00662099741593451,0.242774159607174,
8.42239628869227));
#25663=CARTESIAN_POINT('Ctrl Pts',(0.200377384150519,0.13722986443753,8.41128249963547));
#25664=CARTESIAN_POINT('Ctrl Pts',(0.223968073814581,-0.0939224866161797,
8.40016871057866));
#25665=CARTESIAN_POINT('Ctrl Pts',(0.0425582454220915,-0.239106518161268,
8.38905492152186));
#25666=CARTESIAN_POINT('Ctrl Pts',(-0.15952962843628,-0.171543743623583,
8.37886286068023));
#25667=CARTESIAN_POINT('Ctrl Pts',(-0.204980507373406,-0.0511441782984296,
8.37237539619086));
#25668=CARTESIAN_POINT('Ctrl Pts',(-0.205445190560286,0.000187702189675667,
8.36959252805377));
#25669=CARTESIAN_POINT('Ctrl Pts',(-0.205746142027763,0.000106562949819445,
8.44540747194623));
#25670=CARTESIAN_POINT('Ctrl Pts',(-0.205784824946164,0.00623504139834656,
8.44507396569907));
#25671=CARTESIAN_POINT('Ctrl Pts',(-0.202756731895245,0.0804000642300188,
8.44103586309964));
#25672=CARTESIAN_POINT('Ctrl Pts',(-0.112885495048793,0.215034836414334,
8.43329316414793));
#25673=CARTESIAN_POINT('Ctrl Pts',(0.119440067448933,0.211464412612195,
8.42217937509113));
#25674=CARTESIAN_POINT('Ctrl Pts',(0.242440804004482,0.0143381848173731,
8.41106558603433));
#25675=CARTESIAN_POINT('Ctrl Pts',(0.143532711926644,-0.195911931545135,
8.39995179697752));
#25676=CARTESIAN_POINT('Ctrl Pts',(-0.0867524934706339,-0.226841642534413,
8.38883800792072));
#25677=CARTESIAN_POINT('Ctrl Pts',(-0.197822911553203,-0.0967627749490978,
8.38065656624362));
#25678=CARTESIAN_POINT('Ctrl Pts',(-0.205659952978076,-0.0144138230072569,
8.37617972091879));
#25679=CARTESIAN_POINT('Ctrl Pts',(-0.205528628934285,-0.000183968246708686,
8.37540747194623));
#25680=CARTESIAN_POINT('Origin',(0.,0.,8.75459252805377));
#25681=CARTESIAN_POINT('',(-0.205208153945529,0.000116160874735274,8.51540747194623));
#25682=CARTESIAN_POINT('',(-0.205637856381221,-0.00016039379494083,8.50959252805377));
#25683=CARTESIAN_POINT('',(-0.205475,1.36055398187253E-14,8.75459252805377));
#25684=CARTESIAN_POINT('Ctrl Pts',(-0.205637856381221,-0.000160393794940828,
8.50959252805377));
#25685=CARTESIAN_POINT('Ctrl Pts',(-0.205143095125645,0.0574950566938362,
8.50645928939915));
#25686=CARTESIAN_POINT('Ctrl Pts',(-0.14979446013605,0.184152224411407,
8.49962145439225));
#25687=CARTESIAN_POINT('Ctrl Pts',(0.0648946403841687,0.234033639096515,
8.48907902303309));
#25688=CARTESIAN_POINT('Ctrl Pts',(0.231820203331014,0.0724053476422597,
8.4779652339763));
#25689=CARTESIAN_POINT('Ctrl Pts',(0.18655812004824,-0.155496664131617,
8.46685144491948));
#25690=CARTESIAN_POINT('Ctrl Pts',(-0.0294627337392764,-0.241070672344369,
8.45573765586269));
#25691=CARTESIAN_POINT('Ctrl Pts',(-0.184027107137038,-0.130632731643015,
8.44665135024078));
#25692=CARTESIAN_POINT('Ctrl Pts',(-0.205224463301346,-0.031099122557323,
8.44126964097114));
#25693=CARTESIAN_POINT('Ctrl Pts',(-0.205153388991823,-5.25555079458132E-5,
8.43959252805377));
#25694=CARTESIAN_POINT('Ctrl Pts',(-0.205208153945529,0.00011616087473525,
8.51540747194623));
#25695=CARTESIAN_POINT('Ctrl Pts',(-0.205345942894438,0.0267421115464025,
8.51396821047934));
#25696=CARTESIAN_POINT('Ctrl Pts',(-0.188159225831614,0.121731577366826,
8.50882435266019));
#25697=CARTESIAN_POINT('Ctrl Pts',(-0.0448312245259985,0.238689656539759,
8.49997589848875));
#25698=CARTESIAN_POINT('Ctrl Pts',(0.176222693303572,0.167118876029215,
8.48886210943197));
#25699=CARTESIAN_POINT('Ctrl Pts',(0.235979340716847,-0.0574194692648986,
8.47774832037514));
#25700=CARTESIAN_POINT('Ctrl Pts',(0.0797407360187229,-0.229400234578822,
8.46663453131836));
#25701=CARTESIAN_POINT('Ctrl Pts',(-0.14260643792996,-0.192548870793535,
8.4558542485087));
#25702=CARTESIAN_POINT('Ctrl Pts',(-0.205355134049455,-0.0618402618335321,
8.44877856205133));
#25703=CARTESIAN_POINT('Ctrl Pts',(-0.205746142027763,0.000106562949819445,
8.44540747194623));
#25704=CARTESIAN_POINT('Origin',(0.,0.,8.75459252805377));
#25705=CARTESIAN_POINT('',(-0.205267617401664,-0.000235214789251412,8.58540747194623));
#25706=CARTESIAN_POINT('',(-0.205656479110814,0.00014959981056081,8.57959252805377));
#25707=CARTESIAN_POINT('',(-0.205475,1.36055398187253E-14,8.75459252805377));
#25708=CARTESIAN_POINT('',(-0.0530170217188482,-0.198517432567176,8.6));
#25709=CARTESIAN_POINT('Ctrl Pts',(-0.0530170217188485,-0.198517432567176,
8.6));
#25710=CARTESIAN_POINT('Ctrl Pts',(-0.119028790974543,-0.180888011517996,
8.59629540364773));
#25711=CARTESIAN_POINT('Ctrl Pts',(-0.192495809737496,-0.111280924019936,
8.59143122762981));
#25712=CARTESIAN_POINT('Ctrl Pts',(-0.205429477035024,-0.0216596338882675,
8.58656705161189));
#25713=CARTESIAN_POINT('Ctrl Pts',(-0.205267617401664,-0.000235214789251429,
8.58540747194623));
#25714=CARTESIAN_POINT('',(0.0531303528054007,-0.198873455395433,8.6));
#25715=CARTESIAN_POINT('Origin',(0.,0.,8.6));
#25716=CARTESIAN_POINT('Ctrl Pts',(0.0531304158591932,-0.198873653475093,
8.6));
#25717=CARTESIAN_POINT('Ctrl Pts',(-0.0113304135988541,-0.216006401657972,
8.59636770818144));
#25718=CARTESIAN_POINT('Ctrl Pts',(-0.149305780278568,-0.184063659998061,
8.58956521753269));
#25719=CARTESIAN_POINT('Ctrl Pts',(-0.205170728792184,-0.0581586047744906,
8.58276272688396));
#25720=CARTESIAN_POINT('Ctrl Pts',(-0.205656479110814,0.000149599810560773,
8.57959252805377));
#25721=CARTESIAN_POINT('Origin',(0.6,1.,2.15));
#25722=CARTESIAN_POINT('',(0.473748222256554,0.999995809921948,2.01934196736194));
#25723=CARTESIAN_POINT('',(0.473622351265484,0.999839631194249,2.00565803263806));
#25724=CARTESIAN_POINT('',(0.47355,1.,2.15));
#25725=CARTESIAN_POINT('',(0.504188384727762,1.08252112989365,2.));
#25726=CARTESIAN_POINT('Ctrl Pts',(0.473622351265484,0.999839631194249,
2.00565803263806));
#25727=CARTESIAN_POINT('Ctrl Pts',(0.473885391482026,1.02975027328269,2.00377202175871));
#25728=CARTESIAN_POINT('Ctrl Pts',(0.484630619730662,1.05981347843636,2.00188601087935));
#25729=CARTESIAN_POINT('Ctrl Pts',(0.504188384727762,1.08252112989365,2.));
#25730=CARTESIAN_POINT('',(0.695988975197609,1.08263517233072,2.));
#25731=CARTESIAN_POINT('Origin',(0.6,1.,2.));
#25732=CARTESIAN_POINT('Ctrl Pts',(0.69598984030289,1.08263572859344,2.));
#25733=CARTESIAN_POINT('Ctrl Pts',(0.670163701400848,1.11242100165145,2.0024908160387));
#25734=CARTESIAN_POINT('Ctrl Pts',(0.629259702670384,1.12936970915052,2.0049816320774));
#25735=CARTESIAN_POINT('Ctrl Pts',(0.589969605604523,1.12624206673302,2.0074724481161));
#25736=CARTESIAN_POINT('Ctrl Pts',(0.548691445154515,1.12295616684523,2.01008929846199));
#25737=CARTESIAN_POINT('Ctrl Pts',(0.509194644046665,1.09751080441727,2.01270614880789));
#25738=CARTESIAN_POINT('Ctrl Pts',(0.489166147389288,1.06128256435802,2.01532299915378));
#25739=CARTESIAN_POINT('Ctrl Pts',(0.478912868232585,1.04273607706854,2.01666265522317));
#25740=CARTESIAN_POINT('Ctrl Pts',(0.473761783314308,1.02136364588323,2.01800231129256));
#25741=CARTESIAN_POINT('Ctrl Pts',(0.473748222256554,0.999995809921948,
2.01934196736194));
#25742=CARTESIAN_POINT('Origin',(0.6,1.,2.15));
#25743=CARTESIAN_POINT('',(0.473418004372097,0.999922226677399,2.06934196736194));
#25744=CARTESIAN_POINT('',(0.473391518308752,1.00006258785156,2.05565803263806));
#25745=CARTESIAN_POINT('',(0.47355,1.,2.15));
#25746=CARTESIAN_POINT('Ctrl Pts',(0.473391518308752,1.00006258785156,2.05565803263806));
#25747=CARTESIAN_POINT('Ctrl Pts',(0.473368951434719,1.00377931266751,2.05542330751329));
#25748=CARTESIAN_POINT('Ctrl Pts',(0.473518765465857,1.00749417831325,2.05518858238852));
#25749=CARTESIAN_POINT('Ctrl Pts',(0.473846950690071,1.01119320034366,2.05495385726375));
#25750=CARTESIAN_POINT('Ctrl Pts',(0.477505747839885,1.05243201995956,2.05233700691785));
#25751=CARTESIAN_POINT('Ctrl Pts',(0.503334424526069,1.09170162561774,2.04972015657196));
#25752=CARTESIAN_POINT('Ctrl Pts',(0.539751219345993,1.1113984538297,2.04710330622607));
#25753=CARTESIAN_POINT('Ctrl Pts',(0.576168014165918,1.13109528204167,2.04448645588018));
#25754=CARTESIAN_POINT('Ctrl Pts',(0.623172927119585,1.13121933280741,2.04186960553428));
#25755=CARTESIAN_POINT('Ctrl Pts',(0.659688152943108,1.11170438100077,2.03925275518839));
#25756=CARTESIAN_POINT('Ctrl Pts',(0.69620337876663,1.09218942919414,2.0366359048425));
#25757=CARTESIAN_POINT('Ctrl Pts',(0.722228917460009,1.05303547481514,2.0340190544966));
#25758=CARTESIAN_POINT('Ctrl Pts',(0.726095080681017,1.01182045619333,2.03140220415071));
#25759=CARTESIAN_POINT('Ctrl Pts',(0.729961243902025,0.970605437571516,
2.02878535380482));
#25760=CARTESIAN_POINT('Ctrl Pts',(0.711668031650661,0.927329354706896,
2.02616850345893));
#25761=CARTESIAN_POINT('Ctrl Pts',(0.679417475504429,0.901356588462624,
2.02355165311304));
#25762=CARTESIAN_POINT('Ctrl Pts',(0.647166919358198,0.875383822218351,
2.02093480276714));
#25763=CARTESIAN_POINT('Ctrl Pts',(0.600959019317099,0.866714372594425,
2.01831795242125));
#25764=CARTESIAN_POINT('Ctrl Pts',(0.561514908627169,0.879318620323889,
2.01570110207536));
#25765=CARTESIAN_POINT('Ctrl Pts',(0.522070797937238,0.891922868053354,
2.01308425172946));
#25766=CARTESIAN_POINT('Ctrl Pts',(0.489390476598475,0.925800813136209,
2.01046740138357));
#25767=CARTESIAN_POINT('Ctrl Pts',(0.47813574698779,0.965573631142046,2.00785055103768));
#25768=CARTESIAN_POINT('Ctrl Pts',(0.474992502439002,0.976681467377235,
2.00711971157114));
#25769=CARTESIAN_POINT('Ctrl Pts',(0.473520421751905,0.988249094815541,
2.0063888721046));
#25770=CARTESIAN_POINT('Ctrl Pts',(0.473622351265484,0.999839631194249,
2.00565803263806));
#25771=CARTESIAN_POINT('Ctrl Pts',(0.473748222256554,0.999995809921948,
2.01934196736194));
#25772=CARTESIAN_POINT('Ctrl Pts',(0.473735293486444,0.979624254554346,
2.02061916163845));
#25773=CARTESIAN_POINT('Ctrl Pts',(0.478391980488661,0.959256875893503,
2.02189635591496));
#25774=CARTESIAN_POINT('Ctrl Pts',(0.487748897958052,0.941346462457022,
2.02317355019146));
#25775=CARTESIAN_POINT('Ctrl Pts',(0.5069203373911,0.904649718305799,2.02579040053735));
#25776=CARTESIAN_POINT('Ctrl Pts',(0.545823408464101,0.878267347693885,
2.02840725088324));
#25777=CARTESIAN_POINT('Ctrl Pts',(0.587007341569528,0.874020924816605,
2.03102410122914));
#25778=CARTESIAN_POINT('Ctrl Pts',(0.628191274674955,0.869774501939324,
2.03364095157503));
#25779=CARTESIAN_POINT('Ctrl Pts',(0.671656069812808,0.887664026796678,
2.03625780192092));
#25780=CARTESIAN_POINT('Ctrl Pts',(0.697914735578316,0.919671996193035,
2.03887465226682));
#25781=CARTESIAN_POINT('Ctrl Pts',(0.724173401343824,0.951679965589392,
2.04149150261271));
#25782=CARTESIAN_POINT('Ctrl Pts',(0.733225937736988,0.997806379524751,
2.0441083529586));
#25783=CARTESIAN_POINT('Ctrl Pts',(0.72101148240133,1.03736538090912,2.04672520330449));
#25784=CARTESIAN_POINT('Ctrl Pts',(0.708797027065672,1.07692438229349,2.04934205365039));
#25785=CARTESIAN_POINT('Ctrl Pts',(0.675315580001192,1.10991597112687,2.05195890399628));
#25786=CARTESIAN_POINT('Ctrl Pts',(0.635581432895856,1.12154745886576,2.05457575434217));
#25787=CARTESIAN_POINT('Ctrl Pts',(0.59584728579052,1.13317894660465,2.05719260468807));
#25788=CARTESIAN_POINT('Ctrl Pts',(0.549860438644329,1.12345033324905,2.05980945503396));
#25789=CARTESIAN_POINT('Ctrl Pts',(0.518241526751132,1.09672346863534,2.06242630537985));
#25790=CARTESIAN_POINT('Ctrl Pts',(0.490387977892526,1.07317939375162,2.06473152604054));
#25791=CARTESIAN_POINT('Ctrl Pts',(0.473684088301786,1.03644450847376,2.06703674670124));
#25792=CARTESIAN_POINT('Ctrl Pts',(0.473418004372097,0.999922226677399,
2.06934196736194));
#25793=CARTESIAN_POINT('Origin',(0.6,1.,2.15));
#25794=CARTESIAN_POINT('',(0.473569322058917,1.00010891293128,2.11934196736194));
#25795=CARTESIAN_POINT('',(0.473740555540666,1.00002674768131,2.10565803263806));
#25796=CARTESIAN_POINT('',(0.47355,1.,2.15));
#25797=CARTESIAN_POINT('Ctrl Pts',(0.473740555540666,1.00002674768131,2.10565803263806));
#25798=CARTESIAN_POINT('Ctrl Pts',(0.473703568953707,1.01916777914625,2.10445774292198));
#25799=CARTESIAN_POINT('Ctrl Pts',(0.477794964495735,1.03829380542625,2.10325745320589));
#25800=CARTESIAN_POINT('Ctrl Pts',(0.486097635636878,1.0553725521712,2.10205716348981));
#25801=CARTESIAN_POINT('Ctrl Pts',(0.504198971969625,1.09260733284801,2.09944031314392));
#25802=CARTESIAN_POINT('Ctrl Pts',(0.542317321105284,1.12011099531618,2.09682346279803));
#25803=CARTESIAN_POINT('Ctrl Pts',(0.583359964347627,1.12555066422426,2.09420661245214));
#25804=CARTESIAN_POINT('Ctrl Pts',(0.62440260758997,1.13099033313234,2.09158976210624));
#25805=CARTESIAN_POINT('Ctrl Pts',(0.668369544938998,1.11436600848032,2.08897291176035));
#25806=CARTESIAN_POINT('Ctrl Pts',(0.695545474812698,1.08313205071709,2.08635606141446));
#25807=CARTESIAN_POINT('Ctrl Pts',(0.722721404686398,1.05189809295385,2.08373921106856));
#25808=CARTESIAN_POINT('Ctrl Pts',(0.733106327084771,1.00605450207939,2.08112236072267));
#25809=CARTESIAN_POINT('Ctrl Pts',(0.722043527705466,0.966158451314527,
2.07850551037678));
#25810=CARTESIAN_POINT('Ctrl Pts',(0.71098072832616,0.926262400549665,2.07588866003089));
#25811=CARTESIAN_POINT('Ctrl Pts',(0.678470207169174,0.892313889894401,
2.073271809685));
#25812=CARTESIAN_POINT('Ctrl Pts',(0.639090051974211,0.87953512362367,2.0706549593391));
#25813=CARTESIAN_POINT('Ctrl Pts',(0.599709896779248,0.86675635735294,2.06803810899321));
#25814=CARTESIAN_POINT('Ctrl Pts',(0.553460107546307,0.875147335466744,
2.06542125864732));
#25815=CARTESIAN_POINT('Ctrl Pts',(0.52107967173656,0.900946841310449,2.06280440830142));
#25816=CARTESIAN_POINT('Ctrl Pts',(0.491603682429651,0.924432194096951,
2.0604222830803));
#25817=CARTESIAN_POINT('Ctrl Pts',(0.473620539892396,0.962343132242784,
2.05804015785918));
#25818=CARTESIAN_POINT('Ctrl Pts',(0.473391518308752,1.00006258785156,2.05565803263806));
#25819=CARTESIAN_POINT('Ctrl Pts',(0.473418004372097,0.999922226677399,
2.06934196736194));
#25820=CARTESIAN_POINT('Ctrl Pts',(0.473382033997262,0.994984986883897,
2.06965359704714));
#25821=CARTESIAN_POINT('Ctrl Pts',(0.473646461235087,0.990051632376521,
2.06996522673233));
#25822=CARTESIAN_POINT('Ctrl Pts',(0.474224350273596,0.985155275839,2.07027685641753));
#25823=CARTESIAN_POINT('Ctrl Pts',(0.47907706232946,0.944039063528183,2.07289370676342));
#25824=CARTESIAN_POINT('Ctrl Pts',(0.50603346308139,0.905531754778367,2.07551055710931));
#25825=CARTESIAN_POINT('Ctrl Pts',(0.543005874916624,0.886900335416373,
2.0781274074552));
#25826=CARTESIAN_POINT('Ctrl Pts',(0.579978286751859,0.868268916054378,
2.0807442578011));
#25827=CARTESIAN_POINT('Ctrl Pts',(0.626966709670398,0.869513386080205,
2.08336110814699));
#25828=CARTESIAN_POINT('Ctrl Pts',(0.662901030784248,0.890075786233013,
2.08597795849288));
#25829=CARTESIAN_POINT('Ctrl Pts',(0.698835351898097,0.910638186385821,
2.08859480883878));
#25830=CARTESIAN_POINT('Ctrl Pts',(0.723715571207256,0.95051851666561,2.09121165918467));
#25831=CARTESIAN_POINT('Ctrl Pts',(0.726385074899299,0.991833924307951,
2.09382850953056));
#25832=CARTESIAN_POINT('Ctrl Pts',(0.729054578591342,1.03314933195029,2.09644535987645));
#25833=CARTESIAN_POINT('Ctrl Pts',(0.709513366666269,1.07589981695519,2.09906221022235));
#25834=CARTESIAN_POINT('Ctrl Pts',(0.676523964943026,1.10091557332887,2.10167906056824));
#25835=CARTESIAN_POINT('Ctrl Pts',(0.643534563219784,1.12593132970255,2.10429591091413));
#25836=CARTESIAN_POINT('Ctrl Pts',(0.597096971698373,1.13321235744502,2.10691276126002));
#25837=CARTESIAN_POINT('Ctrl Pts',(0.558034351233094,1.1194937471697,2.10952961160592));
#25838=CARTESIAN_POINT('Ctrl Pts',(0.518971730767816,1.10577513689439,2.11214646195181));
#25839=CARTESIAN_POINT('Ctrl Pts',(0.48728408135867,1.0710568886013,2.1147633122977));
#25840=CARTESIAN_POINT('Ctrl Pts',(0.477180525319141,1.0309070826023,2.11738016264359));
#25841=CARTESIAN_POINT('Ctrl Pts',(0.474655708422174,1.02087389149615,2.11803409754971));
#25842=CARTESIAN_POINT('Ctrl Pts',(0.473478752433508,1.01050151615012,2.11868803245583));
#25843=CARTESIAN_POINT('Ctrl Pts',(0.473569322058917,1.00010891293128,2.11934196736194));
#25844=CARTESIAN_POINT('Origin',(0.6,1.,2.15));
#25845=CARTESIAN_POINT('',(0.473701319324768,0.999928563934628,2.16934196736194));
#25846=CARTESIAN_POINT('',(0.473475969746711,0.999901036847401,2.15565803263806));
#25847=CARTESIAN_POINT('',(0.47355,1.,2.15));
#25848=CARTESIAN_POINT('Ctrl Pts',(0.473475969746711,0.999901036847401,
2.15565803263806));
#25849=CARTESIAN_POINT('Ctrl Pts',(0.473771376261924,1.03425627771038,2.15349217833067));
#25850=CARTESIAN_POINT('Ctrl Pts',(0.488302943448428,1.0688317671636,2.15132632402327));
#25851=CARTESIAN_POINT('Ctrl Pts',(0.513274800541643,1.09229629753053,2.14916046971588));
#25852=CARTESIAN_POINT('Ctrl Pts',(0.543446549698046,1.12064684917997,2.14654361936999));
#25853=CARTESIAN_POINT('Ctrl Pts',(0.588859242361366,1.13277740107318,2.1439267690241));
#25854=CARTESIAN_POINT('Ctrl Pts',(0.629149287366476,1.12324847117969,2.1413099186782));
#25855=CARTESIAN_POINT('Ctrl Pts',(0.669439332371586,1.11371954128621,2.13869306833231));
#25856=CARTESIAN_POINT('Ctrl Pts',(0.704606729718486,1.08253112960603,2.13607621798642));
#25857=CARTESIAN_POINT('Ctrl Pts',(0.718882000334445,1.04366848746118,2.13345936764053));
#25858=CARTESIAN_POINT('Ctrl Pts',(0.733157270950405,1.00480584531632,2.13084251729463));
#25859=CARTESIAN_POINT('Ctrl Pts',(0.726540414835423,0.958268972706794,
2.12822566694874));
#25860=CARTESIAN_POINT('Ctrl Pts',(0.701998509069979,0.924925562785253,
2.12560881660285));
#25861=CARTESIAN_POINT('Ctrl Pts',(0.677456603304535,0.891582152863712,
2.12299196625696));
#25862=CARTESIAN_POINT('Ctrl Pts',(0.634989647888627,0.871432205630162,
2.12037511591106));
#25863=CARTESIAN_POINT('Ctrl Pts',(0.59364033014263,0.873511184567866,2.11775826556517));
#25864=CARTESIAN_POINT('Ctrl Pts',(0.552291012396633,0.87559016350557,2.11514141521928));
#25865=CARTESIAN_POINT('Ctrl Pts',(0.512059332320547,0.899898068614528,
2.11252456487339));
#25866=CARTESIAN_POINT('Ctrl Pts',(0.490985654047422,0.935534970611733,
2.10990771452749));
#25867=CARTESIAN_POINT('Ctrl Pts',(0.479577992537903,0.954826036459998,
2.10849115389768));
#25868=CARTESIAN_POINT('Ctrl Pts',(0.473784206454455,0.977436841907783,
2.10707459326787));
#25869=CARTESIAN_POINT('Ctrl Pts',(0.473740555540666,1.00002674768131,2.10565803263806));
#25870=CARTESIAN_POINT('Ctrl Pts',(0.473569322058917,1.00010891293128,2.11934196736194));
#25871=CARTESIAN_POINT('Ctrl Pts',(0.473841184769449,0.968913451231703,
2.12130488280172));
#25872=CARTESIAN_POINT('Ctrl Pts',(0.485533699168036,0.937535732473691,
2.1232677982415));
#25873=CARTESIAN_POINT('Ctrl Pts',(0.506474126044697,0.914602214201428,
2.12523071368127));
#25874=CARTESIAN_POINT('Ctrl Pts',(0.534390745479694,0.884028515504489,
2.12784756402717));
#25875=CARTESIAN_POINT('Ctrl Pts',(0.578743447019601,0.868462481815532,
2.13046441437306));
#25876=CARTESIAN_POINT('Ctrl Pts',(0.619643953027205,0.874884108988649,
2.13308126471895));
#25877=CARTESIAN_POINT('Ctrl Pts',(0.660544459034809,0.881305736161766,
2.13569811506484));
#25878=CARTESIAN_POINT('Ctrl Pts',(0.697992769510109,0.909715024196956,
2.13831496541074));
#25879=CARTESIAN_POINT('Ctrl Pts',(0.715196616413391,0.947372909972802,
2.14093181575663));
#25880=CARTESIAN_POINT('Ctrl Pts',(0.732400463316672,0.985030795748647,
2.14354866610252));
#25881=CARTESIAN_POINT('Ctrl Pts',(0.729359846647935,1.03193727926515,2.14616551644841));
#25882=CARTESIAN_POINT('Ctrl Pts',(0.707438215309595,1.0670589360858,2.14878236679431));
#25883=CARTESIAN_POINT('Ctrl Pts',(0.685516583971256,1.10218059290645,2.1513992171402));
#25884=CARTESIAN_POINT('Ctrl Pts',(0.644713937963314,1.12551742303125,2.15401606748609));
#25885=CARTESIAN_POINT('Ctrl Pts',(0.603326668644815,1.12660491425775,2.15663291783199));
#25886=CARTESIAN_POINT('Ctrl Pts',(0.561939399326316,1.12769240548424,2.15924976817788));
#25887=CARTESIAN_POINT('Ctrl Pts',(0.51996750669726,1.10653055781244,2.16186661852377));
#25888=CARTESIAN_POINT('Ctrl Pts',(0.496231686388225,1.07260859537424,2.16448346886966));
#25889=CARTESIAN_POINT('Ctrl Pts',(0.481542214702607,1.05161518961582,2.16610296836709));
#25890=CARTESIAN_POINT('Ctrl Pts',(0.473837240540682,1.02573460264732,2.16772246786452));
#25891=CARTESIAN_POINT('Ctrl Pts',(0.473701319324768,0.999928563934628,
2.16934196736194));
#25892=CARTESIAN_POINT('Origin',(0.6,1.,2.15));
#25893=CARTESIAN_POINT('',(0.473352235667534,0.999991049382066,2.21934196736194));
#25894=CARTESIAN_POINT('',(0.473504867419963,1.00010483506638,2.20565803263806));
#25895=CARTESIAN_POINT('',(0.47355,1.,2.15));
#25896=CARTESIAN_POINT('Ctrl Pts',(0.473504867419963,1.00010483506638,2.20565803263806));
#25897=CARTESIAN_POINT('Ctrl Pts',(0.473432601452696,1.00827186028206,2.20514346408525));
#25898=CARTESIAN_POINT('Ctrl Pts',(0.474157534286366,1.01642611923938,2.20462889553244));
#25899=CARTESIAN_POINT('Ctrl Pts',(0.475726914006531,1.02441447959464,2.20411432697963));
#25900=CARTESIAN_POINT('Ctrl Pts',(0.48370803108242,1.0650394720171,2.20149747663373));
#25901=CARTESIAN_POINT('Ctrl Pts',(0.513528695332623,1.10137390406913,2.19888062628784));
#25902=CARTESIAN_POINT('Ctrl Pts',(0.551816966436341,1.11712498450026,2.19626377594195));
#25903=CARTESIAN_POINT('Ctrl Pts',(0.59010523754006,1.1328760649314,2.19364692559606));
#25904=CARTESIAN_POINT('Ctrl Pts',(0.636861115497294,1.12804379374164,2.19103007525016));
#25905=CARTESIAN_POINT('Ctrl Pts',(0.671118708852879,1.10479501880275,2.18841322490427));
#25906=CARTESIAN_POINT('Ctrl Pts',(0.705376302208464,1.08154624386386,2.18579637455838));
#25907=CARTESIAN_POINT('Ctrl Pts',(0.7271356109624,1.03988096517584,2.18317952421248));
#25908=CARTESIAN_POINT('Ctrl Pts',(0.726639502419725,0.998482388913484,
2.18056267386659));
#25909=CARTESIAN_POINT('Ctrl Pts',(0.726143393877049,0.95708381265113,2.1779458235207));
#25910=CARTESIAN_POINT('Ctrl Pts',(0.703391868037763,0.915951938814441,
2.17532897317481));
#25911=CARTESIAN_POINT('Ctrl Pts',(0.668586979533722,0.893530788668923,
2.17271212282892));
#25912=CARTESIAN_POINT('Ctrl Pts',(0.63378209102968,0.871109638523405,2.17009527248302));
#25913=CARTESIAN_POINT('Ctrl Pts',(0.586923839860883,0.867399212069058,
2.16747842213713));
#25914=CARTESIAN_POINT('Ctrl Pts',(0.549024022842182,0.88406330841772,2.16486157179124));
#25915=CARTESIAN_POINT('Ctrl Pts',(0.511124205823482,0.900727404766382,
2.16224472144534));
#25916=CARTESIAN_POINT('Ctrl Pts',(0.482182822954877,0.937766023918054,
2.15962787109945));
#25917=CARTESIAN_POINT('Ctrl Pts',(0.475177534345317,0.978570609196729,
2.15701102075356));
#25918=CARTESIAN_POINT('Ctrl Pts',(0.473970221356853,0.985602996945691,
2.15656002471506));
#25919=CARTESIAN_POINT('Ctrl Pts',(0.473414457221305,0.992747241932372,
2.15610902867656));
#25920=CARTESIAN_POINT('Ctrl Pts',(0.473475969746711,0.999901036847401,
2.15565803263806));
#25921=CARTESIAN_POINT('Ctrl Pts',(0.473701319324768,0.999928563934628,
2.16934196736194));
#25922=CARTESIAN_POINT('Ctrl Pts',(0.473617613747686,0.984036200493609,
2.17033931821041));
#25923=CARTESIAN_POINT('Ctrl Pts',(0.476404528994482,0.968172110044866,
2.17133666905888));
#25924=CARTESIAN_POINT('Ctrl Pts',(0.482198594761734,0.953495162034513,
2.17233401990734));
#25925=CARTESIAN_POINT('Ctrl Pts',(0.497401071433289,0.914985768337587,
2.17495087025323));
#25926=CARTESIAN_POINT('Ctrl Pts',(0.533305772765409,0.884649058148337,
2.17756772059913));
#25927=CARTESIAN_POINT('Ctrl Pts',(0.573812603904437,0.876088372947374,
2.18018457094502));
#25928=CARTESIAN_POINT('Ctrl Pts',(0.614319435043466,0.86752768774641,2.18280142129091));
#25929=CARTESIAN_POINT('Ctrl Pts',(0.659428395989404,0.880743027533735,
2.1854182716368));
#25930=CARTESIAN_POINT('Ctrl Pts',(0.688912092443748,0.909808476845009,
2.1880351219827));
#25931=CARTESIAN_POINT('Ctrl Pts',(0.718395788898092,0.938873926156282,
2.19065197232859));
#25932=CARTESIAN_POINT('Ctrl Pts',(0.732254220860843,0.983789484991505,
2.19326882267448));
#25933=CARTESIAN_POINT('Ctrl Pts',(0.724273102711297,1.02441448287903,2.19588567302037));
#25934=CARTESIAN_POINT('Ctrl Pts',(0.716291984561752,1.06503948076655,2.19850252336627));
#25935=CARTESIAN_POINT('Ctrl Pts',(0.686471316299909,1.10137391770637,2.20111937371216));
#25936=CARTESIAN_POINT('Ctrl Pts',(0.648183040045466,1.11712500025644,2.20373622405805));
#25937=CARTESIAN_POINT('Ctrl Pts',(0.609894763791023,1.13287608280652,2.20635307440395));
#25938=CARTESIAN_POINT('Ctrl Pts',(0.563138879543981,1.12804381096685,2.20896992474984));
#25939=CARTESIAN_POINT('Ctrl Pts',(0.528881281579892,1.10479503290036,2.21158677509573));
#25940=CARTESIAN_POINT('Ctrl Pts',(0.49503980248944,1.0818286521973,2.21417183918447));
#25941=CARTESIAN_POINT('Ctrl Pts',(0.473394826320348,1.04089044984514,2.2167569032732));
#25942=CARTESIAN_POINT('Ctrl Pts',(0.473352235667534,0.999991049382066,
2.21934196736194));
#25943=CARTESIAN_POINT('Origin',(0.6,1.,2.15));
#25944=CARTESIAN_POINT('',(0.473682079464411,1.00008273769678,2.26934196736194));
#25945=CARTESIAN_POINT('',(0.473732170341016,0.999958186567598,2.25565803263806));
#25946=CARTESIAN_POINT('',(0.47355,1.,2.15));
#25947=CARTESIAN_POINT('Ctrl Pts',(0.473732170341016,0.999958186567598,
2.25565803263806));
#25948=CARTESIAN_POINT('Ctrl Pts',(0.47380378639699,1.0235579489136,2.25417789949394));
#25949=CARTESIAN_POINT('Ctrl Pts',(0.480162569358453,1.04719354904427,2.25269776634982));
#25950=CARTESIAN_POINT('Ctrl Pts',(0.492561799143745,1.06705892706426,2.25121763320569));
#25951=CARTESIAN_POINT('Ctrl Pts',(0.514483427533268,1.1021805791598,2.2486007828598));
#25952=CARTESIAN_POINT('Ctrl Pts',(0.555286068051798,1.12551740614607,2.24598393251391));
#25953=CARTESIAN_POINT('Ctrl Pts',(0.596673331802579,1.12660489722647,2.24336708216802));
#25954=CARTESIAN_POINT('Ctrl Pts',(0.63806059555336,1.12769238830687,2.24075023182212));
#25955=CARTESIAN_POINT('Ctrl Pts',(0.680032482536391,1.10653054348142,2.23813338147623));
#25956=CARTESIAN_POINT('Ctrl Pts',(0.703768299652422,1.07260858560646,2.23551653113034));
#25957=CARTESIAN_POINT('Ctrl Pts',(0.727504116768454,1.0386866277315,2.23289968078445));
#25958=CARTESIAN_POINT('Ctrl Pts',(0.733003864017485,0.992004556807043,
2.23028283043855));
#25959=CARTESIAN_POINT('Ctrl Pts',(0.717801389391014,0.953495168290641,
2.22766598009266));
#25960=CARTESIAN_POINT('Ctrl Pts',(0.702598914764542,0.914985779774238,
2.22504912974677));
#25961=CARTESIAN_POINT('Ctrl Pts',(0.666694218262566,0.884649073665893,
2.22243227940087));
#25962=CARTESIAN_POINT('Ctrl Pts',(0.626187392572728,0.876088389616529,
2.21981542905498));
#25963=CARTESIAN_POINT('Ctrl Pts',(0.58568056688289,0.867527705567165,2.21719857870909));
#25964=CARTESIAN_POINT('Ctrl Pts',(0.540571612005191,0.880743043576783,
2.2145817283632));
#25965=CARTESIAN_POINT('Ctrl Pts',(0.511087919517129,0.909808488978038,
2.21196487801731));
#25966=CARTESIAN_POINT('Ctrl Pts',(0.487401800053794,0.933158604039368,
2.20986259622422));
#25967=CARTESIAN_POINT('Ctrl Pts',(0.473800111710378,0.966738263555599,
2.20776031443114));
#25968=CARTESIAN_POINT('Ctrl Pts',(0.473504867419963,1.00010483506638,2.20565803263806));
#25969=CARTESIAN_POINT('Ctrl Pts',(0.473352235667534,0.999991049382066,
2.21934196736194));
#25970=CARTESIAN_POINT('Ctrl Pts',(0.473351711967774,0.99948814546325,2.2193737536191));
#25971=CARTESIAN_POINT('Ctrl Pts',(0.473354454431116,0.998985247411069,
2.21940553987625));
#25972=CARTESIAN_POINT('Ctrl Pts',(0.473360480544096,0.998482388709186,
2.21943732613341));
#25973=CARTESIAN_POINT('Ctrl Pts',(0.473856589153524,0.95708380687781,2.2220541764793));
#25974=CARTESIAN_POINT('Ctrl Pts',(0.496608118053516,0.915951927508368,
2.22467102682519));
#25975=CARTESIAN_POINT('Ctrl Pts',(0.531413011239654,0.893530774346426,
2.22728787717109));
#25976=CARTESIAN_POINT('Ctrl Pts',(0.566217904425792,0.871109621184485,
2.22990472751698));
#25977=CARTESIAN_POINT('Ctrl Pts',(0.613076161898077,0.867399194230046,
2.23252157786287));
#25978=CARTESIAN_POINT('Ctrl Pts',(0.650975984015301,0.88406329282086,2.23513842820876));
#25979=CARTESIAN_POINT('Ctrl Pts',(0.688875806132525,0.900727391411673,
2.23775527855466));
#25980=CARTESIAN_POINT('Ctrl Pts',(0.717817192894688,0.93776601554774,2.24037212890055));
#25981=CARTESIAN_POINT('Ctrl Pts',(0.724822482446523,0.978570606314872,
2.24298897924644));
#25982=CARTESIAN_POINT('Ctrl Pts',(0.731827771998358,1.019375197082,2.24560582959233));
#25983=CARTESIAN_POINT('Ctrl Pts',(0.716896964339864,1.0639457544802,2.24822267993823));
#25984=CARTESIAN_POINT('Ctrl Pts',(0.686725211124828,1.09229630994494,2.25083953028412));
#25985=CARTESIAN_POINT('Ctrl Pts',(0.656553457909791,1.12064686540969,2.25345638063001));
#25986=CARTESIAN_POINT('Ctrl Pts',(0.611140759138212,1.13277741894098,2.25607323097591));
#25987=CARTESIAN_POINT('Ctrl Pts',(0.570850708712658,1.12324848776292,2.2586900813218));
#25988=CARTESIAN_POINT('Ctrl Pts',(0.530560658287105,1.11371955658487,2.26130693166769));
#25989=CARTESIAN_POINT('Ctrl Pts',(0.495393256207577,1.08253114069748,2.26392378201358));
#25990=CARTESIAN_POINT('Ctrl Pts',(0.481117983672093,1.04366849332961,2.26654063235948));
#25991=CARTESIAN_POINT('Ctrl Pts',(0.476024096576591,1.02980102162761,2.26747441069363));
#25992=CARTESIAN_POINT('Ctrl Pts',(0.473590398662461,1.01495639211521,2.26840818902779));
#25993=CARTESIAN_POINT('Ctrl Pts',(0.473682079464411,1.00008273769678,2.26934196736194));
#25994=CARTESIAN_POINT('Origin',(0.6,1.,2.15));
#25995=CARTESIAN_POINT('',(0.473597863174539,0.999893075682974,2.31934196736194));
#25996=CARTESIAN_POINT('',(0.473373733146151,0.999953562449677,2.30565803263806));
#25997=CARTESIAN_POINT('',(0.47355,1.,2.15));
#25998=CARTESIAN_POINT('Ctrl Pts',(0.473373733146151,0.999953562449677,
2.30565803263806));
#25999=CARTESIAN_POINT('Ctrl Pts',(0.473559114374899,1.03866557284283,2.30321233490263));
#26000=CARTESIAN_POINT('Ctrl Pts',(0.492644288253083,1.07753593829701,2.3007666371672));
#26001=CARTESIAN_POINT('Ctrl Pts',(0.523476045360312,1.10091555973398,2.29832093943176));
#26002=CARTESIAN_POINT('Ctrl Pts',(0.556465442652399,1.12593131272659,2.29570408908587));
#26003=CARTESIAN_POINT('Ctrl Pts',(0.602903027909946,1.1332123395264,2.29308723873998));
#26004=CARTESIAN_POINT('Ctrl Pts',(0.641965643116553,1.11949373110512,2.29047038839408));
#26005=CARTESIAN_POINT('Ctrl Pts',(0.681028258323161,1.10577512268384,2.28785353804819));
#26006=CARTESIAN_POINT('Ctrl Pts',(0.712715903478828,1.07105687904148,2.2852366877023));
#26007=CARTESIAN_POINT('Ctrl Pts',(0.722819458161278,1.03090707843903,2.28261983735641));
#26008=CARTESIAN_POINT('Ctrl Pts',(0.732923012843728,0.990757277836576,
2.28000298701051));
#26009=CARTESIAN_POINT('Ctrl Pts',(0.72144247705296,0.945175920274039,2.27738613666462));
#26010=CARTESIAN_POINT('Ctrl Pts',(0.693525861372284,0.914602225692484,
2.27476928631873));
#26011=CARTESIAN_POINT('Ctrl Pts',(0.665609245691608,0.88402853111093,2.27215243597284));
#26012=CARTESIAN_POINT('Ctrl Pts',(0.621256550121025,0.868462499510358,
2.26953558562694));
#26013=CARTESIAN_POINT('Ctrl Pts',(0.580356049616192,0.874884125818288,
2.26691873528105));
#26014=CARTESIAN_POINT('Ctrl Pts',(0.539455549111359,0.881305752126219,
2.26430188493516));
#26015=CARTESIAN_POINT('Ctrl Pts',(0.502007243672275,0.909715036342652,
2.26168503458927));
#26016=CARTESIAN_POINT('Ctrl Pts',(0.484803399082991,0.947372917053277,
2.25906818424337));
#26017=CARTESIAN_POINT('Ctrl Pts',(0.477330328981013,0.963730887562828,
2.2579314670416));
#26018=CARTESIAN_POINT('Ctrl Pts',(0.473677170422209,0.981833968538321,
2.25679474983983));
#26019=CARTESIAN_POINT('Ctrl Pts',(0.473732170341016,0.999958186567598,
2.25565803263806));
#26020=CARTESIAN_POINT('Ctrl Pts',(0.473682079464411,1.00008273769678,2.26934196736194));
#26021=CARTESIAN_POINT('Ctrl Pts',(0.473847327881654,0.973273986038867,
2.27102503937368));
#26022=CARTESIAN_POINT('Ctrl Pts',(0.4822169290695,0.946370939387992,2.27270811138542));
#26023=CARTESIAN_POINT('Ctrl Pts',(0.498001477210419,0.924925552697152,
2.27439118339715));
#26024=CARTESIAN_POINT('Ctrl Pts',(0.522543386275672,0.891582138280912,
2.27700803374305));
#26025=CARTESIAN_POINT('Ctrl Pts',(0.565010347397619,0.871432188296782,
2.27962488408894));
#26026=CARTESIAN_POINT('Ctrl Pts',(0.606359670709474,0.873511167531032,
2.28224173443483));
#26027=CARTESIAN_POINT('Ctrl Pts',(0.64770899402133,0.875590146765282,2.28485858478073));
#26028=CARTESIAN_POINT('Ctrl Pts',(0.687940679523094,0.899898055217912,
2.28747543512662));
#26029=CARTESIAN_POINT('Ctrl Pts',(0.709014360624521,0.935534961978321,
2.29009228547251));
#26030=CARTESIAN_POINT('Ctrl Pts',(0.730088041725949,0.971171868738729,
2.2927091358184));
#26031=CARTESIAN_POINT('Ctrl Pts',(0.73200371842704,1.01813777380691,2.2953259861643));
#26032=CARTESIAN_POINT('Ctrl Pts',(0.713902379672349,1.05537255954882,2.29794283651019));
#26033=CARTESIAN_POINT('Ctrl Pts',(0.695801040917658,1.09260734529072,2.30055968685608));
#26034=CARTESIAN_POINT('Ctrl Pts',(0.657682686707185,1.12011101170634,2.30317653720197));
#26035=CARTESIAN_POINT('Ctrl Pts',(0.616640037917562,1.12555068124487,2.30579338754787));
#26036=CARTESIAN_POINT('Ctrl Pts',(0.57559738912794,1.1309903507834,2.30841023789376));
#26037=CARTESIAN_POINT('Ctrl Pts',(0.531630445759169,1.11436602344484,2.31102708823965));
#26038=CARTESIAN_POINT('Ctrl Pts',(0.504454512281174,1.08313206166147,2.31364393858554));
#26039=CARTESIAN_POINT('Ctrl Pts',(0.484729877635794,1.06046205898416,2.31554328151101));
#26040=CARTESIAN_POINT('Ctrl Pts',(0.473850812735054,1.03009564368688,2.31744262443648));
#26041=CARTESIAN_POINT('Ctrl Pts',(0.473597863174539,0.999893075682974,
2.31934196736194));
#26042=CARTESIAN_POINT('Origin',(0.6,1.,2.15));
#26043=CARTESIAN_POINT('',(0.473395817154925,1.00006080538999,2.36934196736194));
#26044=CARTESIAN_POINT('',(0.473630671680838,1.00010094048498,2.35565803263806));
#26045=CARTESIAN_POINT('',(0.47355,1.,2.15));
#26046=CARTESIAN_POINT('',(0.695811615272236,1.08252112989365,2.4));
#26047=CARTESIAN_POINT('Ctrl Pts',(0.473395817154925,1.00006080538999,2.36934196736194));
#26048=CARTESIAN_POINT('Ctrl Pts',(0.473632259557073,0.962556436040281,
2.37171076053695));
#26049=CARTESIAN_POINT('Ctrl Pts',(0.491389033274771,0.924867297705602,
2.37407955371196));
#26050=CARTESIAN_POINT('Ctrl Pts',(0.520582501482215,0.901356555443706,
2.37644834688697));
#26051=CARTESIAN_POINT('Ctrl Pts',(0.552833074551427,0.875383796542954,
2.37906519723286));
#26052=CARTESIAN_POINT('Ctrl Pts',(0.59904103097391,0.866714403531687,2.38168204757875));
#26053=CARTESIAN_POINT('Ctrl Pts',(0.638485120164714,0.879318631335514,
2.38429889792465));
#26054=CARTESIAN_POINT('Ctrl Pts',(0.677929209355517,0.891922859139342,
2.38691574827054));
#26055=CARTESIAN_POINT('Ctrl Pts',(0.710609431314642,0.925800707758264,
2.38953259861643));
#26056=CARTESIAN_POINT('Ctrl Pts',(0.721864159102138,0.965573527992604,
2.39214944896232));
#26057=CARTESIAN_POINT('Ctrl Pts',(0.733118886889633,1.00534634822694,2.39476629930821));
#26058=CARTESIAN_POINT('Ctrl Pts',(0.7229481205055,1.0510141400767,2.39738314965411));
#26059=CARTESIAN_POINT('Ctrl Pts',(0.695811615272236,1.08252112989365,2.4));
#26060=CARTESIAN_POINT('',(0.50401104110406,1.08263520219401,2.4));
#26061=CARTESIAN_POINT('Origin',(0.6,1.,2.4));
#26062=CARTESIAN_POINT('Ctrl Pts',(0.504010178078501,1.08263575731581,2.4));
#26063=CARTESIAN_POINT('Ctrl Pts',(0.529836321312633,1.11242104812743,2.3975091839613));
#26064=CARTESIAN_POINT('Ctrl Pts',(0.57074030629072,1.12936968375571,2.3950183679226));
#26065=CARTESIAN_POINT('Ctrl Pts',(0.610030393987409,1.12624202648756,2.3925275518839));
#26066=CARTESIAN_POINT('Ctrl Pts',(0.651308544594168,1.12295611099769,2.389910701538));
#26067=CARTESIAN_POINT('Ctrl Pts',(0.690805340696773,1.09751079590418,2.38729385119211));
#26068=CARTESIAN_POINT('Ctrl Pts',(0.710833835900798,1.0612825699207,2.38467700084622));
#26069=CARTESIAN_POINT('Ctrl Pts',(0.730862331104824,1.02505434393722,2.38206015050033));
#26070=CARTESIAN_POINT('Ctrl Pts',(0.73142252541027,0.978043207063774,2.37944330015443));
#26071=CARTESIAN_POINT('Ctrl Pts',(0.712251088485857,0.941346462423258,
2.37682644980854));
#26072=CARTESIAN_POINT('Ctrl Pts',(0.693079651561443,0.904649717782742,
2.37420959946265));
#26073=CARTESIAN_POINT('Ctrl Pts',(0.654176583407171,0.878267365375156,
2.37159274911676));
#26074=CARTESIAN_POINT('Ctrl Pts',(0.612992655582392,0.874020946237636,
2.36897589877086));
#26075=CARTESIAN_POINT('Ctrl Pts',(0.571808727757614,0.869774527100117,
2.36635904842497));
#26076=CARTESIAN_POINT('Ctrl Pts',(0.52834394026233,0.887664041232664,2.36374219807908));
#26077=CARTESIAN_POINT('Ctrl Pts',(0.502085278312862,0.919672004499943,
2.36112534773319));
#26078=CARTESIAN_POINT('Ctrl Pts',(0.483798106092066,0.941963130294246,
2.35930290936814));
#26079=CARTESIAN_POINT('Ctrl Pts',(0.473856023642611,0.971101801466951,
2.3574804710031));
#26080=CARTESIAN_POINT('Ctrl Pts',(0.473630671680838,1.00010094048498,2.35565803263806));
#26081=CARTESIAN_POINT('Origin',(-0.6,1.,2.15));
#26082=CARTESIAN_POINT('',(-0.726251764241557,0.999995816438242,2.01934196736194));
#26083=CARTESIAN_POINT('',(-0.726377624507173,0.999839605165841,2.00565803263806));
#26084=CARTESIAN_POINT('',(-0.72645,1.,2.15));
#26085=CARTESIAN_POINT('',(-0.695811615272238,1.08252112989365,2.));
#26086=CARTESIAN_POINT('Ctrl Pts',(-0.726377624507173,0.999839605165841,
2.00565803263806));
#26087=CARTESIAN_POINT('Ctrl Pts',(-0.726114592834244,1.02975025674996,
2.00377202175871));
#26088=CARTESIAN_POINT('Ctrl Pts',(-0.715369380269338,1.05981347843636,
2.00188601087935));
#26089=CARTESIAN_POINT('Ctrl Pts',(-0.695811615272238,1.08252112989365,
2.));
#26090=CARTESIAN_POINT('',(-0.504011038081522,1.08263519664064,2.));
#26091=CARTESIAN_POINT('Origin',(-0.6,1.,2.));
#26092=CARTESIAN_POINT('Ctrl Pts',(-0.504010174669748,1.08263575197435,
2.));
#26093=CARTESIAN_POINT('Ctrl Pts',(-0.529836317100857,1.11242103949754,
2.0024908160387));
#26094=CARTESIAN_POINT('Ctrl Pts',(-0.570740304630068,1.12936968846467,
2.0049816320774));
#26095=CARTESIAN_POINT('Ctrl Pts',(-0.610030394063595,1.12624203395227,
2.0074724481161));
#26096=CARTESIAN_POINT('Ctrl Pts',(-0.651308546495077,1.12295612135759,
2.010089298462));
#26097=CARTESIAN_POINT('Ctrl Pts',(-0.690805343523631,1.09751079747805,
2.01270614880789));
#26098=CARTESIAN_POINT('Ctrl Pts',(-0.710833838996196,1.06128256888394,
2.01532299915378));
#26099=CARTESIAN_POINT('Ctrl Pts',(-0.721087117546352,1.04273608746385,
2.01666265522317));
#26100=CARTESIAN_POINT('Ctrl Pts',(-0.72623820261666,1.02136365505003,2.01800231129255));
#26101=CARTESIAN_POINT('Ctrl Pts',(-0.726251764241557,0.999995816438242,
2.01934196736194));
#26102=CARTESIAN_POINT('Origin',(-0.6,1.,2.15));
#26103=CARTESIAN_POINT('',(-0.7265819818033,0.99992222657182,2.06934196736194));
#26104=CARTESIAN_POINT('',(-0.726608486751216,1.0000625869776,2.05565803263806));
#26105=CARTESIAN_POINT('',(-0.72645,1.,2.15));
#26106=CARTESIAN_POINT('Ctrl Pts',(-0.726608486751216,1.0000625869776,2.05565803263806));
#26107=CARTESIAN_POINT('Ctrl Pts',(-0.726631053637245,1.00377931196893,
2.05542330751329));
#26108=CARTESIAN_POINT('Ctrl Pts',(-0.726481239616099,1.00749417780353,
2.05518858238852));
#26109=CARTESIAN_POINT('Ctrl Pts',(-0.726153054400444,1.01119320003794,
2.05495385726375));
#26110=CARTESIAN_POINT('Ctrl Pts',(-0.722494257346049,1.0524320219281,2.05233700691785));
#26111=CARTESIAN_POINT('Ctrl Pts',(-0.696665580577272,1.09170163174089,
2.04972015657196));
#26112=CARTESIAN_POINT('Ctrl Pts',(-0.660248783717448,1.1113984599152,2.04710330622607));
#26113=CARTESIAN_POINT('Ctrl Pts',(-0.623831986857623,1.13109528808951,
2.04448645588018));
#26114=CARTESIAN_POINT('Ctrl Pts',(-0.576827069906751,1.13121933462535,
2.04186960553428));
#26115=CARTESIAN_POINT('Ctrl Pts',(-0.540311843519016,1.11170438339395,
2.03925275518839));
#26116=CARTESIAN_POINT('Ctrl Pts',(-0.503796617131281,1.09218943216256,
2.0366359048425));
#26117=CARTESIAN_POINT('Ctrl Pts',(-0.477771081306684,1.05303548316395,
2.03401905449661));
#26118=CARTESIAN_POINT('Ctrl Pts',(-0.473904915961309,1.01182046061616,
2.03140220415071));
#26119=CARTESIAN_POINT('Ctrl Pts',(-0.470038750615934,0.970605438068375,
2.02878535380482));
#26120=CARTESIAN_POINT('Ctrl Pts',(-0.48833195574978,0.927329341971419,
2.02616850345893));
#26121=CARTESIAN_POINT('Ctrl Pts',(-0.520582517234745,0.901356578046236,
2.02355165311303));
#26122=CARTESIAN_POINT('Ctrl Pts',(-0.55283307871971,0.875383814121054,
2.02093480276714));
#26123=CARTESIAN_POINT('Ctrl Pts',(-0.599040996555793,0.866714382367644,
2.01831795242125));
#26124=CARTESIAN_POINT('Ctrl Pts',(-0.63848510046728,0.879318623815634,
2.01570110207536));
#26125=CARTESIAN_POINT('Ctrl Pts',(-0.677929204378768,0.891922865263625,
2.01308425172946));
#26126=CARTESIAN_POINT('Ctrl Pts',(-0.710609494365659,0.925800779913016,
2.01046740138357));
#26127=CARTESIAN_POINT('Ctrl Pts',(-0.721864223397342,0.965573598616285,
2.00785055103768));
#26128=CARTESIAN_POINT('Ctrl Pts',(-0.725007467784426,0.976681435046254,
2.00711971157114));
#26129=CARTESIAN_POINT('Ctrl Pts',(-0.726479550710055,0.988249065107503,
2.0063888721046));
#26130=CARTESIAN_POINT('Ctrl Pts',(-0.726377624507173,0.999839605165841,
2.00565803263806));
#26131=CARTESIAN_POINT('Ctrl Pts',(-0.726251764241557,0.999995816438242,
2.01934196736194));
#26132=CARTESIAN_POINT('Ctrl Pts',(-0.726264693552367,0.979624258543708,
2.02061916163845));
#26133=CARTESIAN_POINT('Ctrl Pts',(-0.721608007468156,0.959256876063438,
2.02189635591495));
#26134=CARTESIAN_POINT('Ctrl Pts',(-0.712251090996448,0.941346462433457,
2.02317355019146));
#26135=CARTESIAN_POINT('Ctrl Pts',(-0.693079653607559,0.904649717885772,
2.02579040053735));
#26136=CARTESIAN_POINT('Ctrl Pts',(-0.654176584913204,0.878267362099087,
2.02840725088324));
#26137=CARTESIAN_POINT('Ctrl Pts',(-0.612992656110291,0.874020942267452,
2.03102410122914));
#26138=CARTESIAN_POINT('Ctrl Pts',(-0.571808727307379,0.869774522435818,
2.03364095157503));
#26139=CARTESIAN_POINT('Ctrl Pts',(-0.528343938395909,0.887664038559235,
2.03625780192092));
#26140=CARTESIAN_POINT('Ctrl Pts',(-0.502085275739541,0.919672002962672,
2.03887465226682));
#26141=CARTESIAN_POINT('Ctrl Pts',(-0.475826613083173,0.951679967366109,
2.04149150261271));
#26142=CARTESIAN_POINT('Ctrl Pts',(-0.466774076681907,0.997806380049565,
2.0441083529586));
#26143=CARTESIAN_POINT('Ctrl Pts',(-0.478988530498336,1.03736537794115,
2.04672520330449));
#26144=CARTESIAN_POINT('Ctrl Pts',(-0.491202984314765,1.07692437583273,
2.04934205365039));
#26145=CARTESIAN_POINT('Ctrl Pts',(-0.52468442834889,1.10991595893243,2.05195890399628));
#26146=CARTESIAN_POINT('Ctrl Pts',(-0.564418571222927,1.12154744492272,
2.05457575434217));
#26147=CARTESIAN_POINT('Ctrl Pts',(-0.604152714096964,1.13317893091301,
2.05719260468806));
#26148=CARTESIAN_POINT('Ctrl Pts',(-0.650139555810913,1.12345031979389,
2.05980945503396));
#26149=CARTESIAN_POINT('Ctrl Pts',(-0.681758464159146,1.09672345837341,
2.06242630537985));
#26150=CARTESIAN_POINT('Ctrl Pts',(-0.709612009894941,1.07317938630266,
2.06473152604055));
#26151=CARTESIAN_POINT('Ctrl Pts',(-0.726315897827418,1.03644450458023,
2.06703674670125));
#26152=CARTESIAN_POINT('Ctrl Pts',(-0.7265819818033,0.99992222657182,2.06934196736194));
#26153=CARTESIAN_POINT('Origin',(-0.6,1.,2.15));
#26154=CARTESIAN_POINT('',(-0.726430664085926,1.00010891291408,2.11934196736194));
#26155=CARTESIAN_POINT('',(-0.726259449807842,1.00002674766465,2.10565803263806));
#26156=CARTESIAN_POINT('',(-0.72645,1.,2.15));
#26157=CARTESIAN_POINT('Ctrl Pts',(-0.726259449807842,1.00002674766465,
2.10565803263806));
#26158=CARTESIAN_POINT('Ctrl Pts',(-0.726296436394794,1.01916777993272,
2.10445774292198));
#26159=CARTESIAN_POINT('Ctrl Pts',(-0.722205040678573,1.0382938070189,2.1032574532059));
#26160=CARTESIAN_POINT('Ctrl Pts',(-0.713902369187372,1.05537255449598,
2.10205716348981));
#26161=CARTESIAN_POINT('Ctrl Pts',(-0.695801032091435,1.09260733676896,
2.09944031314392));
#26162=CARTESIAN_POINT('Ctrl Pts',(-0.657682681356665,1.12011100048129,
2.09682346279803));
#26163=CARTESIAN_POINT('Ctrl Pts',(-0.616640036366223,1.12555066958795,
2.09420661245214));
#26164=CARTESIAN_POINT('Ctrl Pts',(-0.57559739137578,1.13099033869461,2.09158976210624));
#26165=CARTESIAN_POINT('Ctrl Pts',(-0.531630452129665,1.1143660131956,2.08897291176035));
#26166=CARTESIAN_POINT('Ctrl Pts',(-0.504454521120231,1.08313205416568,
2.08635606141446));
#26167=CARTESIAN_POINT('Ctrl Pts',(-0.477278590110797,1.05189809513576,
2.08373921106857));
#26168=CARTESIAN_POINT('Ctrl Pts',(-0.466893667338043,1.00605450257494,
2.08112236072267));
#26169=CARTESIAN_POINT('Ctrl Pts',(-0.477956467154043,0.966158450016923,
2.07850551037678));
#26170=CARTESIAN_POINT('Ctrl Pts',(-0.489019266970043,0.926262397458909,
2.07588866003089));
#26171=CARTESIAN_POINT('Ctrl Pts',(-0.521529789374798,0.892313884903708,
2.07327180968499));
#26172=CARTESIAN_POINT('Ctrl Pts',(-0.560909946303062,0.879535118270141,
2.0706549593391));
#26173=CARTESIAN_POINT('Ctrl Pts',(-0.600290103231324,0.866756351636574,
2.06803810899321));
#26174=CARTESIAN_POINT('Ctrl Pts',(-0.646539894683095,0.875147330924641,
2.06542125864732));
#26175=CARTESIAN_POINT('Ctrl Pts',(-0.678920331738974,0.900946837552442,
2.06280440830142));
#26176=CARTESIAN_POINT('Ctrl Pts',(-0.708396322180238,0.924432191052708,
2.0604222830803));
#26177=CARTESIAN_POINT('Ctrl Pts',(-0.726379465045821,0.962343129588992,
2.05804015785918));
#26178=CARTESIAN_POINT('Ctrl Pts',(-0.726608486751216,1.0000625869776,2.05565803263806));
#26179=CARTESIAN_POINT('Ctrl Pts',(-0.7265819818033,0.99992222657182,2.06934196736194));
#26180=CARTESIAN_POINT('Ctrl Pts',(-0.726617952184381,0.99498498729039,
2.06965359704714));
#26181=CARTESIAN_POINT('Ctrl Pts',(-0.726353524983949,0.990051633299336,
2.06996522673233));
#26182=CARTESIAN_POINT('Ctrl Pts',(-0.725775636014574,0.985155277281126,
2.07027685641753));
#26183=CARTESIAN_POINT('Ctrl Pts',(-0.720922924539255,0.944039069331128,
2.07289370676342));
#26184=CARTESIAN_POINT('Ctrl Pts',(-0.693966526606102,0.905531765152948,
2.07551055710931));
#26185=CARTESIAN_POINT('Ctrl Pts',(-0.656994118794319,0.886900347913169,
2.0781274074552));
#26186=CARTESIAN_POINT('Ctrl Pts',(-0.620021710982536,0.868268930673389,
2.0807442578011));
#26187=CARTESIAN_POINT('Ctrl Pts',(-0.573033293292122,0.86951340037201,
2.08336110814699));
#26188=CARTESIAN_POINT('Ctrl Pts',(-0.537098976133817,0.890075798227289,
2.08597795849288));
#26189=CARTESIAN_POINT('Ctrl Pts',(-0.501164658975514,0.910638196082568,
2.08859480883878));
#26190=CARTESIAN_POINT('Ctrl Pts',(-0.476284442349319,0.950518522094504,
2.09121165918467));
#26191=CARTESIAN_POINT('Ctrl Pts',(-0.473614938940181,0.991833925232179,
2.09382850953056));
#26192=CARTESIAN_POINT('Ctrl Pts',(-0.470945435531044,1.03314932836985,
2.09644535987645));
#26193=CARTESIAN_POINT('Ctrl Pts',(-0.490486645338963,1.07589980863327,
2.09906221022235));
#26194=CARTESIAN_POINT('Ctrl Pts',(-0.523476043451828,1.10091556225217,
2.10167906056824));
#26195=CARTESIAN_POINT('Ctrl Pts',(-0.556465441564692,1.12593131587107,
2.10429591091413));
#26196=CARTESIAN_POINT('Ctrl Pts',(-0.6029030279825,1.13321234284545,2.10691276126002));
#26197=CARTESIAN_POINT('Ctrl Pts',(-0.64196564416317,1.11949373408075,2.10952961160592));
#26198=CARTESIAN_POINT('Ctrl Pts',(-0.68102826034384,1.10577512531604,2.11214646195181));
#26199=CARTESIAN_POINT('Ctrl Pts',(-0.712715906287371,1.07105688081224,
2.1147633122977));
#26200=CARTESIAN_POINT('Ctrl Pts',(-0.722819461221189,1.03090707921019,
2.1173801626436));
#26201=CARTESIAN_POINT('Ctrl Pts',(-0.725344277841846,1.02087388920281,
2.11803409754971));
#26202=CARTESIAN_POINT('Ctrl Pts',(-0.72652123370157,1.01050151499351,2.11868803245583));
#26203=CARTESIAN_POINT('Ctrl Pts',(-0.726430664085926,1.00010891291408,
2.11934196736194));
#26204=CARTESIAN_POINT('Origin',(-0.6,1.,2.15));
#26205=CARTESIAN_POINT('',(-0.726298666832045,0.999928563942421,2.16934196736194));
#26206=CARTESIAN_POINT('',(-0.72652403561687,0.999901036843312,2.15565803263806));
#26207=CARTESIAN_POINT('',(-0.72645,1.,2.15));
#26208=CARTESIAN_POINT('Ctrl Pts',(-0.72652403561687,0.999901036843312,
2.15565803263806));
#26209=CARTESIAN_POINT('Ctrl Pts',(-0.726228629089082,1.03425627916229,
2.15349217833067));
#26210=CARTESIAN_POINT('Ctrl Pts',(-0.711697061286474,1.06883177008057,
2.15132632402327));
#26211=CARTESIAN_POINT('Ctrl Pts',(-0.686725203134716,1.09229630144258,
2.14916046971588));
#26212=CARTESIAN_POINT('Ctrl Pts',(-0.65655345269935,1.12064685429431,2.14654361936999));
#26213=CARTESIAN_POINT('Ctrl Pts',(-0.611140758111187,1.13277740670372,
2.1439267690241));
#26214=CARTESIAN_POINT('Ctrl Pts',(-0.570850711397976,1.12324847640543,
2.1413099186782));
#26215=CARTESIAN_POINT('Ctrl Pts',(-0.530560664684765,1.11371954610715,
2.13869306833231));
#26216=CARTESIAN_POINT('Ctrl Pts',(-0.495393265846508,1.08253113310118,
2.13607621798642));
#26217=CARTESIAN_POINT('Ctrl Pts',(-0.481117994625666,1.04366848931044,
2.13345936764053));
#26218=CARTESIAN_POINT('Ctrl Pts',(-0.466842723404823,1.00480584551971,
2.13084251729463));
#26219=CARTESIAN_POINT('Ctrl Pts',(-0.473459579801396,0.958268970944215,
2.12822566694874));
#26220=CARTESIAN_POINT('Ctrl Pts',(-0.498001486606679,0.924925559606287,
2.12560881660285));
#26221=CARTESIAN_POINT('Ctrl Pts',(-0.522543393411961,0.89158214826836,
2.12299196625695));
#26222=CARTESIAN_POINT('Ctrl Pts',(-0.565010350625955,0.871432200167998,
2.12037511591106));
#26223=CARTESIAN_POINT('Ctrl Pts',(-0.606359670125879,0.873511179199166,
2.11775826556517));
#26224=CARTESIAN_POINT('Ctrl Pts',(-0.647708989625804,0.875590158230334,
2.11514141521928));
#26225=CARTESIAN_POINT('Ctrl Pts',(-0.687940671411661,0.899898064393031,
2.11252456487338));
#26226=CARTESIAN_POINT('Ctrl Pts',(-0.709014350576037,0.935534967891196,
2.10990771452749));
#26227=CARTESIAN_POINT('Ctrl Pts',(-0.72042201256801,0.954826034551965,
2.10849115389768));
#26228=CARTESIAN_POINT('Ctrl Pts',(-0.726215798894061,0.977436840943303,
2.10707459326787));
#26229=CARTESIAN_POINT('Ctrl Pts',(-0.726259449807842,1.00002674766465,
2.10565803263806));
#26230=CARTESIAN_POINT('Ctrl Pts',(-0.726430664085926,1.00010891291408,
2.11934196736194));
#26231=CARTESIAN_POINT('Ctrl Pts',(-0.726158801404701,0.968913454634673,
2.12130488280172));
#26232=CARTESIAN_POINT('Ctrl Pts',(-0.714466288285182,0.937535739321086,
2.1232677982415));
#26233=CARTESIAN_POINT('Ctrl Pts',(-0.693525863703029,0.914602223563998,
2.12523071368127));
#26234=CARTESIAN_POINT('Ctrl Pts',(-0.665609247326942,0.884028528220152,
2.12784756402716));
#26235=CARTESIAN_POINT('Ctrl Pts',(-0.621256550650662,0.868462496232756,
2.13046441437306));
#26236=CARTESIAN_POINT('Ctrl Pts',(-0.580356049126553,0.874884122700947,
2.13308126471895));
#26237=CARTESIAN_POINT('Ctrl Pts',(-0.539455547602445,0.881305749169137,
2.13569811506484));
#26238=CARTESIAN_POINT('Ctrl Pts',(-0.502007241230509,0.909715034092914,
2.13831496541074));
#26239=CARTESIAN_POINT('Ctrl Pts',(-0.484803396212605,0.947372915741768,
2.14093181575663));
#26240=CARTESIAN_POINT('Ctrl Pts',(-0.467599551194702,0.985030797390621,
2.14354866610252));
#26241=CARTESIAN_POINT('Ctrl Pts',(-0.470640167530832,1.03193727576455,
2.14616551644841));
#26242=CARTESIAN_POINT('Ctrl Pts',(-0.492561796466562,1.06705892873532,
2.14878236679431));
#26243=CARTESIAN_POINT('Ctrl Pts',(-0.514483425402293,1.10218058170609,
2.1513992171402));
#26244=CARTESIAN_POINT('Ctrl Pts',(-0.555286066937625,1.1255174092737,2.15401606748609));
#26245=CARTESIAN_POINT('Ctrl Pts',(-0.596673331719711,1.12660490038116,
2.15663291783198));
#26246=CARTESIAN_POINT('Ctrl Pts',(-0.638060596501796,1.12769239148863,
2.15924976817788));
#26247=CARTESIAN_POINT('Ctrl Pts',(-0.680032484530636,1.10653054613594,
2.16186661852377));
#26248=CARTESIAN_POINT('Ctrl Pts',(-0.703768302238105,1.07260858741574,
2.16448346886966));
#26249=CARTESIAN_POINT('Ctrl Pts',(-0.718457772313683,1.05161518395829,
2.16610296836709));
#26250=CARTESIAN_POINT('Ctrl Pts',(-0.726162745631061,1.02573459982654,
2.16772246786452));
#26251=CARTESIAN_POINT('Ctrl Pts',(-0.726298666832045,0.999928563942421,
2.16934196736194));
#26252=CARTESIAN_POINT('Origin',(-0.6,1.,2.15));
#26253=CARTESIAN_POINT('',(-0.726647750450984,0.999991049383163,2.21934196736194));
#26254=CARTESIAN_POINT('',(-0.726495137942383,1.00010483507083,2.20565803263806));
#26255=CARTESIAN_POINT('',(-0.72645,1.,2.15));
#26256=CARTESIAN_POINT('Ctrl Pts',(-0.726495137942383,1.00010483507083,
2.20565803263806));
#26257=CARTESIAN_POINT('Ctrl Pts',(-0.726567403912713,1.00827186063272,
2.20514346408525));
#26258=CARTESIAN_POINT('Ctrl Pts',(-0.725842471048314,1.01642611993573,
2.20462889553244));
#26259=CARTESIAN_POINT('Ctrl Pts',(-0.72427309126162,1.02441448062962,2.20411432697963));
#26260=CARTESIAN_POINT('Ctrl Pts',(-0.716291973847398,1.06503947477424,
2.20149747663373));
#26261=CARTESIAN_POINT('Ctrl Pts',(-0.686471308333041,1.10137390836652,
2.19888062628784));
#26262=CARTESIAN_POINT('Ctrl Pts',(-0.648183035606218,1.11712498946538,
2.19626377594195));
#26263=CARTESIAN_POINT('Ctrl Pts',(-0.609894762879395,1.13287607056424,
2.19364692559606));
#26264=CARTESIAN_POINT('Ctrl Pts',(-0.563138882940105,1.12804379916968,
2.19103007525017));
#26265=CARTESIAN_POINT('Ctrl Pts',(-0.52888128813228,1.10479502324521,2.18841322490427));
#26266=CARTESIAN_POINT('Ctrl Pts',(-0.494623693324455,1.08154624732075,
2.18579637455838));
#26267=CARTESIAN_POINT('Ctrl Pts',(-0.472864383648094,1.03988096686638,
2.18317952421249));
#26268=CARTESIAN_POINT('Ctrl Pts',(-0.473360492211805,0.998482388849106,
2.18056267386659));
#26269=CARTESIAN_POINT('Ctrl Pts',(-0.473856600775515,0.957083810831832,
2.1779458235207));
#26270=CARTESIAN_POINT('Ctrl Pts',(-0.496608127579297,0.915951935251654,
2.17532897317481));
#26271=CARTESIAN_POINT('Ctrl Pts',(-0.531413017558768,0.893530784155595,
2.17271212282892));
#26272=CARTESIAN_POINT('Ctrl Pts',(-0.56621790753824,0.871109633059536,
2.17009527248302));
#26273=CARTESIAN_POINT('Ctrl Pts',(-0.613076160693402,0.867399206447596,
2.16747842213713));
#26274=CARTESIAN_POINT('Ctrl Pts',(-0.650975979318758,0.884063303502809,
2.16486157179124));
#26275=CARTESIAN_POINT('Ctrl Pts',(-0.688875797944115,0.900727400558021,
2.16224472144534));
#26276=CARTESIAN_POINT('Ctrl Pts',(-0.717817182039666,0.937766021280388,
2.15962787109945));
#26277=CARTESIAN_POINT('Ctrl Pts',(-0.724822470946157,0.978570608288594,
2.15701102075356));
#26278=CARTESIAN_POINT('Ctrl Pts',(-0.726029783985795,0.985602996335628,
2.15656002471506));
#26279=CARTESIAN_POINT('Ctrl Pts',(-0.726585548144894,0.9927472416251,2.15610902867656));
#26280=CARTESIAN_POINT('Ctrl Pts',(-0.72652403561687,0.999901036843312,
2.15565803263806));
#26281=CARTESIAN_POINT('Ctrl Pts',(-0.726298666832045,0.999928563942421,
2.16934196736194));
#26282=CARTESIAN_POINT('Ctrl Pts',(-0.726382372399933,0.984036202243351,
2.17033931821041));
#26283=CARTESIAN_POINT('Ctrl Pts',(-0.723595457458582,0.968172113533461,
2.17133666905888));
#26284=CARTESIAN_POINT('Ctrl Pts',(-0.71780139232639,0.95349516713182,2.17233401990734));
#26285=CARTESIAN_POINT('Ctrl Pts',(-0.702598917321108,0.914985777655832,
2.17495087025323));
#26286=CARTESIAN_POINT('Ctrl Pts',(-0.666694219924447,0.884649070791584,
2.17756772059913));
#26287=CARTESIAN_POINT('Ctrl Pts',(-0.626187393225259,0.876088386528911,
2.18018457094502));
#26288=CARTESIAN_POINT('Ctrl Pts',(-0.58568056652607,0.867527702266238,
2.18280142129091));
#26289=CARTESIAN_POINT('Ctrl Pts',(-0.540571610524354,0.880743040605142,
2.1854182716368));
#26290=CARTESIAN_POINT('Ctrl Pts',(-0.511087917301621,0.909808486730647,
2.1880351219827));
#26291=CARTESIAN_POINT('Ctrl Pts',(-0.481604224078888,0.938873932856152,
2.19065197232859));
#26292=CARTESIAN_POINT('Ctrl Pts',(-0.467745793635136,0.983789486768259,
2.19326882267448));
#26293=CARTESIAN_POINT('Ctrl Pts',(-0.475726910909899,1.02441448020301,
2.19588567302037));
#26294=CARTESIAN_POINT('Ctrl Pts',(-0.483708028184661,1.06503947363776,
2.19850252336627));
#26295=CARTESIAN_POINT('Ctrl Pts',(-0.513528693177939,1.10137390659515,
2.20111937371216));
#26296=CARTESIAN_POINT('Ctrl Pts',(-0.551816965235723,1.11712498741877,
2.20373622405805));
#26297=CARTESIAN_POINT('Ctrl Pts',(-0.590105237293507,1.1328760682424,2.20635307440395));
#26298=CARTESIAN_POINT('Ctrl Pts',(-0.636861116415798,1.12804379693225,
2.20896992474984));
#26299=CARTESIAN_POINT('Ctrl Pts',(-0.671118710625013,1.10479502141404,
2.21158677509573));
#26300=CARTESIAN_POINT('Ctrl Pts',(-0.704960186006201,1.0818286432283,2.21417183918447));
#26301=CARTESIAN_POINT('Ctrl Pts',(-0.726605159802828,1.04089044536347,
2.21675690327321));
#26302=CARTESIAN_POINT('Ctrl Pts',(-0.726647750450984,0.999991049383163,
2.21934196736194));
#26303=CARTESIAN_POINT('Origin',(-0.6,1.,2.15));
#26304=CARTESIAN_POINT('',(-0.726317906690824,1.0000827376849,2.26934196736194));
#26305=CARTESIAN_POINT('',(-0.726267835011577,0.999958186565595,2.25565803263806));
#26306=CARTESIAN_POINT('',(-0.72645,1.,2.15));
#26307=CARTESIAN_POINT('Ctrl Pts',(-0.726267835011577,0.999958186565595,
2.25565803263806));
#26308=CARTESIAN_POINT('Ctrl Pts',(-0.726196218952626,1.02355794991214,
2.25417789949394));
#26309=CARTESIAN_POINT('Ctrl Pts',(-0.719837435721701,1.04719355104496,
2.25269776634982));
#26310=CARTESIAN_POINT('Ctrl Pts',(-0.707438205410818,1.06705892990714,
2.25121763320569));
#26311=CARTESIAN_POINT('Ctrl Pts',(-0.685516576092059,1.10218058349167,
2.2486007828598));
#26312=CARTESIAN_POINT('Ctrl Pts',(-0.644713933843695,1.12551741146695,
2.24598393251391));
#26313=CARTESIAN_POINT('Ctrl Pts',(-0.603326668338405,1.12660490259339,
2.24336708216802));
#26314=CARTESIAN_POINT('Ctrl Pts',(-0.561939402833115,1.12769239371984,
2.24075023182213));
#26315=CARTESIAN_POINT('Ctrl Pts',(-0.519967514070899,1.10653054799744,
2.23813338147623));
#26316=CARTESIAN_POINT('Ctrl Pts',(-0.496231695948683,1.0726085886845,2.23551653113034));
#26317=CARTESIAN_POINT('Ctrl Pts',(-0.472495877826467,1.03868662937157,
2.23289968078445));
#26318=CARTESIAN_POINT('Ctrl Pts',(-0.466996130344251,0.992004556468098,
2.23028283043855));
#26319=CARTESIAN_POINT('Ctrl Pts',(-0.482198605615172,0.9534951663192,2.22766598009266));
#26320=CARTESIAN_POINT('Ctrl Pts',(-0.497401080886093,0.914985776170301,
2.22504912974677));
#26321=CARTESIAN_POINT('Ctrl Pts',(-0.533305778910153,0.884649068775973,
2.22243227940087));
#26322=CARTESIAN_POINT('Ctrl Pts',(-0.573812606317149,0.876088384363716,
2.21981542905498));
#26323=CARTESIAN_POINT('Ctrl Pts',(-0.614319433724146,0.867527699951458,
2.21719857870909));
#26324=CARTESIAN_POINT('Ctrl Pts',(-0.659428390514079,0.88074303852127,
2.2145817283632));
#26325=CARTESIAN_POINT('Ctrl Pts',(-0.688912084252003,0.909808485154657,
2.21196487801731));
#26326=CARTESIAN_POINT('Ctrl Pts',(-0.712598204719431,0.933158601205837,
2.20986259622422));
#26327=CARTESIAN_POINT('Ctrl Pts',(-0.72619989363945,0.96673826214558,2.20776031443114));
#26328=CARTESIAN_POINT('Ctrl Pts',(-0.726495137942383,1.00010483507083,
2.20565803263806));
#26329=CARTESIAN_POINT('Ctrl Pts',(-0.726647750450984,0.999991049383163,
2.21934196736194));
#26330=CARTESIAN_POINT('Ctrl Pts',(-0.726648274150687,0.999488145519468,
2.2193737536191));
#26331=CARTESIAN_POINT('Ctrl Pts',(-0.726645531687645,0.998985247522407,
2.21940553987625));
#26332=CARTESIAN_POINT('Ctrl Pts',(-0.726639505575326,0.99848238887564,
2.21943732613341));
#26333=CARTESIAN_POINT('Ctrl Pts',(-0.726143397020285,0.957083811581739,
2.2220541764793));
#26334=CARTESIAN_POINT('Ctrl Pts',(-0.703391870614066,0.915951936720223,
2.22467102682519));
#26335=CARTESIAN_POINT('Ctrl Pts',(-0.668586981242762,0.893530786015975,
2.22728787717108));
#26336=CARTESIAN_POINT('Ctrl Pts',(-0.633782091871458,0.871109635311727,
2.22990472751698));
#26337=CARTESIAN_POINT('Ctrl Pts',(-0.586923839535069,0.867399208764748,
2.23252157786287));
#26338=CARTESIAN_POINT('Ctrl Pts',(-0.549024021571972,0.884063305528724,
2.23513842820877));
#26339=CARTESIAN_POINT('Ctrl Pts',(-0.511124203608875,0.9007274022927,2.23775527855466));
#26340=CARTESIAN_POINT('Ctrl Pts',(-0.48218282001907,0.93776602236763,2.24037212890055));
#26341=CARTESIAN_POINT('Ctrl Pts',(-0.475177531234974,0.978570608662929,
2.24298897924644));
#26342=CARTESIAN_POINT('Ctrl Pts',(-0.468172242450878,1.01937519495823,
2.24560582959233));
#26343=CARTESIAN_POINT('Ctrl Pts',(-0.483103048472492,1.06394574747389,
2.24822267993823));
#26344=CARTESIAN_POINT('Ctrl Pts',(-0.513274798380673,1.09229629983004,
2.25083953028412));
#26345=CARTESIAN_POINT('Ctrl Pts',(-0.543446548288854,1.12064685218619,
2.25345638063001));
#26346=CARTESIAN_POINT('Ctrl Pts',(-0.588859242083601,1.13277740438282,
2.25607323097591));
#26347=CARTESIAN_POINT('Ctrl Pts',(-0.629149288092737,1.1232484742514,2.2586900813218));
#26348=CARTESIAN_POINT('Ctrl Pts',(-0.669439334101873,1.11371954411997,
2.26130693166769));
#26349=CARTESIAN_POINT('Ctrl Pts',(-0.704606732325397,1.08253113166048,
2.26392378201358));
#26350=CARTESIAN_POINT('Ctrl Pts',(-0.718882003296907,1.04366848854818,
2.26654063235948));
#26351=CARTESIAN_POINT('Ctrl Pts',(-0.723975889834331,1.0298010183647,2.26747441069363));
#26352=CARTESIAN_POINT('Ctrl Pts',(-0.726409587482227,1.01495639047621,
2.26840818902779));
#26353=CARTESIAN_POINT('Ctrl Pts',(-0.726317906690824,1.0000827376849,2.26934196736194));
#26354=CARTESIAN_POINT('Origin',(-0.6,1.,2.15));
#26355=CARTESIAN_POINT('',(-0.72640212307541,0.999893075304641,2.31934196736194));
#26356=CARTESIAN_POINT('',(-0.726626272216059,0.999953562434948,2.30565803263806));
#26357=CARTESIAN_POINT('',(-0.72645,1.,2.15));
#26358=CARTESIAN_POINT('Ctrl Pts',(-0.726626272216059,0.999953562434948,
2.30565803263806));
#26359=CARTESIAN_POINT('Ctrl Pts',(-0.726440890977488,1.03866557446413,
2.30321233490263));
#26360=CARTESIAN_POINT('Ctrl Pts',(-0.707355716298753,1.0775359415853,2.3007666371672));
#26361=CARTESIAN_POINT('Ctrl Pts',(-0.676523957886503,1.10091556401805,
2.29832093943176));
#26362=CARTESIAN_POINT('Ctrl Pts',(-0.643534559198068,1.12593131807613,
2.29570408908587));
#26363=CARTESIAN_POINT('Ctrl Pts',(-0.597096971966626,1.13321234517294,
2.29308723873998));
#26364=CARTESIAN_POINT('Ctrl Pts',(-0.558034355102894,1.11949373616741,
2.29047038839408));
#26365=CARTESIAN_POINT('Ctrl Pts',(-0.518971738239162,1.10577512716188,
2.28785353804819));
#26366=CARTESIAN_POINT('Ctrl Pts',(-0.487284091743139,1.07105688205399,
2.2852366877023));
#26367=CARTESIAN_POINT('Ctrl Pts',(-0.477180536633045,1.03090707975097,
2.28261983735641));
#26368=CARTESIAN_POINT('Ctrl Pts',(-0.467076981522952,0.990757277447954,
2.28000298701051));
#26369=CARTESIAN_POINT('Ctrl Pts',(-0.478557517798788,0.945175917949804,
2.27738613666462));
#26370=CARTESIAN_POINT('Ctrl Pts',(-0.506474134662531,0.914602222071399,
2.27476928631873));
#26371=CARTESIAN_POINT('Ctrl Pts',(-0.534390751526274,0.884028526192994,
2.27215243597283));
#26372=CARTESIAN_POINT('Ctrl Pts',(-0.578743448977924,0.868462493934334,
2.26953558562694));
#26373=CARTESIAN_POINT('Ctrl Pts',(-0.6196439512168,0.874884120514905,2.26691873528105));
#26374=CARTESIAN_POINT('Ctrl Pts',(-0.660544453455676,0.881305747095476,
2.26430188493516));
#26375=CARTESIAN_POINT('Ctrl Pts',(-0.697992760481779,0.909715032515278,
2.26168503458927));
#26376=CARTESIAN_POINT('Ctrl Pts',(-0.715196605800255,0.947372914822063,
2.25906818424337));
#26377=CARTESIAN_POINT('Ctrl Pts',(-0.722669676218981,0.96373088602496,
2.2579314670416));
#26378=CARTESIAN_POINT('Ctrl Pts',(-0.72632283493267,0.981833967767914,
2.25679474983983));
#26379=CARTESIAN_POINT('Ctrl Pts',(-0.726267835011577,0.999958186565595,
2.25565803263806));
#26380=CARTESIAN_POINT('Ctrl Pts',(-0.726317906690824,1.0000827376849,2.26934196736194));
#26381=CARTESIAN_POINT('Ctrl Pts',(-0.726152658292592,0.973273988959771,
2.27102503937368));
#26382=CARTESIAN_POINT('Ctrl Pts',(-0.717783058022956,0.946370945252116,
2.27270811138542));
#26383=CARTESIAN_POINT('Ctrl Pts',(-0.701998511611248,0.924925560916646,
2.27439118339715));
#26384=CARTESIAN_POINT('Ctrl Pts',(-0.677456605234583,0.891582150162549,
2.27700803374305));
#26385=CARTESIAN_POINT('Ctrl Pts',(-0.634989648761757,0.871432202419483,
2.27962488408894));
#26386=CARTESIAN_POINT('Ctrl Pts',(-0.593640329984797,0.873511181412128,
2.28224173443483));
#26387=CARTESIAN_POINT('Ctrl Pts',(-0.552291011207836,0.875590160404774,
2.28485858478073));
#26388=CARTESIAN_POINT('Ctrl Pts',(-0.512059330126741,0.899898066133132,
2.28747543512662));
#26389=CARTESIAN_POINT('Ctrl Pts',(-0.490985651329738,0.935534969012601,
2.29009228547251));
#26390=CARTESIAN_POINT('Ctrl Pts',(-0.469911972532735,0.971171871892071,
2.2927091358184));
#26391=CARTESIAN_POINT('Ctrl Pts',(-0.467996296019824,1.01813777192265,
2.29532598616429));
#26392=CARTESIAN_POINT('Ctrl Pts',(-0.486097632801175,1.0553725535377,2.29794283651019));
#26393=CARTESIAN_POINT('Ctrl Pts',(-0.504198969582526,1.09260733515275,
2.30055968685608));
#26394=CARTESIAN_POINT('Ctrl Pts',(-0.54231731965814,1.12011099835227,2.30317653720197));
#26395=CARTESIAN_POINT('Ctrl Pts',(-0.583359963928024,1.12555066737707,
2.30579338754787));
#26396=CARTESIAN_POINT('Ctrl Pts',(-0.624402608197908,1.13099033640186,
2.30841023789376));
#26397=CARTESIAN_POINT('Ctrl Pts',(-0.668369546662063,1.11436601125193,
2.31102708823965));
#26398=CARTESIAN_POINT('Ctrl Pts',(-0.695545477203344,1.08313205274415,
2.31364393858554));
#26399=CARTESIAN_POINT('Ctrl Pts',(-0.71527010971722,1.0604620524443,2.31554328151101));
#26400=CARTESIAN_POINT('Ctrl Pts',(-0.726149173523156,1.0300956400971,2.31744262443648));
#26401=CARTESIAN_POINT('Ctrl Pts',(-0.72640212307541,0.999893075304641,
2.31934196736194));
#26402=CARTESIAN_POINT('Origin',(-0.6,1.,2.15));
#26403=CARTESIAN_POINT('',(-0.726604172280256,1.00006079745576,2.36934196736194));
#26404=CARTESIAN_POINT('',(-0.726369333664333,1.00010094057762,2.35565803263806));
#26405=CARTESIAN_POINT('',(-0.72645,1.,2.15));
#26406=CARTESIAN_POINT('',(-0.504188384727764,1.08252112989365,2.4));
#26407=CARTESIAN_POINT('Ctrl Pts',(-0.726604172280256,1.00006079745576,
2.36934196736194));
#26408=CARTESIAN_POINT('Ctrl Pts',(-0.7263677230741,0.962556440882506,2.37171076053695));
#26409=CARTESIAN_POINT('Ctrl Pts',(-0.708610935503227,0.92486733001342,
2.37407955371196));
#26410=CARTESIAN_POINT('Ctrl Pts',(-0.679417479773344,0.901356582338566,
2.37644834688697));
#26411=CARTESIAN_POINT('Ctrl Pts',(-0.647166920488327,0.875383817458018,
2.37906519723286));
#26412=CARTESIAN_POINT('Ctrl Pts',(-0.600959009984164,0.866714378341853,
2.38168204757875));
#26413=CARTESIAN_POINT('Ctrl Pts',(-0.561514903279023,0.879318622378776,
2.38429889792465));
#26414=CARTESIAN_POINT('Ctrl Pts',(-0.522070796573882,0.891922866415699,
2.38691574827054));
#26415=CARTESIAN_POINT('Ctrl Pts',(-0.489390493667762,0.92580079360571,
2.38953259861643));
#26416=CARTESIAN_POINT('Ctrl Pts',(-0.478135764397917,0.965573612020961,
2.39214944896232));
#26417=CARTESIAN_POINT('Ctrl Pts',(-0.466881035128071,1.00534643043621,
2.39476629930821));
#26418=CARTESIAN_POINT('Ctrl Pts',(-0.4770518794945,1.0510141400767,2.39738314965411));
#26419=CARTESIAN_POINT('Ctrl Pts',(-0.504188384727764,1.08252112989365,
2.4));
#26420=CARTESIAN_POINT('',(-0.695988964037237,1.08263519275223,2.4));
#26421=CARTESIAN_POINT('Origin',(-0.6,1.,2.4));
#26422=CARTESIAN_POINT('Ctrl Pts',(-0.695989827719566,1.0826357482344,2.4));
#26423=CARTESIAN_POINT('Ctrl Pts',(-0.670163685851419,1.11242103345157,
2.3975091839613));
#26424=CARTESIAN_POINT('Ctrl Pts',(-0.629259696534257,1.12936969176545,
2.3950183679226));
#26425=CARTESIAN_POINT('Ctrl Pts',(-0.589969605883147,1.12624203918417,
2.3925275518839));
#26426=CARTESIAN_POINT('Ctrl Pts',(-0.548691452172472,1.12295612861833,
2.38991070153801));
#26427=CARTESIAN_POINT('Ctrl Pts',(-0.509194654494277,1.09751079858255,
2.38729385119211));
#26428=CARTESIAN_POINT('Ctrl Pts',(-0.489166158833217,1.06128256815865,
2.38467700084622));
#26429=CARTESIAN_POINT('Ctrl Pts',(-0.469137663172157,1.02505433773475,
2.38206015050033));
#26430=CARTESIAN_POINT('Ctrl Pts',(-0.468577469528232,0.978043206922726,
2.37944330015444));
#26431=CARTESIAN_POINT('Ctrl Pts',(-0.487748907242888,0.94134646243954,
2.37682644980854));
#26432=CARTESIAN_POINT('Ctrl Pts',(-0.506920344957544,0.904649717956355,
2.37420959946265));
#26433=CARTESIAN_POINT('Ctrl Pts',(-0.54582341403078,0.878267359802006,
2.37159274911676));
#26434=CARTESIAN_POINT('Ctrl Pts',(-0.587007343519609,0.874020939484002,
2.36897589877086));
#26435=CARTESIAN_POINT('Ctrl Pts',(-0.628191273008439,0.869774519165998,
2.36635904842497));
#26436=CARTESIAN_POINT('Ctrl Pts',(-0.671656062912861,0.887664036684341,
2.36374219807908));
#26437=CARTESIAN_POINT('Ctrl Pts',(-0.697914726064929,0.919672001884272,
2.36112534773319));
#26438=CARTESIAN_POINT('Ctrl Pts',(-0.716201899123246,0.94196312902452,
2.35930290936814));
#26439=CARTESIAN_POINT('Ctrl Pts',(-0.726143981825042,0.971101800838385,
2.3574804710031));
#26440=CARTESIAN_POINT('Ctrl Pts',(-0.726369333664333,1.00010094057762,
2.35565803263806));
#26441=CARTESIAN_POINT('Origin',(0.6,1.,2.51042117235887));
#26442=CARTESIAN_POINT('',(0.44550661348391,1.00007637252271,2.03957882764113));
#26443=CARTESIAN_POINT('',(0.445941879748409,0.999994887077554,2.03542117235887));
#26444=CARTESIAN_POINT('',(0.4457,1.,2.51042117235887));
#26445=CARTESIAN_POINT('',(0.639851384185725,0.850935057178149,2.));
#26446=CARTESIAN_POINT('Ctrl Pts',(0.445941879748409,0.999994887077554,
2.03542117235887));
#26447=CARTESIAN_POINT('Ctrl Pts',(0.445958427563446,1.02606888540753,2.03408151628949));
#26448=CARTESIAN_POINT('Ctrl Pts',(0.464522119816522,1.10309173428669,2.03012500987421));
#26449=CARTESIAN_POINT('Ctrl Pts',(0.585586764715563,1.18108624726655,2.02355165311303));
#26450=CARTESIAN_POINT('Ctrl Pts',(0.74321627607811,1.11199512704675,2.01570110207536));
#26451=CARTESIAN_POINT('Ctrl Pts',(0.772174135599484,0.94213024790789,2.00785055103768));
#26452=CARTESIAN_POINT('Ctrl Pts',(0.688870364005735,0.864039910406678,
2.00261685034589));
#26453=CARTESIAN_POINT('Ctrl Pts',(0.639851384185725,0.850935057178149,
2.));
#26454=CARTESIAN_POINT('',(0.560048264277831,0.850698128346977,2.));
#26455=CARTESIAN_POINT('Origin',(0.6,1.,2.));
#26456=CARTESIAN_POINT('Ctrl Pts',(0.44550661348391,1.00007637252271,2.03957882764113));
#26457=CARTESIAN_POINT('Ctrl Pts',(0.445479076365182,1.00461168797626,2.03934410251636));
#26458=CARTESIAN_POINT('Ctrl Pts',(0.447699955244927,1.0596817411018,2.03649252704569));
#26459=CARTESIAN_POINT('Ctrl Pts',(0.513561617374857,1.15981701056446,2.03102410122914));
#26460=CARTESIAN_POINT('Ctrl Pts',(0.685634169421134,1.1602711276025,2.02317355019146));
#26461=CARTESIAN_POINT('Ctrl Pts',(0.780906782004492,1.01693885807272,2.01532299915378));
#26462=CARTESIAN_POINT('Ctrl Pts',(0.715015266367875,0.861059909554376,
2.00759848242329));
#26463=CARTESIAN_POINT('Ctrl Pts',(0.606562024823064,0.838426846369365,
2.0024908160387));
#26464=CARTESIAN_POINT('Ctrl Pts',(0.560047775926799,0.850696975355777,
2.));
#26465=CARTESIAN_POINT('Origin',(0.6,1.,2.51042117235887));
#26466=CARTESIAN_POINT('',(0.445932524475483,1.00003263872856,2.08957882764113));
#26467=CARTESIAN_POINT('',(0.445538932974414,0.999905097479817,2.08542117235887));
#26468=CARTESIAN_POINT('',(0.4457,1.,2.51042117235887));
#26469=CARTESIAN_POINT('Ctrl Pts',(0.445538932974414,0.999905097479817,
2.08542117235887));
#26470=CARTESIAN_POINT('Ctrl Pts',(0.445863620600756,1.04447123493477,2.08311595169817));
#26471=CARTESIAN_POINT('Ctrl Pts',(0.489384741719965,1.14018208017193,2.07819388069158));
#26472=CARTESIAN_POINT('Ctrl Pts',(0.651047898079357,1.17438225782416,2.0706549593391));
#26473=CARTESIAN_POINT('Ctrl Pts',(0.773614618887169,1.05360877841752,2.06280440830142));
#26474=CARTESIAN_POINT('Ctrl Pts',(0.740475677832241,0.884752178886651,
2.05495385726374));
#26475=CARTESIAN_POINT('Ctrl Pts',(0.581362560637208,0.819263360725568,
2.04710330622607));
#26476=CARTESIAN_POINT('Ctrl Pts',(0.463250898323639,0.899361552534091,
2.04059241125778));
#26477=CARTESIAN_POINT('Ctrl Pts',(0.445926103479307,0.975136595316218,
2.03669836663538));
#26478=CARTESIAN_POINT('Ctrl Pts',(0.445941879748409,0.999994887077554,
2.03542117235887));
#26479=CARTESIAN_POINT('Ctrl Pts',(0.445932524475483,1.00003263872856,2.08957882764113));
#26480=CARTESIAN_POINT('Ctrl Pts',(0.445887391771903,1.02338938965811,2.08837853792505));
#26481=CARTESIAN_POINT('Ctrl Pts',(0.461764469489331,1.09760988546538,2.08456139786307));
#26482=CARTESIAN_POINT('Ctrl Pts',(0.57612672137744,1.18012607114374,2.07812740745521));
#26483=CARTESIAN_POINT('Ctrl Pts',(0.737078048375186,1.11926881624917,2.07027685641753));
#26484=CARTESIAN_POINT('Ctrl Pts',(0.775094502137202,0.951447557128672,
2.06242630537985));
#26485=CARTESIAN_POINT('Ctrl Pts',(0.656082084236305,0.827171040068,2.05457575434217));
#26486=CARTESIAN_POINT('Ctrl Pts',(0.491836019895195,0.856969773295158,
2.04695992842926));
#26487=CARTESIAN_POINT('Ctrl Pts',(0.445786075962011,0.954049389522044,
2.04196095286225));
#26488=CARTESIAN_POINT('Ctrl Pts',(0.44550661348391,1.00007637252271,2.03957882764113));
#26489=CARTESIAN_POINT('Origin',(0.6,1.,2.51042117235887));
#26490=CARTESIAN_POINT('',(0.445609664942012,0.999879240692409,2.13957882764113));
#26491=CARTESIAN_POINT('',(0.445723577648801,1.00013290047684,2.13542117235887));
#26492=CARTESIAN_POINT('',(0.4457,1.,2.51042117235887));
#26493=CARTESIAN_POINT('Ctrl Pts',(0.445723577648801,1.00013290047684,2.13542117235887));
#26494=CARTESIAN_POINT('Ctrl Pts',(0.445613060502099,1.01281442421482,2.13476723745276));
#26495=CARTESIAN_POINT('Ctrl Pts',(0.45279637409468,1.07612012598108,2.13149645220075));
#26496=CARTESIAN_POINT('Ctrl Pts',(0.539792347657613,1.17143637275151,2.12560881660284));
#26497=CARTESIAN_POINT('Ctrl Pts',(0.70978808601476,1.14478245624706,2.11775826556517));
#26498=CARTESIAN_POINT('Ctrl Pts',(0.781323293607615,0.988284239491303,
2.10990771452749));
#26499=CARTESIAN_POINT('Ctrl Pts',(0.690243392316909,0.842292899938004,
2.10205716348982));
#26500=CARTESIAN_POINT('Ctrl Pts',(0.518231205927094,0.837737224374896,
2.09420661245213));
#26501=CARTESIAN_POINT('Ctrl Pts',(0.448527232502997,0.937309583846461,
2.08866128207516));
#26502=CARTESIAN_POINT('Ctrl Pts',(0.445495040298755,0.993880454536856,
2.08573280204407));
#26503=CARTESIAN_POINT('Ctrl Pts',(0.445538932974414,0.999905097479817,
2.08542117235887));
#26504=CARTESIAN_POINT('Ctrl Pts',(0.445609664942012,0.999879240692409,
2.13957882764113));
#26505=CARTESIAN_POINT('Ctrl Pts',(0.445970133311311,1.04180105694513,2.13741297333374));
#26506=CARTESIAN_POINT('Ctrl Pts',(0.485126633726011,1.13496755094661,2.13263026868045));
#26507=CARTESIAN_POINT('Ctrl Pts',(0.641820162707069,1.17682322770038,2.12523071368128));
#26508=CARTESIAN_POINT('Ctrl Pts',(0.770558701511974,1.06265070285456,2.11738016264359));
#26509=CARTESIAN_POINT('Ctrl Pts',(0.746336141641471,0.892291522696776,
2.10952961160592));
#26510=CARTESIAN_POINT('Ctrl Pts',(0.590875851708506,0.818527896169216,
2.10167906056824));
#26511=CARTESIAN_POINT('Ctrl Pts',(0.466115932152929,0.893907603907564,
2.09502879924665));
#26512=CARTESIAN_POINT('Ctrl Pts',(0.445985789291595,0.972467415629669,
2.09099538827094));
#26513=CARTESIAN_POINT('Ctrl Pts',(0.445932524475483,1.00003263872856,2.08957882764113));
#26514=CARTESIAN_POINT('Origin',(0.6,1.,2.51042117235887));
#26515=CARTESIAN_POINT('',(0.445644927187824,1.00012792448195,2.18957882764113));
#26516=CARTESIAN_POINT('',(0.445884646673086,0.999912830487253,2.18542117235887));
#26517=CARTESIAN_POINT('',(0.4457,1.,2.51042117235887));
#26518=CARTESIAN_POINT('Ctrl Pts',(0.445884646673086,0.999912830487253,
2.18542117235887));
#26519=CARTESIAN_POINT('Ctrl Pts',(0.446050503878428,1.03140252422683,2.18380167286145));
#26520=CARTESIAN_POINT('Ctrl Pts',(0.470644510125523,1.11401244662307,2.17956532301813));
#26521=CARTESIAN_POINT('Ctrl Pts',(0.604772735062981,1.18163868139168,2.17271212282892));
#26522=CARTESIAN_POINT('Ctrl Pts',(0.754140428515542,1.09620871962996,2.16486157179123));
#26523=CARTESIAN_POINT('Ctrl Pts',(0.765271321801097,0.924496491715462,
2.15701102075356));
#26524=CARTESIAN_POINT('Ctrl Pts',(0.628182963406343,0.820497603368372,
2.14916046971588));
#26525=CARTESIAN_POINT('Ctrl Pts',(0.479344005128078,0.872734156235485,
2.14196385358432));
#26526=CARTESIAN_POINT('Ctrl Pts',(0.446055316804476,0.962066789442876,
2.13738408779865));
#26527=CARTESIAN_POINT('Ctrl Pts',(0.445723577648801,1.00013290047684,2.13542117235887));
#26528=CARTESIAN_POINT('Ctrl Pts',(0.445644927187824,1.00012792448195,2.18957882764113));
#26529=CARTESIAN_POINT('Ctrl Pts',(0.445556744991309,1.01009369744184,2.18906425908832));
#26530=CARTESIAN_POINT('Ctrl Pts',(0.450939973182116,1.07064584055842,2.18593284018961));
#26531=CARTESIAN_POINT('Ctrl Pts',(0.530872330435983,1.16803793011858,2.18018457094502));
#26532=CARTESIAN_POINT('Ctrl Pts',(0.702033231237909,1.1503482635805,2.17233401990734));
#26533=CARTESIAN_POINT('Ctrl Pts',(0.781688304564893,0.997822700079642,
2.16448346886966));
#26534=CARTESIAN_POINT('Ctrl Pts',(0.698400986961052,0.847249790637147,
2.15663291783198));
#26535=CARTESIAN_POINT('Ctrl Pts',(0.526865324912526,0.833666900912216,
2.14878236679431));
#26536=CARTESIAN_POINT('Ctrl Pts',(0.450147764311532,0.931848543518796,
2.14309767006402));
#26537=CARTESIAN_POINT('Ctrl Pts',(0.445534604580841,0.991149857098978,
2.14002982367963));
#26538=CARTESIAN_POINT('Ctrl Pts',(0.445609664942012,0.999879240692409,
2.13957882764113));
#26539=CARTESIAN_POINT('Origin',(0.6,1.,2.51042117235887));
#26540=CARTESIAN_POINT('',(0.445922292476226,0.999948977361648,2.23957882764113));
#26541=CARTESIAN_POINT('',(0.445458679031241,0.999989078051821,2.23542117235887));
#26542=CARTESIAN_POINT('',(0.4457,1.,2.51042117235887));
#26543=CARTESIAN_POINT('Ctrl Pts',(0.445458679031242,0.999989078051821,
2.23542117235887));
#26544=CARTESIAN_POINT('Ctrl Pts',(0.445510650069037,1.04989637335789,2.23283610827014));
#26545=CARTESIAN_POINT('Ctrl Pts',(0.498659772012076,1.15041990786983,2.22763419383551));
#26546=CARTESIAN_POINT('Ctrl Pts',(0.669127678863374,1.16803795272366,2.21981542905498));
#26547=CARTESIAN_POINT('Ctrl Pts',(0.778293256865801,1.03502719068774,2.21196487801731));
#26548=CARTESIAN_POINT('Ctrl Pts',(0.727561203441069,0.870603211369231,
2.20411432697963));
#26549=CARTESIAN_POINT('Ctrl Pts',(0.562429230156179,0.822225348280642,
2.19626377594195));
#26550=CARTESIAN_POINT('Ctrl Pts',(0.458106037926808,0.910370419295299,
2.1900327244017));
#26551=CARTESIAN_POINT('Ctrl Pts',(0.445782505348105,0.980520250977966,
2.18641852320734));
#26552=CARTESIAN_POINT('Ctrl Pts',(0.445884646673086,0.999912830487253,
2.18542117235887));
#26553=CARTESIAN_POINT('Ctrl Pts',(0.445922292476226,0.999948977361648,
2.23957882764113));
#26554=CARTESIAN_POINT('Ctrl Pts',(0.446009681621634,1.02874647305155,2.23809869449701));
#26555=CARTESIAN_POINT('Ctrl Pts',(0.467487221018094,1.10857850003564,2.23400171100699));
#26556=CARTESIAN_POINT('Ctrl Pts',(0.595227265578502,1.18163865695784,2.22728787717108));
#26557=CARTESIAN_POINT('Ctrl Pts',(0.748875240939872,1.10417074102503,2.21943732613341));
#26558=CARTESIAN_POINT('Ctrl Pts',(0.769008360762544,0.933280028245809,
2.21158677509573));
#26559=CARTESIAN_POINT('Ctrl Pts',(0.637570764789711,0.822225372195567,
2.20373622405805));
#26560=CARTESIAN_POINT('Ctrl Pts',(0.483262475482066,0.867432276377129,
2.19640024157318));
#26561=CARTESIAN_POINT('Ctrl Pts',(0.446005197603095,0.959412527217309,
2.19168110943421));
#26562=CARTESIAN_POINT('Ctrl Pts',(0.445644927187824,1.00012792448195,2.18957882764113));
#26563=CARTESIAN_POINT('Origin',(0.6,1.,2.51042117235887));
#26564=CARTESIAN_POINT('',(0.445484911225394,0.999943334804163,2.28957882764113));
#26565=CARTESIAN_POINT('',(0.445861169326679,1.00010096027373,2.28542117235887));
#26566=CARTESIAN_POINT('',(0.4457,1.,2.51042117235887));
#26567=CARTESIAN_POINT('Ctrl Pts',(0.445861169326679,1.00010096027373,2.28542117235887));
#26568=CARTESIAN_POINT('Ctrl Pts',(0.445749296272184,1.01825046503264,2.28448739402472));
#26569=CARTESIAN_POINT('Ctrl Pts',(0.457041409544473,1.08712805126299,2.28093676534467));
#26570=CARTESIAN_POINT('Ctrl Pts',(0.558179831669208,1.17682325150234,2.27476928631873));
#26571=CARTESIAN_POINT('Ctrl Pts',(0.724423708785572,1.13241650393702,2.26691873528105));
#26572=CARTESIAN_POINT('Ctrl Pts',(0.779081445955335,0.969255483615749,
2.25906818424337));
#26573=CARTESIAN_POINT('Ctrl Pts',(0.673134684925636,0.833666878534013,
2.25121763320569));
#26574=CARTESIAN_POINT('Ctrl Pts',(0.50159899980171,0.84724977008965,2.24336708216802));
#26575=CARTESIAN_POINT('Ctrl Pts',(0.445736890155226,0.948241381044753,
2.23810159521908));
#26576=CARTESIAN_POINT('Ctrl Pts',(0.445458039989146,0.999375411980858,
2.23545295861603));
#26577=CARTESIAN_POINT('Ctrl Pts',(0.445458679031242,0.999989078051821,
2.23542117235887));
#26578=CARTESIAN_POINT('Ctrl Pts',(0.445484911225394,0.999943334804162,
2.28957882764113));
#26579=CARTESIAN_POINT('Ctrl Pts',(0.445711121771824,1.04718147797272,2.2871331299057));
#26580=CARTESIAN_POINT('Ctrl Pts',(0.493918064875951,1.14536352796849,2.28207058182437));
#26581=CARTESIAN_POINT('Ctrl Pts',(0.660207644220989,1.17143634973614,2.27439118339715));
#26582=CARTESIAN_POINT('Ctrl Pts',(0.776207730757634,1.04434204382826,2.26654063235948));
#26583=CARTESIAN_POINT('Ctrl Pts',(0.734180526190243,0.87748075149375,2.2586900813218));
#26584=CARTESIAN_POINT('Ctrl Pts',(0.571817040388558,0.820497627508739,
2.25083953028412));
#26585=CARTESIAN_POINT('Ctrl Pts',(0.460575165814633,0.904888683245033,
2.24446911239056));
#26586=CARTESIAN_POINT('Ctrl Pts',(0.445855179091712,0.977832988101724,
2.2407155448429));
#26587=CARTESIAN_POINT('Ctrl Pts',(0.445922292476226,0.999948977361648,
2.23957882764113));
#26588=CARTESIAN_POINT('Origin',(0.6,1.,2.51042117235887));
#26589=CARTESIAN_POINT('',(0.445798439227784,1.00012317213786,2.33957882764113));
#26590=CARTESIAN_POINT('',(0.445758404806891,0.999869526120069,2.33542117235887));
#26591=CARTESIAN_POINT('',(0.4457,1.,2.51042117235887));
#26592=CARTESIAN_POINT('Ctrl Pts',(0.445758404806891,0.999869526120069,
2.33542117235887));
#26593=CARTESIAN_POINT('Ctrl Pts',(0.446067065282869,1.03672406343128,2.33352182943341));
#26594=CARTESIAN_POINT('Ctrl Pts',(0.477632210806756,1.12483092984331,2.32900563616205));
#26595=CARTESIAN_POINT('Ctrl Pts',(0.623873281963166,1.1801260959606,2.3218725925448));
#26596=CARTESIAN_POINT('Ctrl Pts',(0.76341449322476,1.07944244879737,2.31402204150712));
#26597=CARTESIAN_POINT('Ctrl Pts',(0.756401707578768,0.907512694301026,
2.30617149046944));
#26598=CARTESIAN_POINT('Ctrl Pts',(0.609124149502328,0.818527871661859,
2.29832093943176));
#26599=CARTESIAN_POINT('Ctrl Pts',(0.472154957249585,0.883517743796439,
2.29140416672824));
#26600=CARTESIAN_POINT('Ctrl Pts',(0.446062812907388,0.967387710919709,
2.28710424437061));
#26601=CARTESIAN_POINT('Ctrl Pts',(0.445861169326679,1.00010096027373,2.28542117235887));
#26602=CARTESIAN_POINT('Ctrl Pts',(0.445798439227784,1.00012317213786,2.33957882764113));
#26603=CARTESIAN_POINT('Ctrl Pts',(0.445678571748812,1.01554817070058,2.33878441566028));
#26604=CARTESIAN_POINT('Ctrl Pts',(0.454838216821075,1.08164530296445,2.33537315333353));
#26605=CARTESIAN_POINT('Ctrl Pts',(0.548952109888326,1.17438223097154,2.3293450406609));
#26606=CARTESIAN_POINT('Ctrl Pts',(0.717297767916034,1.1387683610531,2.32149448962322));
#26607=CARTESIAN_POINT('Ctrl Pts',(0.780449022522885,0.978702297157564,
2.31364393858554));
#26608=CARTESIAN_POINT('Ctrl Pts',(0.681768782849741,0.837737246759644,
2.30579338754786));
#26609=CARTESIAN_POINT('Ctrl Pts',(0.509756619949943,0.842292920851884,
2.29794283651019));
#26610=CARTESIAN_POINT('Ctrl Pts',(0.447051029253845,0.942803275635825,
2.29253798320794));
#26611=CARTESIAN_POINT('Ctrl Pts',(0.445469080763202,0.996637557724894,
2.28974998025159));
#26612=CARTESIAN_POINT('Ctrl Pts',(0.445484911225394,0.999943334804162,
2.28957882764113));
#26613=CARTESIAN_POINT('Origin',(0.6,1.,2.51042117235887));
#26614=CARTESIAN_POINT('',(0.445864724392684,0.99983533609866,2.38957882764113));
#26615=CARTESIAN_POINT('',(0.44551185913013,1.0000741974826,2.38542117235887));
#26616=CARTESIAN_POINT('',(0.4457,1.,2.51042117235887));
#26617=CARTESIAN_POINT('',(0.560148615814278,0.850935057178148,2.4));
#26618=CARTESIAN_POINT('Ctrl Pts',(0.560148615814278,0.850935057178148,
2.4));
#26619=CARTESIAN_POINT('Ctrl Pts',(0.511129635994267,0.864039910406677,
2.39738314965411));
#26620=CARTESIAN_POINT('Ctrl Pts',(0.455839024989005,0.915869990257929,
2.39390942553448));
#26621=CARTESIAN_POINT('Ctrl Pts',(0.445750544275333,0.983186184474914,
2.39043570141486));
#26622=CARTESIAN_POINT('Ctrl Pts',(0.445864724392684,0.99983533609866,2.38957882764113));
#26623=CARTESIAN_POINT('',(0.639951772688379,0.850698147244252,2.4));
#26624=CARTESIAN_POINT('Origin',(0.6,1.,2.4));
#26625=CARTESIAN_POINT('Ctrl Pts',(0.639952262351544,0.850696991672977,
2.4));
#26626=CARTESIAN_POINT('Ctrl Pts',(0.593438030028895,0.838426877605595,
2.3975091839613));
#26627=CARTESIAN_POINT('Ctrl Pts',(0.490251767896999,0.859960628309645,
2.39264957474759));
#26628=CARTESIAN_POINT('Ctrl Pts',(0.445800376826071,0.954309672447724,
2.38778996553388));
#26629=CARTESIAN_POINT('Ctrl Pts',(0.445511859130131,1.0000741974826,2.38542117235887));
#26630=CARTESIAN_POINT('Origin',(-0.6,1.,2.51042117235887));
#26631=CARTESIAN_POINT('',(-0.75449339269049,1.00007637145626,2.03957882764113));
#26632=CARTESIAN_POINT('',(-0.754058103775977,0.999994895029031,2.03542117235887));
#26633=CARTESIAN_POINT('',(-0.7543,1.,2.51042117235887));
#26634=CARTESIAN_POINT('',(-0.560148615814275,0.850935057178149,2.));
#26635=CARTESIAN_POINT('Ctrl Pts',(-0.754058103775977,0.999994895029031,
2.03542117235887));
#26636=CARTESIAN_POINT('Ctrl Pts',(-0.754041555268885,1.02606889659328,
2.03408151628949));
#26637=CARTESIAN_POINT('Ctrl Pts',(-0.735477862467914,1.10309174989979,
2.03012500987421));
#26638=CARTESIAN_POINT('Ctrl Pts',(-0.614413230072635,1.18108614472194,
2.02355165311304));
#26639=CARTESIAN_POINT('Ctrl Pts',(-0.456783762484268,1.11199525865091,
2.01570110207535));
#26640=CARTESIAN_POINT('Ctrl Pts',(-0.427825820216639,0.942129974923708,
2.00785055103768));
#26641=CARTESIAN_POINT('Ctrl Pts',(-0.511129635994264,0.864039910406679,
2.00261685034589));
#26642=CARTESIAN_POINT('Ctrl Pts',(-0.560148615814275,0.850935057178149,
2.));
#26643=CARTESIAN_POINT('',(-0.639951747396791,0.850698134330425,2.));
#26644=CARTESIAN_POINT('Origin',(-0.6,1.,2.));
#26645=CARTESIAN_POINT('Ctrl Pts',(-0.754493392690491,1.00007637145626,
2.03957882764113));
#26646=CARTESIAN_POINT('Ctrl Pts',(-0.754520929823858,1.00461168712382,
2.03934410251636));
#26647=CARTESIAN_POINT('Ctrl Pts',(-0.752300051092223,1.05968174304917,
2.03649252704569));
#26648=CARTESIAN_POINT('Ctrl Pts',(-0.686438388751686,1.15981702310584,
2.03102410122914));
#26649=CARTESIAN_POINT('Ctrl Pts',(-0.514365822072695,1.16027112465931,
2.02317355019146));
#26650=CARTESIAN_POINT('Ctrl Pts',(-0.41909321999119,1.01693887482571,2.01532299915378));
#26651=CARTESIAN_POINT('Ctrl Pts',(-0.484984709990756,0.861059878644944,
2.00759848242329));
#26652=CARTESIAN_POINT('Ctrl Pts',(-0.593437992489385,0.838426856238601,
2.0024908160387));
#26653=CARTESIAN_POINT('Ctrl Pts',(-0.63995223616215,0.850696980524376,
2.));
#26654=CARTESIAN_POINT('Origin',(-0.6,1.,2.51042117235887));
#26655=CARTESIAN_POINT('',(-0.754067482051008,1.00003263870824,2.08957882764113));
#26656=CARTESIAN_POINT('',(-0.754461050156182,0.999905097350985,2.08542117235887));
#26657=CARTESIAN_POINT('',(-0.7543,1.,2.51042117235887));
#26658=CARTESIAN_POINT('Ctrl Pts',(-0.754461050156182,0.999905097350985,
2.08542117235887));
#26659=CARTESIAN_POINT('Ctrl Pts',(-0.754136362473472,1.0444712301837,2.08311595169818));
#26660=CARTESIAN_POINT('Ctrl Pts',(-0.71061524567478,1.14018206615738,2.07819388069158));
#26661=CARTESIAN_POINT('Ctrl Pts',(-0.548952108412014,1.17438223594748,
2.0706549593391));
#26662=CARTESIAN_POINT('Ctrl Pts',(-0.426385398697532,1.05360877753029,
2.06280440830142));
#26663=CARTESIAN_POINT('Ctrl Pts',(-0.459524339782119,0.884752182582313,
2.05495385726375));
#26664=CARTESIAN_POINT('Ctrl Pts',(-0.618637434184013,0.819263396393857,
2.04710330622607));
#26665=CARTESIAN_POINT('Ctrl Pts',(-0.736749089275893,0.89936154319225,
2.04059241125778));
#26666=CARTESIAN_POINT('Ctrl Pts',(-0.754073880704865,0.975136600184218,
2.03669836663538));
#26667=CARTESIAN_POINT('Ctrl Pts',(-0.754058103775977,0.999994895029031,
2.03542117235887));
#26668=CARTESIAN_POINT('Ctrl Pts',(-0.754067482051008,1.00003263870824,
2.08957882764113));
#26669=CARTESIAN_POINT('Ctrl Pts',(-0.754112614754579,1.02338939061779,
2.08837853792505));
#26670=CARTESIAN_POINT('Ctrl Pts',(-0.738235536361179,1.09760988955354,
2.08456139786307));
#26671=CARTESIAN_POINT('Ctrl Pts',(-0.623873279675432,1.18012607896462,
2.0781274074552));
#26672=CARTESIAN_POINT('Ctrl Pts',(-0.462921945732953,1.11926882096942,
2.07027685641753));
#26673=CARTESIAN_POINT('Ctrl Pts',(-0.424905490600427,0.951447555675582,
2.06242630537985));
#26674=CARTESIAN_POINT('Ctrl Pts',(-0.54391791306908,0.827171031659744,
2.05457575434217));
#26675=CARTESIAN_POINT('Ctrl Pts',(-0.708163985289881,0.856969769057042,
2.04695992842926));
#26676=CARTESIAN_POINT('Ctrl Pts',(-0.754213930063824,0.954049386283767,
2.04196095286225));
#26677=CARTESIAN_POINT('Ctrl Pts',(-0.754493392690491,1.00007637145626,
2.03957882764113));
#26678=CARTESIAN_POINT('Origin',(-0.6,1.,2.51042117235887));
#26679=CARTESIAN_POINT('',(-0.754390341602871,0.999879240687419,2.13957882764113));
#26680=CARTESIAN_POINT('',(-0.75427640544451,1.00013290045585,2.13542117235887));
#26681=CARTESIAN_POINT('',(-0.7543,1.,2.51042117235887));
#26682=CARTESIAN_POINT('Ctrl Pts',(-0.75427640544451,1.00013290045585,2.13542117235887));
#26683=CARTESIAN_POINT('Ctrl Pts',(-0.754386922579298,1.01281442280347,
2.13476723745276));
#26684=CARTESIAN_POINT('Ctrl Pts',(-0.747203609773684,1.07612011763199,
2.13149645220075));
#26685=CARTESIAN_POINT('Ctrl Pts',(-0.660207645725328,1.17143635399922,
2.12560881660285));
#26686=CARTESIAN_POINT('Ctrl Pts',(-0.490211926051119,1.14478244030651,
2.11775826556517));
#26687=CARTESIAN_POINT('Ctrl Pts',(-0.418676726208604,0.988284240908056,
2.10990771452749));
#26688=CARTESIAN_POINT('Ctrl Pts',(-0.509756617677689,0.842292916978238,
2.10205716348981));
#26689=CARTESIAN_POINT('Ctrl Pts',(-0.681768784928714,0.837737242612945,
2.09420661245213));
#26690=CARTESIAN_POINT('Ctrl Pts',(-0.75147275106401,0.937309590263154,
2.08866128207516));
#26691=CARTESIAN_POINT('Ctrl Pts',(-0.754504942839462,0.993880455032877,
2.08573280204407));
#26692=CARTESIAN_POINT('Ctrl Pts',(-0.754461050156182,0.999905097350985,
2.08542117235887));
#26693=CARTESIAN_POINT('Ctrl Pts',(-0.75439034160287,0.999879240687419,
2.13957882764113));
#26694=CARTESIAN_POINT('Ctrl Pts',(-0.754029873218229,1.04180105871682,
2.13741297333374));
#26695=CARTESIAN_POINT('Ctrl Pts',(-0.714873371143386,1.13496755666601,
2.13263026868045));
#26696=CARTESIAN_POINT('Ctrl Pts',(-0.558179835520779,1.17682323520091,
2.12523071368127));
#26697=CARTESIAN_POINT('Ctrl Pts',(-0.429441291256411,1.0626507055017,2.1173801626436));
#26698=CARTESIAN_POINT('Ctrl Pts',(-0.453663852157743,0.892291518147041,
2.10952961160592));
#26699=CARTESIAN_POINT('Ctrl Pts',(-0.609124148673025,0.818527888446316,
2.10167906056824));
#26700=CARTESIAN_POINT('Ctrl Pts',(-0.733884073530661,0.893907599452349,
2.09502879924664));
#26701=CARTESIAN_POINT('Ctrl Pts',(-0.754014217234906,0.972467414452767,
2.09099538827094));
#26702=CARTESIAN_POINT('Ctrl Pts',(-0.754067482051008,1.00003263870824,
2.08957882764113));
#26703=CARTESIAN_POINT('Origin',(-0.6,1.,2.51042117235887));
#26704=CARTESIAN_POINT('',(-0.754355079355554,1.00012792448738,2.18957882764113));
#26705=CARTESIAN_POINT('',(-0.754115336434833,0.999912830496762,2.18542117235887));
#26706=CARTESIAN_POINT('',(-0.7543,1.,2.51042117235887));
#26707=CARTESIAN_POINT('Ctrl Pts',(-0.754115336434833,0.999912830496762,
2.18542117235887));
#26708=CARTESIAN_POINT('Ctrl Pts',(-0.753949479247709,1.03140252078477,
2.18380167286145));
#26709=CARTESIAN_POINT('Ctrl Pts',(-0.72935547569638,1.11401243412622,2.17956532301813));
#26710=CARTESIAN_POINT('Ctrl Pts',(-0.595227265459685,1.1816386614837,2.17271212282892));
#26711=CARTESIAN_POINT('Ctrl Pts',(-0.445859588380167,1.09620870908317,
2.16486157179124));
#26712=CARTESIAN_POINT('Ctrl Pts',(-0.434728696312199,0.924496499994273,
2.15701102075356));
#26713=CARTESIAN_POINT('Ctrl Pts',(-0.571817039685625,0.820497623037239,
2.14916046971588));
#26714=CARTESIAN_POINT('Ctrl Pts',(-0.720655981642513,0.872734170194251,
2.14196385358432));
#26715=CARTESIAN_POINT('Ctrl Pts',(-0.753944666324598,0.962066793595335,
2.13738408779865));
#26716=CARTESIAN_POINT('Ctrl Pts',(-0.75427640544451,1.00013290045585,2.13542117235887));
#26717=CARTESIAN_POINT('Ctrl Pts',(-0.754355079355553,1.00012792448738,
2.18957882764113));
#26718=CARTESIAN_POINT('Ctrl Pts',(-0.754443261555807,1.01009369786974,
2.18906425908832));
#26719=CARTESIAN_POINT('Ctrl Pts',(-0.749060033136799,1.07064584355324,
2.18593284018961));
#26720=CARTESIAN_POINT('Ctrl Pts',(-0.669127672494447,1.16803793724193,
2.18018457094502));
#26721=CARTESIAN_POINT('Ctrl Pts',(-0.497966764436741,1.15034826995414,
2.17233401990734));
#26722=CARTESIAN_POINT('Ctrl Pts',(-0.418311687733005,0.997822699987136,
2.16448346886966));
#26723=CARTESIAN_POINT('Ctrl Pts',(-0.501599008867606,0.847249784162188,
2.15663291783199));
#26724=CARTESIAN_POINT('Ctrl Pts',(-0.673134678187691,0.833666893860354,
2.1487823667943));
#26725=CARTESIAN_POINT('Ctrl Pts',(-0.749852242041061,0.931848540630513,
2.14309767006402));
#26726=CARTESIAN_POINT('Ctrl Pts',(-0.754465401967237,0.99114985672403,
2.14002982367963));
#26727=CARTESIAN_POINT('Ctrl Pts',(-0.75439034160287,0.999879240687419,
2.13957882764113));
#26728=CARTESIAN_POINT('Origin',(-0.6,1.,2.51042117235887));
#26729=CARTESIAN_POINT('',(-0.75407771405525,0.999948977359204,2.23957882764113));
#26730=CARTESIAN_POINT('',(-0.754541304029948,0.999989078053162,2.23542117235887));
#26731=CARTESIAN_POINT('',(-0.7543,1.,2.51042117235887));
#26732=CARTESIAN_POINT('Ctrl Pts',(-0.754541304029948,0.999989078053162,
2.23542117235887));
#26733=CARTESIAN_POINT('Ctrl Pts',(-0.754489332997837,1.04989636788915,
2.23283610827014));
#26734=CARTESIAN_POINT('Ctrl Pts',(-0.701340216880369,1.15041989138249,
2.2276341938355));
#26735=CARTESIAN_POINT('Ctrl Pts',(-0.530872328713473,1.16803793430571,
2.21981542905499));
#26736=CARTESIAN_POINT('Ctrl Pts',(-0.421706762676398,1.0350271868484,2.2119648780173));
#26737=CARTESIAN_POINT('Ctrl Pts',(-0.472438810540477,0.870603225552124,
2.20411432697963));
#26738=CARTESIAN_POINT('Ctrl Pts',(-0.637570765725878,0.822225367765818,
2.19626377594195));
#26739=CARTESIAN_POINT('Ctrl Pts',(-0.741893946520544,0.910370429119493,
2.1900327244017));
#26740=CARTESIAN_POINT('Ctrl Pts',(-0.754217477748594,0.980520253113081,
2.18641852320734));
#26741=CARTESIAN_POINT('Ctrl Pts',(-0.754115336434833,0.999912830496762,
2.18542117235887));
#26742=CARTESIAN_POINT('Ctrl Pts',(-0.75407771405525,0.999948977359204,
2.23957882764113));
#26743=CARTESIAN_POINT('Ctrl Pts',(-0.753990324906209,1.02874647427002,
2.23809869449701));
#26744=CARTESIAN_POINT('Ctrl Pts',(-0.732512784599607,1.10857850463897,
2.23400171100699));
#26745=CARTESIAN_POINT('Ctrl Pts',(-0.604772734623643,1.18163866465747,
2.22728787717109));
#26746=CARTESIAN_POINT('Ctrl Pts',(-0.451124752749149,1.10417074544119,
2.21943732613341));
#26747=CARTESIAN_POINT('Ctrl Pts',(-0.43099163207285,0.933280025417337,
2.21158677509573));
#26748=CARTESIAN_POINT('Ctrl Pts',(-0.562429233617627,0.822225364659454,
2.20373622405805));
#26749=CARTESIAN_POINT('Ctrl Pts',(-0.716737529466624,0.867432270757321,
2.19640024157319));
#26750=CARTESIAN_POINT('Ctrl Pts',(-0.753994808925007,0.959412525496741,
2.19168110943421));
#26751=CARTESIAN_POINT('Ctrl Pts',(-0.754355079355553,1.00012792448738,
2.18957882764113));
#26752=CARTESIAN_POINT('Origin',(-0.6,1.,2.51042117235887));
#26753=CARTESIAN_POINT('',(-0.754515095317817,0.999943334786189,2.28957882764113));
#26754=CARTESIAN_POINT('',(-0.754138813779314,1.00010096025924,2.28542117235887));
#26755=CARTESIAN_POINT('',(-0.7543,1.,2.51042117235887));
#26756=CARTESIAN_POINT('Ctrl Pts',(-0.754138813779314,1.00010096025924,
2.28542117235887));
#26757=CARTESIAN_POINT('Ctrl Pts',(-0.754250686820938,1.01825046303266,
2.28448739402472));
#26758=CARTESIAN_POINT('Ctrl Pts',(-0.74295857478395,1.08712804172823,2.28093676534467));
#26759=CARTESIAN_POINT('Ctrl Pts',(-0.641820163748749,1.17682323210921,
2.27476928631873));
#26760=CARTESIAN_POINT('Ctrl Pts',(-0.47557630485125,1.13241648942973,2.26691873528105));
#26761=CARTESIAN_POINT('Ctrl Pts',(-0.420918573673669,0.969255486982105,
2.25906818424337));
#26762=CARTESIAN_POINT('Ctrl Pts',(-0.526865323090207,0.833666896767115,
2.2512176332057));
#26763=CARTESIAN_POINT('Ctrl Pts',(-0.698400989412974,0.847249786831145,
2.24336708216802));
#26764=CARTESIAN_POINT('Ctrl Pts',(-0.75426309293647,0.948241386717884,
2.23810159521908));
#26765=CARTESIAN_POINT('Ctrl Pts',(-0.754541943071973,0.999375412049459,
2.23545295861603));
#26766=CARTESIAN_POINT('Ctrl Pts',(-0.754541304029948,0.999989078053162,
2.23542117235887));
#26767=CARTESIAN_POINT('Ctrl Pts',(-0.754515095317817,0.999943334786189,
2.28957882764113));
#26768=CARTESIAN_POINT('Ctrl Pts',(-0.754288884759399,1.04718147995109,
2.2871331299057));
#26769=CARTESIAN_POINT('Ctrl Pts',(-0.706081939633174,1.1453635341575,2.28207058182437));
#26770=CARTESIAN_POINT('Ctrl Pts',(-0.539792353219763,1.17143635698873,
2.27439118339715));
#26771=CARTESIAN_POINT('Ctrl Pts',(-0.423792261776434,1.04434204571596,
2.26654063235948));
#26772=CARTESIAN_POINT('Ctrl Pts',(-0.465819468119529,0.877480746295693,
2.2586900813218));
#26773=CARTESIAN_POINT('Ctrl Pts',(-0.6281829608073,0.820497619901593,2.25083953028412));
#26774=CARTESIAN_POINT('Ctrl Pts',(-0.73942484009554,0.90488867921255,2.24446911239056));
#26775=CARTESIAN_POINT('Ctrl Pts',(-0.754144827442555,0.977832987161639,
2.2407155448429));
#26776=CARTESIAN_POINT('Ctrl Pts',(-0.75407771405525,0.999948977359204,
2.23957882764113));
#26777=CARTESIAN_POINT('Origin',(-0.6,1.,2.51042117235887));
#26778=CARTESIAN_POINT('',(-0.754201567294635,1.0001231722509,2.33957882764113));
#26779=CARTESIAN_POINT('',(-0.754241578414675,0.999869525658411,2.33542117235887));
#26780=CARTESIAN_POINT('',(-0.7543,1.,2.51042117235887));
#26781=CARTESIAN_POINT('Ctrl Pts',(-0.754241578414675,0.999869525658411,
2.33542117235887));
#26782=CARTESIAN_POINT('Ctrl Pts',(-0.753932917948777,1.03672405905087,
2.33352182943341));
#26783=CARTESIAN_POINT('Ctrl Pts',(-0.72236777560142,1.12483091690338,2.32900563616205));
#26784=CARTESIAN_POINT('Ctrl Pts',(-0.576126720758545,1.18012607574093,
2.3218725925448));
#26785=CARTESIAN_POINT('Ctrl Pts',(-0.436585524633584,1.079442440351,2.31402204150712));
#26786=CARTESIAN_POINT('Ctrl Pts',(-0.443598309590693,0.907512704295987,
2.30617149046944));
#26787=CARTESIAN_POINT('Ctrl Pts',(-0.59087585148424,0.818527891629664,
2.29832093943176));
#26788=CARTESIAN_POINT('Ctrl Pts',(-0.727845028742113,0.883517756536112,
2.29140416672824));
#26789=CARTESIAN_POINT('Ctrl Pts',(-0.753937170221803,0.967387714483928,
2.28710424437061));
#26790=CARTESIAN_POINT('Ctrl Pts',(-0.754138813779314,1.00010096025924,
2.28542117235887));
#26791=CARTESIAN_POINT('Ctrl Pts',(-0.754201567294635,1.0001231722509,2.33957882764113));
#26792=CARTESIAN_POINT('Ctrl Pts',(-0.754321434708458,1.01554817119723,
2.33878441566028));
#26793=CARTESIAN_POINT('Ctrl Pts',(-0.745161788983251,1.08164530518807,
2.33537315333353));
#26794=CARTESIAN_POINT('Ctrl Pts',(-0.651047892623131,1.17438223943631,
2.3293450406609));
#26795=CARTESIAN_POINT('Ctrl Pts',(-0.48270222690289,1.13876836634555,2.32149448962322));
#26796=CARTESIAN_POINT('Ctrl Pts',(-0.419550969949932,0.978702296577685,
2.31364393858554));
#26797=CARTESIAN_POINT('Ctrl Pts',(-0.518231213613428,0.837737239705173,
2.30579338754787));
#26798=CARTESIAN_POINT('Ctrl Pts',(-0.690243383915708,0.842292914261777,
2.29794283651019));
#26799=CARTESIAN_POINT('Ctrl Pts',(-0.752948977226896,0.9428032732054,2.29253798320794));
#26800=CARTESIAN_POINT('Ctrl Pts',(-0.754530925780848,0.996637557567215,
2.28974998025159));
#26801=CARTESIAN_POINT('Ctrl Pts',(-0.754515095317817,0.999943334786189,
2.28957882764113));
#26802=CARTESIAN_POINT('Origin',(-0.6,1.,2.51042117235887));
#26803=CARTESIAN_POINT('',(-0.754135271629158,0.999835375941562,2.38957882764113));
#26804=CARTESIAN_POINT('',(-0.754488127978201,1.0000741878009,2.38542117235887));
#26805=CARTESIAN_POINT('',(-0.7543,1.,2.51042117235887));
#26806=CARTESIAN_POINT('',(-0.639851384185722,0.850935057178148,2.4));
#26807=CARTESIAN_POINT('Ctrl Pts',(-0.639851384185722,0.850935057178148,
2.4));
#26808=CARTESIAN_POINT('Ctrl Pts',(-0.688870364005733,0.864039910406677,
2.39738314965411));
#26809=CARTESIAN_POINT('Ctrl Pts',(-0.744160963654378,0.915870060408085,
2.39390942553448));
#26810=CARTESIAN_POINT('Ctrl Pts',(-0.754249449960209,0.983186232192211,
2.39043570141486));
#26811=CARTESIAN_POINT('Ctrl Pts',(-0.754135271629158,0.999835375941562,
2.38957882764113));
#26812=CARTESIAN_POINT('',(-0.560048257412569,0.850698131867252,2.4));
#26813=CARTESIAN_POINT('Origin',(-0.6,1.,2.4));
#26814=CARTESIAN_POINT('Ctrl Pts',(-0.56004776881791,0.850696978396875,
2.4));
#26815=CARTESIAN_POINT('Ctrl Pts',(-0.606562014643699,0.838426852173434,
2.3975091839613));
#26816=CARTESIAN_POINT('Ctrl Pts',(-0.709748176229453,0.859960702974294,
2.39264957474759));
#26817=CARTESIAN_POINT('Ctrl Pts',(-0.754199601979702,0.954309678356425,
2.38778996553388));
#26818=CARTESIAN_POINT('Ctrl Pts',(-0.754488127978201,1.0000741878009,2.38542117235887));
#26819=CARTESIAN_POINT('Origin',(-0.6,1.,2.51042117235887));
#26820=CARTESIAN_POINT('Ctrl Pts',(-0.754488127978201,1.0000741878009,2.38542117235887));
#26821=CARTESIAN_POINT('Ctrl Pts',(-0.754518342073576,1.00486659216084,
2.38517311518799));
#26822=CARTESIAN_POINT('Ctrl Pts',(-0.75215961407118,1.06018735745674,2.38230820767121));
#26823=CARTESIAN_POINT('Ctrl Pts',(-0.685634174422424,1.16027112587027,
2.37682644980854));
#26824=CARTESIAN_POINT('Ctrl Pts',(-0.513561613772921,1.15981701793772,
2.36897589877087));
#26825=CARTESIAN_POINT('Ctrl Pts',(-0.419009660745144,1.01606137072615,
2.36112534773318));
#26826=CARTESIAN_POINT('Ctrl Pts',(-0.486773837186857,0.857888188850051,
2.35327479669551));
#26827=CARTESIAN_POINT('Ctrl Pts',(-0.656082085820325,0.827171035125292,
2.34542424565783));
#26828=CARTESIAN_POINT('Ctrl Pts',(-0.746300935356365,0.921380401738197,
2.33947303754562));
#26829=CARTESIAN_POINT('Ctrl Pts',(-0.754358179883375,0.985947131323567,
2.3361386797793));
#26830=CARTESIAN_POINT('Ctrl Pts',(-0.754241578414675,0.999869525658411,
2.33542117235887));
#26831=CARTESIAN_POINT('Ctrl Pts',(-0.754135271629158,0.999835375941562,
2.38957882764113));
#26832=CARTESIAN_POINT('Ctrl Pts',(-0.753900754954872,1.03403189804748,
2.38781885106897));
#26833=CARTESIAN_POINT('Ctrl Pts',(-0.726011265053425,1.1195363898437,2.38344202415091));
#26834=CARTESIAN_POINT('Ctrl Pts',(-0.585586769094172,1.18108616109394,
2.37644834688697));
#26835=CARTESIAN_POINT('Ctrl Pts',(-0.44099944093888,1.08793753892263,2.36859779584929));
#26836=CARTESIAN_POINT('Ctrl Pts',(-0.438948720197302,0.915842224941729,
2.36074724481161));
#26837=CARTESIAN_POINT('Ctrl Pts',(-0.581362564989717,0.819263390701727,
2.35289669377393));
#26838=CARTESIAN_POINT('Ctrl Pts',(-0.724374710267433,0.878125248400964,
2.34584055471711));
#26839=CARTESIAN_POINT('Ctrl Pts',(-0.753926582804302,0.964737112450477,
2.34140126600617));
#26840=CARTESIAN_POINT('Ctrl Pts',(-0.754201567294635,1.0001231722509,2.33957882764113));
#26841=CARTESIAN_POINT('Ctrl Pts',(-0.504188384727764,1.08252112989365,
2.4));
#26842=CARTESIAN_POINT('Ctrl Pts',(-0.4770518794945,1.0510141400767,2.39738314965411));
#26843=CARTESIAN_POINT('Ctrl Pts',(-0.456710190761643,0.959678720795721,
2.39214944896232));
#26844=CARTESIAN_POINT('Ctrl Pts',(-0.554751099480001,0.858044939225688,
2.38429889792465));
#26845=CARTESIAN_POINT('Ctrl Pts',(-0.69337483099249,0.884053256574183,
2.37644834688697));
#26846=CARTESIAN_POINT('Ctrl Pts',(-0.7482544551901,1.01388152850897,2.36859779584929));
#26847=CARTESIAN_POINT('Ctrl Pts',(-0.670177844171844,1.13134338215356,
2.36074724481161));
#26848=CARTESIAN_POINT('Ctrl Pts',(-0.52916309826044,1.13097123731837,2.35289669377393));
#26849=CARTESIAN_POINT('Ctrl Pts',(-0.451677068057184,1.01316241301569,
2.34504614273626));
#26850=CARTESIAN_POINT('Ctrl Pts',(-0.507210315698497,0.883538311601356,
2.33719559169857));
#26851=CARTESIAN_POINT('Ctrl Pts',(-0.645959687310304,0.858365375188547,
2.3293450406609));
#26852=CARTESIAN_POINT('Ctrl Pts',(-0.743491252981436,0.960210910505111,
2.32149448962322));
#26853=CARTESIAN_POINT('Ctrl Pts',(-0.712336485126218,1.097741686102,2.31364393858554));
#26854=CARTESIAN_POINT('Ctrl Pts',(-0.580435669733753,1.14761466155179,
2.30579338754787));
#26855=CARTESIAN_POINT('Ctrl Pts',(-0.466080619506913,1.06510367195323,
2.29794283651019));
#26856=CARTESIAN_POINT('Ctrl Pts',(-0.471827649045646,0.924205971861489,
2.29009228547251));
#26857=CARTESIAN_POINT('Ctrl Pts',(-0.592522692288931,0.851282254676416,
2.28224173443483));
#26858=CARTESIAN_POINT('Ctrl Pts',(-0.719923561707409,0.911732097905615,
2.27439118339715));
#26859=CARTESIAN_POINT('Ctrl Pts',(-0.739774130548921,1.051342719201,2.26654063235948));
#26860=CARTESIAN_POINT('Ctrl Pts',(-0.634271935878349,1.14490795657946,
2.2586900813218));
#26861=CARTESIAN_POINT('Ctrl Pts',(-0.498033854494106,1.10851629998956,
2.25083953028412));
#26862=CARTESIAN_POINT('Ctrl Pts',(-0.453241436429265,0.974804642442561,
2.24298897924644));
#26863=CARTESIAN_POINT('Ctrl Pts',(-0.540065587198681,0.86368878221777,
2.23513842820877));
#26864=CARTESIAN_POINT('Ctrl Pts',(-0.680640344207846,0.874820061858706,
2.22728787717108));
#26865=CARTESIAN_POINT('Ctrl Pts',(-0.748894923426505,0.998215686443256,
2.21943732613341));
#26866=CARTESIAN_POINT('Ctrl Pts',(-0.68361699553809,1.12321152562211,2.21158677509573));
#26867=CARTESIAN_POINT('Ctrl Pts',(-0.543349358171216,1.13770833955254,
2.20373622405805));
#26868=CARTESIAN_POINT('Ctrl Pts',(-0.453887363191384,1.02870504068037,
2.19588567302037));
#26869=CARTESIAN_POINT('Ctrl Pts',(-0.49546265452264,0.893958378944044,
2.1880351219827));
#26870=CARTESIAN_POINT('Ctrl Pts',(-0.630789522527785,0.854312363927335,
2.18018457094502));
#26871=CARTESIAN_POINT('Ctrl Pts',(-0.73850361471777,0.945322484520081,
2.17233401990734));
#26872=CARTESIAN_POINT('Ctrl Pts',(-0.722004372559477,1.08536870078326,
2.16448346886966));
#26873=CARTESIAN_POINT('Ctrl Pts',(-0.596088708472957,1.14885423684131,
2.15663291783199));
#26874=CARTESIAN_POINT('Ctrl Pts',(-0.473680783866961,1.07884375413848,
2.14878236679431));
#26875=CARTESIAN_POINT('Ctrl Pts',(-0.464558934858572,0.938124319016692,
2.14093181575663));
#26876=CARTESIAN_POINT('Ctrl Pts',(-0.576903853974382,0.85289646424536,
2.13308126471895));
#26877=CARTESIAN_POINT('Ctrl Pts',(-0.709961944003222,0.899594560207548,
2.12523071368127));
#26878=CARTESIAN_POINT('Ctrl Pts',(-0.744403552230901,1.03633863630844,
2.1173801626436));
#26879=CARTESIAN_POINT('Ctrl Pts',(-0.64934061440031,1.14049336981984,2.10952961160591));
#26880=CARTESIAN_POINT('Ctrl Pts',(-0.510027855146882,1.11865028889668,
2.10167906056824));
#26881=CARTESIAN_POINT('Ctrl Pts',(-0.451404225723124,0.99039884810644,
2.09382850953056));
#26882=CARTESIAN_POINT('Ctrl Pts',(-0.526044875601709,0.87075787007063,
2.08597795849289));
#26883=CARTESIAN_POINT('Ctrl Pts',(-0.667010128672949,0.867024460974769,
2.0781274074552));
#26884=CARTESIAN_POINT('Ctrl Pts',(-0.747879322472409,0.982546373509308,
2.07027685641753));
#26885=CARTESIAN_POINT('Ctrl Pts',(-0.696126397524862,1.11372170867476,
2.06242630537985));
#26886=CARTESIAN_POINT('Ctrl Pts',(-0.558165872383014,1.14290754203214,
2.05457575434217));
#26887=CARTESIAN_POINT('Ctrl Pts',(-0.457721540280641,1.04393279273302,
2.04672520330449));
#26888=CARTESIAN_POINT('Ctrl Pts',(-0.484879149484439,0.905553554682652,
2.03887465226682));
#26889=CARTESIAN_POINT('Ctrl Pts',(-0.615273516218849,0.851885006312401,
2.03102410122914));
#26890=CARTESIAN_POINT('Ctrl Pts',(-0.731982722301914,0.931032073672457,
2.02317355019146));
#26891=CARTESIAN_POINT('Ctrl Pts',(-0.730302140552184,1.07206547359851,
2.01532299915378));
#26892=CARTESIAN_POINT('Ctrl Pts',(-0.611811749466523,1.14840144523713,
2.0074724481161));
#26893=CARTESIAN_POINT('Ctrl Pts',(-0.482633225963291,1.09178094916661,
1.99962189707843));
#26894=CARTESIAN_POINT('Ctrl Pts',(-0.45890197645103,0.952575083143895,
1.99177134604075));
#26895=CARTESIAN_POINT('Ctrl Pts',(-0.527170074345267,0.888579693265875,
1.98653764534896));
#26896=CARTESIAN_POINT('Ctrl Pts',(-0.56734149364689,0.877840168374445,
1.98392079500307));
#26897=CARTESIAN_POINT('Ctrl Pts',(-0.497154370004338,1.08857942294107,
2.40535973499898));
#26898=CARTESIAN_POINT('Ctrl Pts',(-0.468025636826573,1.05475934582637,
2.40274288465309));
#26899=CARTESIAN_POINT('Ctrl Pts',(-0.446190561956348,0.956718531983702,
2.3975091839613));
#26900=CARTESIAN_POINT('Ctrl Pts',(-0.551429149092544,0.847623301048373,
2.38965863292362));
#26901=CARTESIAN_POINT('Ctrl Pts',(-0.700229949071154,0.875541020369071,
2.38180808188594));
#26902=CARTESIAN_POINT('Ctrl Pts',(-0.759138563736414,1.01490064164717,
2.37395753084827));
#26903=CARTESIAN_POINT('Ctrl Pts',(-0.675329954255372,1.14098596339246,
2.36610697981059));
#26904=CARTESIAN_POINT('Ctrl Pts',(-0.523962603431266,1.14058649752482,
2.35825642877291));
#26905=CARTESIAN_POINT('Ctrl Pts',(-0.440787932286505,1.01412873225251,
2.35040587773523));
#26906=CARTESIAN_POINT('Ctrl Pts',(-0.500398156194616,0.874988270684254,
2.34255532669756));
#26907=CARTESIAN_POINT('Ctrl Pts',(-0.649333820146978,0.84796726183413,
2.33470477565988));
#26908=CARTESIAN_POINT('Ctrl Pts',(-0.754025670789615,0.957289792428312,
2.3268542246222));
#26909=CARTESIAN_POINT('Ctrl Pts',(-0.720583674030304,1.10491739707588,
2.31900367358452));
#26910=CARTESIAN_POINT('Ctrl Pts',(-0.578999353408684,1.15845179961484,
2.31115312254684));
#26911=CARTESIAN_POINT('Ctrl Pts',(-0.456248921215803,1.06988326141916,
2.30330257150917));
#26912=CARTESIAN_POINT('Ctrl Pts',(-0.462417869227328,0.918641549339655,
2.29545202047149));
#26913=CARTESIAN_POINT('Ctrl Pts',(-0.591973745354034,0.840364133660832,
2.28760146943381));
#26914=CARTESIAN_POINT('Ctrl Pts',(-0.728727756233707,0.905251905277888,
2.27975091839613));
#26915=CARTESIAN_POINT('Ctrl Pts',(-0.750035655620193,1.05511204760418,
2.27190036735845));
#26916=CARTESIAN_POINT('Ctrl Pts',(-0.636788011835149,1.15554638175604,
2.26404981632077));
#26917=CARTESIAN_POINT('Ctrl Pts',(-0.490548004613153,1.11648302980295,
2.2561992652831));
#26918=CARTESIAN_POINT('Ctrl Pts',(-0.442467148844067,0.972954923955743,
2.24834871424542));
#26919=CARTESIAN_POINT('Ctrl Pts',(-0.535665499162523,0.85368148706755,
2.24049816320774));
#26920=CARTESIAN_POINT('Ctrl Pts',(-0.686560559276222,0.865629970182854,
2.23264761217006));
#26921=CARTESIAN_POINT('Ctrl Pts',(-0.759826051981739,0.998084690970592,
2.22479706113239));
#26922=CARTESIAN_POINT('Ctrl Pts',(-0.689755741618848,1.13225710619039,
2.21694651009471));
#26923=CARTESIAN_POINT('Ctrl Pts',(-0.539190348351968,1.14781820447026,
2.20909595905703));
#26924=CARTESIAN_POINT('Ctrl Pts',(-0.443160496353055,1.03081242273638,
2.20124540801935));
#26925=CARTESIAN_POINT('Ctrl Pts',(-0.48778803986192,0.886173327813403,
2.19339485698167));
#26926=CARTESIAN_POINT('Ctrl Pts',(-0.633049936927148,0.843616698540163,
2.185544305944));
#26927=CARTESIAN_POINT('Ctrl Pts',(-0.748671864803154,0.941308331874462,
2.17769375490632));
#26928=CARTESIAN_POINT('Ctrl Pts',(-0.730961329922812,1.09163604839579,
2.16984320386864));
#26929=CARTESIAN_POINT('Ctrl Pts',(-0.595801560801866,1.15978237838877,
2.16199265283096));
#26930=CARTESIAN_POINT('Ctrl Pts',(-0.46440705203803,1.08463207245338,2.15414210179328));
#26931=CARTESIAN_POINT('Ctrl Pts',(-0.454615522009781,0.933581712675886,
2.14629155075561));
#26932=CARTESIAN_POINT('Ctrl Pts',(-0.575208249211462,0.842096850509319,
2.13844099971793));
#26933=CARTESIAN_POINT('Ctrl Pts',(-0.718034805847138,0.892223289617803,
2.13059044868025));
#26934=CARTESIAN_POINT('Ctrl Pts',(-0.755004946535977,1.03900643918491,
2.12273989764257));
#26935=CARTESIAN_POINT('Ctrl Pts',(-0.652962958175316,1.15080769787963,
2.11488934660489));
#26936=CARTESIAN_POINT('Ctrl Pts',(-0.503422545448295,1.12736100603329,
2.10703879556722));
#26937=CARTESIAN_POINT('Ctrl Pts',(-0.440495059218284,0.989693979040313,
2.09918824452954));
#26938=CARTESIAN_POINT('Ctrl Pts',(-0.520615456293703,0.861269552373166,
2.09133769349186));
#26939=CARTESIAN_POINT('Ctrl Pts',(-0.671929680758203,0.857262054854161,
2.08348714245418));
#26940=CARTESIAN_POINT('Ctrl Pts',(-0.758735890630724,0.98126501461181,
2.07563659141651));
#26941=CARTESIAN_POINT('Ctrl Pts',(-0.703183522003752,1.12207059383778,
2.06778604037882));
#26942=CARTESIAN_POINT('Ctrl Pts',(-0.555094617726015,1.15339910667059,
2.05993548934115));
#26943=CARTESIAN_POINT('Ctrl Pts',(-0.447276159752938,1.04715812099878,
2.05208493830347));
#26944=CARTESIAN_POINT('Ctrl Pts',(-0.476427546250332,0.89861976398254,
2.0442343872658));
#26945=CARTESIAN_POINT('Ctrl Pts',(-0.616394822207238,0.841011136339552,
2.03638383622811));
#26946=CARTESIAN_POINT('Ctrl Pts',(-0.74167224073109,0.925968789770463,
2.02853328519044));
#26947=CARTESIAN_POINT('Ctrl Pts',(-0.73986827898471,1.07735616409467,2.02068273415276));
#26948=CARTESIAN_POINT('Ctrl Pts',(-0.612678909668559,1.1592963450654,2.01283218311508));
#26949=CARTESIAN_POINT('Ctrl Pts',(-0.474016738136951,1.09851905232804,
2.0049816320774));
#26950=CARTESIAN_POINT('Ctrl Pts',(-0.448543257706232,0.949093380403833,
1.99713108103973));
#26951=CARTESIAN_POINT('Ctrl Pts',(-0.5218232615616,0.880399765646143,1.99189738034794));
#26952=CARTESIAN_POINT('Ctrl Pts',(-0.564943867702685,0.86887179797568,
1.98928053000205));
#26953=CARTESIAN_POINT('Ctrl Pts',(-0.490120355280912,1.09463771598849,
2.41071946999795));
#26954=CARTESIAN_POINT('Ctrl Pts',(-0.458999394158645,1.05850455157604,
2.40810261965206));
#26955=CARTESIAN_POINT('Ctrl Pts',(-0.435670933151054,0.953758343171685,
2.40286891896027));
#26956=CARTESIAN_POINT('Ctrl Pts',(-0.548107198705087,0.837201662871056,
2.3950183679226));
#26957=CARTESIAN_POINT('Ctrl Pts',(-0.707085067149817,0.867028784163962,
2.38716781688492));
#26958=CARTESIAN_POINT('Ctrl Pts',(-0.770022672282728,1.01591975478537,
2.37931726584724));
#26959=CARTESIAN_POINT('Ctrl Pts',(-0.680482064338898,1.15062854463137,
2.37146671480957));
#26960=CARTESIAN_POINT('Ctrl Pts',(-0.518762108602093,1.15020175773127,
2.36361616377188));
#26961=CARTESIAN_POINT('Ctrl Pts',(-0.429898796515824,1.01509505148933,
2.35576561273421));
#26962=CARTESIAN_POINT('Ctrl Pts',(-0.493585996690737,0.866438229767152,
2.34791506169653));
#26963=CARTESIAN_POINT('Ctrl Pts',(-0.652707952983651,0.837569148479711,
2.34006451065885));
#26964=CARTESIAN_POINT('Ctrl Pts',(-0.764560088597795,0.954368674351516,
2.33221395962117));
#26965=CARTESIAN_POINT('Ctrl Pts',(-0.728830862934391,1.11209310804976,
2.3243634085835));
#26966=CARTESIAN_POINT('Ctrl Pts',(-0.577563037083615,1.16928893767788,
2.31651285754582));
#26967=CARTESIAN_POINT('Ctrl Pts',(-0.446417222924693,1.07466285088508,
2.30866230650814));
#26968=CARTESIAN_POINT('Ctrl Pts',(-0.453008089409011,0.913077126817822,
2.30081175547046));
#26969=CARTESIAN_POINT('Ctrl Pts',(-0.591424798419137,0.829446012645248,
2.29296120443278));
#26970=CARTESIAN_POINT('Ctrl Pts',(-0.737531950760006,0.89877171265016,
2.28511065339511));
#26971=CARTESIAN_POINT('Ctrl Pts',(-0.760297180691466,1.05888137600737,
2.27726010235743));
#26972=CARTESIAN_POINT('Ctrl Pts',(-0.639304087791949,1.16618480693263,
2.26940955131975));
#26973=CARTESIAN_POINT('Ctrl Pts',(-0.483062154732201,1.12444975961634,
2.26155900028207));
#26974=CARTESIAN_POINT('Ctrl Pts',(-0.431692861258868,0.971105205468923,
2.25370844924439));
#26975=CARTESIAN_POINT('Ctrl Pts',(-0.531265411126364,0.843674191917333,
2.24585789820672));
#26976=CARTESIAN_POINT('Ctrl Pts',(-0.692480774344598,0.856439878506999,
2.23800734716904));
#26977=CARTESIAN_POINT('Ctrl Pts',(-0.770757180536974,0.997953695497927,
2.23015679613137));
#26978=CARTESIAN_POINT('Ctrl Pts',(-0.695894487699607,1.14130268675866,
2.22230624509368));
#26979=CARTESIAN_POINT('Ctrl Pts',(-0.53503133853272,1.15792806938798,2.21445569405601));
#26980=CARTESIAN_POINT('Ctrl Pts',(-0.432433629514727,1.03291980479239,
2.20660514301833));
#26981=CARTESIAN_POINT('Ctrl Pts',(-0.480113425201198,0.878388276682764,
2.19875459198065));
#26982=CARTESIAN_POINT('Ctrl Pts',(-0.635310351326514,0.83292103315299,
2.19090404094297));
#26983=CARTESIAN_POINT('Ctrl Pts',(-0.758840114888534,0.937294179228842,
2.18305348990529));
#26984=CARTESIAN_POINT('Ctrl Pts',(-0.739918287286149,1.09790339600832,
2.17520293886762));
#26985=CARTESIAN_POINT('Ctrl Pts',(-0.595514413130776,1.17071051993624,
2.16735238782994));
#26986=CARTESIAN_POINT('Ctrl Pts',(-0.455133320209099,1.09042039076827,
2.15950183679226));
#26987=CARTESIAN_POINT('Ctrl Pts',(-0.44467210916099,0.92903910633508,2.15165128575458));
#26988=CARTESIAN_POINT('Ctrl Pts',(-0.573512644448544,0.831297236773279,
2.14380073471691));
#26989=CARTESIAN_POINT('Ctrl Pts',(-0.726107667691055,0.884852019028058,
2.13595018367922));
#26990=CARTESIAN_POINT('Ctrl Pts',(-0.765606340841053,1.04167424206138,
2.12809963264155));
#26991=CARTESIAN_POINT('Ctrl Pts',(-0.656585301950322,1.16112202593943,
2.12024908160387));
#26992=CARTESIAN_POINT('Ctrl Pts',(-0.496817235749707,1.1360717231699,2.11239853056619));
#26993=CARTESIAN_POINT('Ctrl Pts',(-0.429585892713444,0.988989109974185,
2.10454797952851));
#26994=CARTESIAN_POINT('Ctrl Pts',(-0.515186036985696,0.851781234675702,
2.09669742849084));
#26995=CARTESIAN_POINT('Ctrl Pts',(-0.67684923284346,0.847499648733552,
2.08884687745316));
#26996=CARTESIAN_POINT('Ctrl Pts',(-0.769592458789038,0.979983655714312,
2.08099632641548));
#26997=CARTESIAN_POINT('Ctrl Pts',(-0.710240646482644,1.1304194790008,2.0731457753778));
#26998=CARTESIAN_POINT('Ctrl Pts',(-0.552023363069014,1.16389067130903,
2.06529522434013));
#26999=CARTESIAN_POINT('Ctrl Pts',(-0.436830779225235,1.05038344926453,
2.05744467330245));
#27000=CARTESIAN_POINT('Ctrl Pts',(-0.467975943016225,0.891685973282426,
2.04959412226477));
#27001=CARTESIAN_POINT('Ctrl Pts',(-0.617516128195625,0.830137266366705,
2.04174357122709));
#27002=CARTESIAN_POINT('Ctrl Pts',(-0.751361759160267,0.920905505868468,
2.03389302018941));
#27003=CARTESIAN_POINT('Ctrl Pts',(-0.749434417417234,1.08264685459083,
2.02604246915173));
#27004=CARTESIAN_POINT('Ctrl Pts',(-0.613546069870597,1.17019124489367,
2.01819191811406));
#27005=CARTESIAN_POINT('Ctrl Pts',(-0.465400250310609,1.10525715548948,
2.01034136707638));
#27006=CARTESIAN_POINT('Ctrl Pts',(-0.438184538961436,0.945611677663771,
2.0024908160387));
#27007=CARTESIAN_POINT('Ctrl Pts',(-0.516476448777932,0.872219838026411,
1.99725711534692));
#27008=CARTESIAN_POINT('Ctrl Pts',(-0.56254624175848,0.859903427576914,
1.99464026500102));
#27009=CARTESIAN_POINT('Ctrl Pts',(-0.483086340557485,1.10069600903591,
2.41607920499693));
#27010=CARTESIAN_POINT('Ctrl Pts',(-0.449973151490718,1.0622497573257,2.41346235465104));
#27011=CARTESIAN_POINT('Ctrl Pts',(-0.42515130434576,0.950798154359666,
2.40822865395925));
#27012=CARTESIAN_POINT('Ctrl Pts',(-0.54478524831763,0.826780024693742,
2.40037810292158));
#27013=CARTESIAN_POINT('Ctrl Pts',(-0.71394018522848,0.858516547958849,
2.3925275518839));
#27014=CARTESIAN_POINT('Ctrl Pts',(-0.780906780829043,1.01693886792356,
2.38467700084622));
#27015=CARTESIAN_POINT('Ctrl Pts',(-0.685634174422424,1.16027112587027,
2.37682644980854));
#27016=CARTESIAN_POINT('Ctrl Pts',(-0.513561613772921,1.15981701793772,
2.36897589877087));
#27017=CARTESIAN_POINT('Ctrl Pts',(-0.419009660745144,1.01606137072615,
2.36112534773318));
#27018=CARTESIAN_POINT('Ctrl Pts',(-0.486773837186857,0.857888188850051,
2.35327479669551));
#27019=CARTESIAN_POINT('Ctrl Pts',(-0.656082085820325,0.827171035125292,
2.34542424565783));
#27020=CARTESIAN_POINT('Ctrl Pts',(-0.775094506405975,0.951447556274721,
2.33757369462015));
#27021=CARTESIAN_POINT('Ctrl Pts',(-0.737078051838477,1.11926881902364,
2.32972314358247));
#27022=CARTESIAN_POINT('Ctrl Pts',(-0.576126720758545,1.18012607574093,
2.3218725925448));
#27023=CARTESIAN_POINT('Ctrl Pts',(-0.436585524633584,1.079442440351,2.31402204150712));
#27024=CARTESIAN_POINT('Ctrl Pts',(-0.443598309590693,0.907512704295987,
2.30617149046944));
#27025=CARTESIAN_POINT('Ctrl Pts',(-0.59087585148424,0.818527891629664,
2.29832093943176));
#27026=CARTESIAN_POINT('Ctrl Pts',(-0.746336145286304,0.892291520022432,
2.29047038839408));
#27027=CARTESIAN_POINT('Ctrl Pts',(-0.77055870576274,1.06265070441055,2.28261983735641));
#27028=CARTESIAN_POINT('Ctrl Pts',(-0.641820163748749,1.17682323210921,
2.27476928631873));
#27029=CARTESIAN_POINT('Ctrl Pts',(-0.47557630485125,1.13241648942973,2.26691873528105));
#27030=CARTESIAN_POINT('Ctrl Pts',(-0.420918573673669,0.969255486982105,
2.25906818424337));
#27031=CARTESIAN_POINT('Ctrl Pts',(-0.526865323090207,0.833666896767115,
2.2512176332057));
#27032=CARTESIAN_POINT('Ctrl Pts',(-0.698400989412974,0.847249786831145,
2.24336708216802));
#27033=CARTESIAN_POINT('Ctrl Pts',(-0.781688309092209,0.997822700025263,
2.23551653113034));
#27034=CARTESIAN_POINT('Ctrl Pts',(-0.702033233780365,1.15034826732694,
2.22766598009266));
#27035=CARTESIAN_POINT('Ctrl Pts',(-0.530872328713473,1.16803793430571,
2.21981542905499));
#27036=CARTESIAN_POINT('Ctrl Pts',(-0.421706762676398,1.0350271868484,2.2119648780173));
#27037=CARTESIAN_POINT('Ctrl Pts',(-0.472438810540477,0.870603225552124,
2.20411432697963));
#27038=CARTESIAN_POINT('Ctrl Pts',(-0.637570765725878,0.822225367765818,
2.19626377594195));
#27039=CARTESIAN_POINT('Ctrl Pts',(-0.769008364973917,0.933280026583224,
2.18841322490427));
#27040=CARTESIAN_POINT('Ctrl Pts',(-0.748875244649484,1.10417074362085,
2.18056267386659));
#27041=CARTESIAN_POINT('Ctrl Pts',(-0.595227265459685,1.1816386614837,2.17271212282892));
#27042=CARTESIAN_POINT('Ctrl Pts',(-0.445859588380167,1.09620870908317,
2.16486157179124));
#27043=CARTESIAN_POINT('Ctrl Pts',(-0.434728696312199,0.924496499994273,
2.15701102075356));
#27044=CARTESIAN_POINT('Ctrl Pts',(-0.571817039685625,0.820497623037239,
2.14916046971588));
#27045=CARTESIAN_POINT('Ctrl Pts',(-0.734180529534971,0.877480748438312,
2.14130991867821));
#27046=CARTESIAN_POINT('Ctrl Pts',(-0.776207735146129,1.04434204493786,
2.13345936764052));
#27047=CARTESIAN_POINT('Ctrl Pts',(-0.660207645725328,1.17143635399922,
2.12560881660285));
#27048=CARTESIAN_POINT('Ctrl Pts',(-0.490211926051119,1.14478244030651,
2.11775826556517));
#27049=CARTESIAN_POINT('Ctrl Pts',(-0.418676726208604,0.988284240908056,
2.10990771452749));
#27050=CARTESIAN_POINT('Ctrl Pts',(-0.509756617677689,0.842292916978238,
2.10205716348981));
#27051=CARTESIAN_POINT('Ctrl Pts',(-0.681768784928714,0.837737242612945,
2.09420661245213));
#27052=CARTESIAN_POINT('Ctrl Pts',(-0.780449026947353,0.978702296816814,
2.08635606141446));
#27053=CARTESIAN_POINT('Ctrl Pts',(-0.717297770961535,1.13876836416382,
2.07850551037678));
#27054=CARTESIAN_POINT('Ctrl Pts',(-0.548952108412014,1.17438223594748,
2.0706549593391));
#27055=CARTESIAN_POINT('Ctrl Pts',(-0.426385398697532,1.05360877753029,
2.06280440830142));
#27056=CARTESIAN_POINT('Ctrl Pts',(-0.459524339782119,0.884752182582313,
2.05495385726375));
#27057=CARTESIAN_POINT('Ctrl Pts',(-0.618637434184013,0.819263396393857,
2.04710330622607));
#27058=CARTESIAN_POINT('Ctrl Pts',(-0.761051277589445,0.915842221966472,
2.03925275518839));
#27059=CARTESIAN_POINT('Ctrl Pts',(-0.759000555849758,1.08793754508699,
2.03140220415071));
#27060=CARTESIAN_POINT('Ctrl Pts',(-0.614413230072635,1.18108614472194,
2.02355165311304));
#27061=CARTESIAN_POINT('Ctrl Pts',(-0.456783762484268,1.11199525865091,
2.01570110207535));
#27062=CARTESIAN_POINT('Ctrl Pts',(-0.427825820216639,0.942129974923708,
2.00785055103768));
#27063=CARTESIAN_POINT('Ctrl Pts',(-0.511129635994264,0.864039910406679,
2.00261685034589));
#27064=CARTESIAN_POINT('Ctrl Pts',(-0.560148615814275,0.850935057178149,
2.));
#27065=CARTESIAN_POINT('Ctrl Pts',(-0.560148615814275,0.850935057178149,
2.));
#27066=CARTESIAN_POINT('Ctrl Pts',(-0.550119441743087,0.85459967610481,
2.));
#27067=CARTESIAN_POINT('Ctrl Pts',(-0.540564999899567,0.859362631836586,
2.));
#27068=CARTESIAN_POINT('Ctrl Pts',(-0.531596825272739,0.86507409197529,
2.));
#27069=CARTESIAN_POINT('Ctrl Pts',(-0.527131635014649,0.867917787290334,
2.));
#27070=CARTESIAN_POINT('Ctrl Pts',(-0.522812202969371,0.870997335784893,
2.));
#27071=CARTESIAN_POINT('Ctrl Pts',(-0.518655551555349,0.874297548143145,
2.));
#27072=CARTESIAN_POINT('Ctrl Pts',(-0.515850210886717,0.876524874666724,
2.));
#27073=CARTESIAN_POINT('Ctrl Pts',(-0.51311906464033,0.878852752659134,
2.));
#27074=CARTESIAN_POINT('Ctrl Pts',(-0.510468070497139,0.881276854651557,
2.));
#27075=CARTESIAN_POINT('Ctrl Pts',(-0.508096882944962,0.883445098019579,
2.));
#27076=CARTESIAN_POINT('Ctrl Pts',(-0.505796523707934,0.885684247113283,
2.));
#27077=CARTESIAN_POINT('Ctrl Pts',(-0.503571407093493,0.887989067169883,
2.));
#27078=CARTESIAN_POINT('Ctrl Pts',(-0.496344337828248,0.895475009293033,
2.));
#27079=CARTESIAN_POINT('Ctrl Pts',(-0.489902887206981,0.90365635994166,
2.));
#27080=CARTESIAN_POINT('Ctrl Pts',(-0.4843803033401,0.912413093858066,2.));
#27081=CARTESIAN_POINT('Ctrl Pts',(-0.482085852075076,0.91605122769112,
2.));
#27082=CARTESIAN_POINT('Ctrl Pts',(-0.479950567463666,0.919788922535331,
2.));
#27083=CARTESIAN_POINT('Ctrl Pts',(-0.477986666560954,0.923618208076587,
2.));
#27084=CARTESIAN_POINT('Ctrl Pts',(-0.47650289740366,0.926511315245457,
2.));
#27085=CARTESIAN_POINT('Ctrl Pts',(-0.475117210175375,0.929457020402162,
2.));
#27086=CARTESIAN_POINT('Ctrl Pts',(-0.473840374763333,0.932438174193855,
2.));
#27087=CARTESIAN_POINT('Ctrl Pts',(-0.470678071962382,0.939821514988315,
2.));
#27088=CARTESIAN_POINT('Ctrl Pts',(-0.468171074744705,0.947441922900028,
2.));
#27089=CARTESIAN_POINT('Ctrl Pts',(-0.466390213028648,0.95524361805541,
2.));
#27090=CARTESIAN_POINT('Ctrl Pts',(-0.464752059680358,0.962420128688376,
2.));
#27091=CARTESIAN_POINT('Ctrl Pts',(-0.463728780577517,0.969750541677906,
2.));
#27092=CARTESIAN_POINT('Ctrl Pts',(-0.463308983993722,0.977159407672611,
2.));
#27093=CARTESIAN_POINT('Ctrl Pts',(-0.46313283978449,0.9802681248283,2.));
#27094=CARTESIAN_POINT('Ctrl Pts',(-0.463063521137214,0.983387155046876,
2.));
#27095=CARTESIAN_POINT('Ctrl Pts',(-0.463099420187341,0.986501027428933,
2.));
#27096=CARTESIAN_POINT('Ctrl Pts',(-0.463196744049792,0.994942868824082,
2.));
#27097=CARTESIAN_POINT('Ctrl Pts',(-0.464064111260558,1.00336874731576,
2.));
#27098=CARTESIAN_POINT('Ctrl Pts',(-0.465675457037548,1.01166504030789,
2.));
#27099=CARTESIAN_POINT('Ctrl Pts',(-0.466871286975471,1.01782197799031,
2.));
#27100=CARTESIAN_POINT('Ctrl Pts',(-0.468477483228933,1.02390757245997,
2.));
#27101=CARTESIAN_POINT('Ctrl Pts',(-0.47049180892072,1.02987016754483,2.));
#27102=CARTESIAN_POINT('Ctrl Pts',(-0.471677004317114,1.03337845832122,
2.));
#27103=CARTESIAN_POINT('Ctrl Pts',(-0.473001297362186,1.03683670978256,
2.));
#27104=CARTESIAN_POINT('Ctrl Pts',(-0.474460925722079,1.04022912201569,
2.));
#27105=CARTESIAN_POINT('Ctrl Pts',(-0.476751357662528,1.04555245605566,
2.));
#27106=CARTESIAN_POINT('Ctrl Pts',(-0.479376312983413,1.05071850549913,
2.));
#27107=CARTESIAN_POINT('Ctrl Pts',(-0.482333055615295,1.05568494193306,
2.));
#27108=CARTESIAN_POINT('Ctrl Pts',(-0.484374509820886,1.05911396968661,
2.));
#27109=CARTESIAN_POINT('Ctrl Pts',(-0.486574680171624,1.06244757845398,
2.));
#27110=CARTESIAN_POINT('Ctrl Pts',(-0.488924280031899,1.0656592034053,2.));
#27111=CARTESIAN_POINT('Ctrl Pts',(-0.492216707647991,1.07015956232216,
2.));
#27112=CARTESIAN_POINT('Ctrl Pts',(-0.495805970213506,1.07442716727356,
2.));
#27113=CARTESIAN_POINT('Ctrl Pts',(-0.499690940637682,1.07842077494232,
2.));
#27114=CARTESIAN_POINT('Ctrl Pts',(-0.501092717011139,1.07986174984398,
2.));
#27115=CARTESIAN_POINT('Ctrl Pts',(-0.502533033199793,1.08126699098065,
2.));
#27116=CARTESIAN_POINT('Ctrl Pts',(-0.504010174669742,1.08263575197434,
2.));
#27117=CARTESIAN_POINT('Ctrl Pts',(-0.504188384727764,1.08252112989365,
2.4));
#27118=CARTESIAN_POINT('Ctrl Pts',(-0.497506954663502,1.07628156217526,
2.4));
#27119=CARTESIAN_POINT('Ctrl Pts',(-0.491604269963233,1.06931033894935,
2.4));
#27120=CARTESIAN_POINT('Ctrl Pts',(-0.48648731081533,1.06178682142811,2.4));
#27121=CARTESIAN_POINT('Ctrl Pts',(-0.482497621478512,1.05592074027282,
2.4));
#27122=CARTESIAN_POINT('Ctrl Pts',(-0.478985885254584,1.04971755224006,
2.4));
#27123=CARTESIAN_POINT('Ctrl Pts',(-0.475968008505373,1.04324617240972,
2.4));
#27124=CARTESIAN_POINT('Ctrl Pts',(-0.474670784833122,1.04046447262352,
2.4));
#27125=CARTESIAN_POINT('Ctrl Pts',(-0.473467326409776,1.03763771123602,
2.4));
#27126=CARTESIAN_POINT('Ctrl Pts',(-0.472361166010358,1.03477908326479,
2.4));
#27127=CARTESIAN_POINT('Ctrl Pts',(-0.46880698586937,1.02559408733548,2.4));
#27128=CARTESIAN_POINT('Ctrl Pts',(-0.466243719906724,1.01606060675579,
2.4));
#27129=CARTESIAN_POINT('Ctrl Pts',(-0.464705314070165,1.00636042835626,
2.4));
#27130=CARTESIAN_POINT('Ctrl Pts',(-0.463992227392452,1.00186417137142,
2.4));
#27131=CARTESIAN_POINT('Ctrl Pts',(-0.463499928942431,0.997331640290426,
2.4));
#27132=CARTESIAN_POINT('Ctrl Pts',(-0.463235268916811,0.992779403524773,
2.4));
#27133=CARTESIAN_POINT('Ctrl Pts',(-0.463040851274643,0.989435358134849,
2.4));
#27134=CARTESIAN_POINT('Ctrl Pts',(-0.462969940004504,0.986088143884579,
2.4));
#27135=CARTESIAN_POINT('Ctrl Pts',(-0.463023793901296,0.982751466845985,
2.4));
#27136=CARTESIAN_POINT('Ctrl Pts',(-0.463137062422501,0.975733581485534,
2.4));
#27137=CARTESIAN_POINT('Ctrl Pts',(-0.463800894161501,0.968753185610107,
2.4));
#27138=CARTESIAN_POINT('Ctrl Pts',(-0.465031332332612,0.96187163776825,
2.4));
#27139=CARTESIAN_POINT('Ctrl Pts',(-0.466389645164331,0.954274917384296,
2.4));
#27140=CARTESIAN_POINT('Ctrl Pts',(-0.468438000905081,0.946798204321114,
2.4));
#27141=CARTESIAN_POINT('Ctrl Pts',(-0.471116528460654,0.93949859713407,
2.4));
#27142=CARTESIAN_POINT('Ctrl Pts',(-0.472251134057494,0.936406534425243,
2.4));
#27143=CARTESIAN_POINT('Ctrl Pts',(-0.473496260389133,0.933354194164882,
2.4));
#27144=CARTESIAN_POINT('Ctrl Pts',(-0.474844488633202,0.930349739998837,
2.4));
#27145=CARTESIAN_POINT('Ctrl Pts',(-0.478666411965482,0.9218327893056,2.4));
#27146=CARTESIAN_POINT('Ctrl Pts',(-0.4833179823867,0.913689872025069,2.4));
#27147=CARTESIAN_POINT('Ctrl Pts',(-0.488689869589499,0.906016299690457,
2.4));
#27148=CARTESIAN_POINT('Ctrl Pts',(-0.491565626713204,0.901908370861642,
2.4));
#27149=CARTESIAN_POINT('Ctrl Pts',(-0.494648453197326,0.897935009702848,
2.4));
#27150=CARTESIAN_POINT('Ctrl Pts',(-0.497925430586844,0.894112166139119,
2.4));
#27151=CARTESIAN_POINT('Ctrl Pts',(-0.500336511660046,0.89129945653917,
2.4));
#27152=CARTESIAN_POINT('Ctrl Pts',(-0.502853434868661,0.888568042774596,
2.4));
#27153=CARTESIAN_POINT('Ctrl Pts',(-0.505459753140441,0.885935602377086,
2.4));
#27154=CARTESIAN_POINT('Ctrl Pts',(-0.510032980818731,0.881316538996496,
2.4));
#27155=CARTESIAN_POINT('Ctrl Pts',(-0.514888373574847,0.876993017632294,
2.4));
#27156=CARTESIAN_POINT('Ctrl Pts',(-0.519995790255463,0.872997627556259,
2.4));
#27157=CARTESIAN_POINT('Ctrl Pts',(-0.524771384850184,0.869261812672909,
2.4));
#27158=CARTESIAN_POINT('Ctrl Pts',(-0.529772960099733,0.865810225418053,
2.4));
#27159=CARTESIAN_POINT('Ctrl Pts',(-0.534950219195867,0.86268896384257,
2.4));
#27160=CARTESIAN_POINT('Ctrl Pts',(-0.540826101062414,0.859146517163432,
2.4));
#27161=CARTESIAN_POINT('Ctrl Pts',(-0.546932707573367,0.85602468566073,
2.4));
#27162=CARTESIAN_POINT('Ctrl Pts',(-0.553238064171717,0.853364150883981,
2.4));
#27163=CARTESIAN_POINT('Ctrl Pts',(-0.555483414843566,0.852416728885673,
2.4));
#27164=CARTESIAN_POINT('Ctrl Pts',(-0.557754020887936,0.851527863380312,
2.4));
#27165=CARTESIAN_POINT('Ctrl Pts',(-0.560047768817924,0.850696978396871,
2.4));
#27166=CARTESIAN_POINT('Ctrl Pts',(-0.72640212307541,0.999893075304641,
2.31934196736194));
#27167=CARTESIAN_POINT('Ctrl Pts',(-0.726497678848041,0.988483569383442,
2.32005947478237));
#27168=CARTESIAN_POINT('Ctrl Pts',(-0.725076811113891,0.977097445695636,
2.32077698220279));
#27169=CARTESIAN_POINT('Ctrl Pts',(-0.722043530727044,0.966158450551832,
2.32149448962322));
#27170=CARTESIAN_POINT('Ctrl Pts',(-0.710980731091059,0.926262398732923,
2.32411133996911));
#27171=CARTESIAN_POINT('Ctrl Pts',(-0.678470209200682,0.892313886960735,
2.32672819031501));
#27172=CARTESIAN_POINT('Ctrl Pts',(-0.639090052986859,0.879535120476776,
2.3293450406609));
#27173=CARTESIAN_POINT('Ctrl Pts',(-0.599709896773035,0.866756353992817,
2.33196189100679));
#27174=CARTESIAN_POINT('Ctrl Pts',(-0.553460106235766,0.875147332797086,
2.33457874135268));
#27175=CARTESIAN_POINT('Ctrl Pts',(-0.52107966969358,0.900946839101611,
2.33719559169858));
#27176=CARTESIAN_POINT('Ctrl Pts',(-0.488699233151393,0.926746345406136,
2.33981244204447));
#27177=CARTESIAN_POINT('Ctrl Pts',(-0.470188150604288,0.969954379210915,
2.34242929239036));
#27178=CARTESIAN_POINT('Ctrl Pts',(-0.473846947697945,1.01119320016375,
2.34504614273626));
#27179=CARTESIAN_POINT('Ctrl Pts',(-0.477505744791602,1.05243202111659,
2.34766299308215));
#27180=CARTESIAN_POINT('Ctrl Pts',(-0.503334421526021,1.09170162921748,
2.35027984342804));
#27181=CARTESIAN_POINT('Ctrl Pts',(-0.539751217545131,1.11139845740712,
2.35289669377393));
#27182=CARTESIAN_POINT('Ctrl Pts',(-0.576168013564241,1.13109528559677,
2.35551354411982));
#27183=CARTESIAN_POINT('Ctrl Pts',(-0.623172928868043,1.13121933387517,
2.35813039446572));
#27184=CARTESIAN_POINT('Ctrl Pts',(-0.659688155022986,1.11170438240693,
2.36074724481161));
#27185=CARTESIAN_POINT('Ctrl Pts',(-0.696203381177929,1.0921894309387,2.3633640951575));
#27186=CARTESIAN_POINT('Ctrl Pts',(-0.722228918184014,1.05303547972384,
2.3659809455034));
#27187=CARTESIAN_POINT('Ctrl Pts',(-0.726095082654122,1.01182045879394,
2.36859779584929));
#27188=CARTESIAN_POINT('Ctrl Pts',(-0.726461565140266,1.00791359361693,
2.36884585302017));
#27189=CARTESIAN_POINT('Ctrl Pts',(-0.726628932956602,1.00398820854659,
2.36909391019106));
#27190=CARTESIAN_POINT('Ctrl Pts',(-0.726604172280256,1.00006079745576,
2.36934196736194));
#27191=CARTESIAN_POINT('Ctrl Pts',(-0.639851384185722,0.850935057178148,
2.4));
#27192=CARTESIAN_POINT('Ctrl Pts',(-0.688870364005733,0.864039910406677,
2.39738314965411));
#27193=CARTESIAN_POINT('Ctrl Pts',(-0.772174172732383,0.942130018479807,
2.39214944896232));
#27194=CARTESIAN_POINT('Ctrl Pts',(-0.743216243669936,1.11199523763249,
2.38429889792464));
#27195=CARTESIAN_POINT('Ctrl Pts',(-0.585586769094172,1.18108616109394,
2.37644834688697));
#27196=CARTESIAN_POINT('Ctrl Pts',(-0.44099944093888,1.08793753892263,2.36859779584929));
#27197=CARTESIAN_POINT('Ctrl Pts',(-0.438948720197302,0.915842224941729,
2.36074724481161));
#27198=CARTESIAN_POINT('Ctrl Pts',(-0.581362564989717,0.819263390701727,
2.35289669377393));
#27199=CARTESIAN_POINT('Ctrl Pts',(-0.740475663026546,0.88475218199663,
2.34504614273626));
#27200=CARTESIAN_POINT('Ctrl Pts',(-0.773614604105453,1.05360877766967,
2.33719559169858));
#27201=CARTESIAN_POINT('Ctrl Pts',(-0.651047892623131,1.17438223943631,
2.3293450406609));
#27202=CARTESIAN_POINT('Ctrl Pts',(-0.48270222690289,1.13876836634555,2.32149448962322));
#27203=CARTESIAN_POINT('Ctrl Pts',(-0.419550969949932,0.978702296577685,
2.31364393858554));
#27204=CARTESIAN_POINT('Ctrl Pts',(-0.518231213613428,0.837737239705173,
2.30579338754787));
#27205=CARTESIAN_POINT('Ctrl Pts',(-0.690243383915708,0.842292914261777,
2.29794283651019));
#27206=CARTESIAN_POINT('Ctrl Pts',(-0.781323276950512,0.988284240682119,
2.29009228547251));
#27207=CARTESIAN_POINT('Ctrl Pts',(-0.709788075872465,1.14478244284782,
2.28224173443483));
#27208=CARTESIAN_POINT('Ctrl Pts',(-0.539792353219763,1.17143635698873,
2.27439118339715));
#27209=CARTESIAN_POINT('Ctrl Pts',(-0.423792261776434,1.04434204571596,
2.26654063235948));
#27210=CARTESIAN_POINT('Ctrl Pts',(-0.465819468119529,0.877480746295693,
2.2586900813218));
#27211=CARTESIAN_POINT('Ctrl Pts',(-0.6281829608073,0.820497619901593,2.25083953028412));
#27212=CARTESIAN_POINT('Ctrl Pts',(-0.765271306575456,0.924496498674441,
2.24298897924644));
#27213=CARTESIAN_POINT('Ctrl Pts',(-0.754140414313383,1.09620871076456,
2.23513842820876));
#27214=CARTESIAN_POINT('Ctrl Pts',(-0.604772734623643,1.18163866465747,
2.22728787717109));
#27215=CARTESIAN_POINT('Ctrl Pts',(-0.451124752749149,1.10417074544119,
2.21943732613341));
#27216=CARTESIAN_POINT('Ctrl Pts',(-0.43099163207285,0.933280025417337,
2.21158677509573));
#27217=CARTESIAN_POINT('Ctrl Pts',(-0.562429233617627,0.822225364659454,
2.20373622405805));
#27218=CARTESIAN_POINT('Ctrl Pts',(-0.727561191688486,0.870603223291056,
2.19588567302038));
#27219=CARTESIAN_POINT('Ctrl Pts',(-0.778293240439059,1.03502718746047,
2.1880351219827));
#27220=CARTESIAN_POINT('Ctrl Pts',(-0.669127672494447,1.16803793724193,
2.18018457094502));
#27221=CARTESIAN_POINT('Ctrl Pts',(-0.497966764436741,1.15034826995414,
2.17233401990734));
#27222=CARTESIAN_POINT('Ctrl Pts',(-0.418311687733005,0.997822699987136,
2.16448346886966));
#27223=CARTESIAN_POINT('Ctrl Pts',(-0.501599008867606,0.847249784162188,
2.15663291783199));
#27224=CARTESIAN_POINT('Ctrl Pts',(-0.673134678187691,0.833666893860354,
2.1487823667943));
#27225=CARTESIAN_POINT('Ctrl Pts',(-0.779081429455625,0.969255486445431,
2.14093181575663));
#27226=CARTESIAN_POINT('Ctrl Pts',(-0.724423697322763,1.1324164917425,2.13308126471895));
#27227=CARTESIAN_POINT('Ctrl Pts',(-0.558179835520779,1.17682323520091,
2.12523071368127));
#27228=CARTESIAN_POINT('Ctrl Pts',(-0.429441291256411,1.0626507055017,2.1173801626436));
#27229=CARTESIAN_POINT('Ctrl Pts',(-0.453663852157743,0.892291518147041,
2.10952961160592));
#27230=CARTESIAN_POINT('Ctrl Pts',(-0.609124148673025,0.818527888446316,
2.10167906056824));
#27231=CARTESIAN_POINT('Ctrl Pts',(-0.756401693146515,0.907512702702641,
2.09382850953056));
#27232=CARTESIAN_POINT('Ctrl Pts',(-0.763414478213392,1.07944244169741,
2.08597795849288));
#27233=CARTESIAN_POINT('Ctrl Pts',(-0.623873279675432,1.18012607896462,
2.0781274074552));
#27234=CARTESIAN_POINT('Ctrl Pts',(-0.462921945732953,1.11926882096942,
2.07027685641753));
#27235=CARTESIAN_POINT('Ctrl Pts',(-0.424905490600427,0.951447555675582,
2.06242630537985));
#27236=CARTESIAN_POINT('Ctrl Pts',(-0.54391791306908,0.827171031659744,
2.05457575434217));
#27237=CARTESIAN_POINT('Ctrl Pts',(-0.713226165050295,0.857888187155562,
2.04672520330449));
#27238=CARTESIAN_POINT('Ctrl Pts',(-0.780990341905239,1.01606136962747,
2.03887465226682));
#27239=CARTESIAN_POINT('Ctrl Pts',(-0.686438388751686,1.15981702310584,
2.03102410122914));
#27240=CARTESIAN_POINT('Ctrl Pts',(-0.514365822072695,1.16027112465931,
2.02317355019146));
#27241=CARTESIAN_POINT('Ctrl Pts',(-0.41909321999119,1.01693887482571,2.01532299915378));
#27242=CARTESIAN_POINT('Ctrl Pts',(-0.486059804858393,0.858516534902566,
2.0074724481161));
#27243=CARTESIAN_POINT('Ctrl Pts',(-0.655214768609463,0.826780038590561,
1.99962189707843));
#27244=CARTESIAN_POINT('Ctrl Pts',(-0.774848665287453,0.950798122348591,
1.99177134604075));
#27245=CARTESIAN_POINT('Ctrl Pts',(-0.750026848509283,1.0622497573257,1.98653764534896));
#27246=CARTESIAN_POINT('Ctrl Pts',(-0.716913659442517,1.10069600903591,
1.98392079500307));
#27247=CARTESIAN_POINT('Ctrl Pts',(-0.637453758241517,0.859903427576914,
2.40535973499898));
#27248=CARTESIAN_POINT('Ctrl Pts',(-0.683523551222066,0.872219838026409,
2.40274288465309));
#27249=CARTESIAN_POINT('Ctrl Pts',(-0.761815454411802,0.945611718599352,
2.3975091839613));
#27250=CARTESIAN_POINT('Ctrl Pts',(-0.734599755473333,1.10525713573561,
2.38965863292362));
#27251=CARTESIAN_POINT('Ctrl Pts',(-0.586453929346337,1.17019126028066,
2.38180808188594));
#27252=CARTESIAN_POINT('Ctrl Pts',(-0.450565579564614,1.08264684879734,
2.37395753084827));
#27253=CARTESIAN_POINT('Ctrl Pts',(-0.448638238759637,0.920905508664721,
2.36610697981058));
#27254=CARTESIAN_POINT('Ctrl Pts',(-0.582483871027817,0.830137261017037,
2.35825642877291));
#27255=CARTESIAN_POINT('Ctrl Pts',(-0.732024059623459,0.891685972731981,
2.35040587773523));
#27256=CARTESIAN_POINT('Ctrl Pts',(-0.76316922340911,1.05038344939552,2.34255532669756));
#27257=CARTESIAN_POINT('Ctrl Pts',(-0.647976637903853,1.16389067458796,
2.33470477565988));
#27258=CARTESIAN_POINT('Ctrl Pts',(-0.489759351510266,1.13041948105126,
2.3268542246222));
#27259=CARTESIAN_POINT('Ctrl Pts',(-0.430407538294919,0.979983655489569,
2.31900367358452));
#27260=CARTESIAN_POINT('Ctrl Pts',(-0.523150765786394,0.847499646000726,
2.31115312254684));
#27261=CARTESIAN_POINT('Ctrl Pts',(-0.684813964511835,0.851781232122674,
2.30330257150917));
#27262=CARTESIAN_POINT('Ctrl Pts',(-0.770414110255606,0.98898910976184,
2.29545202047149));
#27263=CARTESIAN_POINT('Ctrl Pts',(-0.703182766058146,1.13607172555832,
2.28760146943381));
#27264=CARTESIAN_POINT('Ctrl Pts',(-0.543414697058237,1.16112202874907,
2.27975091839613));
#27265=CARTESIAN_POINT('Ctrl Pts',(-0.434393656266662,1.04167424279268,
2.27190036735845));
#27266=CARTESIAN_POINT('Ctrl Pts',(-0.47389233010456,0.884852017014347,
2.26404981632077));
#27267=CARTESIAN_POINT('Ctrl Pts',(-0.626487356014725,0.831297233826287,
2.2561992652831));
#27268=CARTESIAN_POINT('Ctrl Pts',(-0.755327893552931,0.929039105094654,
2.24834871424542));
#27269=CARTESIAN_POINT('Ctrl Pts',(-0.744866682322397,1.0904203923485,2.24049816320774));
#27270=CARTESIAN_POINT('Ctrl Pts',(-0.604485586947538,1.17071052291906,
2.23264761217006));
#27271=CARTESIAN_POINT('Ctrl Pts',(-0.460081710268994,1.09790339771914,
2.22479706113239));
#27272=CARTESIAN_POINT('Ctrl Pts',(-0.441159882335912,0.937294178133102,
2.21694651009471));
#27273=CARTESIAN_POINT('Ctrl Pts',(-0.564689648056489,0.832921030233517,
2.20909595905703));
#27274=CARTESIAN_POINT('Ctrl Pts',(-0.719886576893662,0.878388274557731,
2.20124540801935));
#27275=CARTESIAN_POINT('Ctrl Pts',(-0.767566373413291,1.03291980536764,
2.19339485698167));
#27276=CARTESIAN_POINT('Ctrl Pts',(-0.664968662602526,1.15792807214755,
2.185544305944));
#27277=CARTESIAN_POINT('Ctrl Pts',(-0.504105510624766,1.1413026892278,2.17769375490632));
#27278=CARTESIAN_POINT('Ctrl Pts',(-0.429242816479248,0.997953695462094,
2.16984320386864));
#27279=CARTESIAN_POINT('Ctrl Pts',(-0.50751922403943,0.856439875998617,
2.16199265283096));
#27280=CARTESIAN_POINT('Ctrl Pts',(-0.668734590074648,0.843674189185456,
2.15414210179328));
#27281=CARTESIAN_POINT('Ctrl Pts',(-0.768307141682156,0.971105204964537,
2.14629155075561));
#27282=CARTESIAN_POINT('Ctrl Pts',(-0.716937847311012,1.12444976178997,
2.13844099971793));
#27283=CARTESIAN_POINT('Ctrl Pts',(-0.560695911521528,1.16618480983832,
2.13059044868025));
#27284=CARTESIAN_POINT('Ctrl Pts',(-0.439702816507024,1.05888137703287,
2.12273989764257));
#27285=CARTESIAN_POINT('Ctrl Pts',(-0.462468046837819,0.8987717108876,2.11488934660489));
#27286=CARTESIAN_POINT('Ctrl Pts',(-0.608575201728667,0.829446009653423,
2.10703879556722));
#27287=CARTESIAN_POINT('Ctrl Pts',(-0.746991913163515,0.913077125320336,
2.09918824452953));
#27288=CARTESIAN_POINT('Ctrl Pts',(-0.753582779750997,1.07466285215048,
2.09133769349186));
#27289=CARTESIAN_POINT('Ctrl Pts',(-0.622436963324253,1.16928894070762,
2.08348714245418));
#27290=CARTESIAN_POINT('Ctrl Pts',(-0.471169134783152,1.11209310987848,
2.07563659141651));
#27291=CARTESIAN_POINT('Ctrl Pts',(-0.435439908588715,0.954368673788424,
2.06778604037882));
#27292=CARTESIAN_POINT('Ctrl Pts',(-0.547292045972571,0.837569145222665,
2.05993548934115));
#27293=CARTESIAN_POINT('Ctrl Pts',(-0.706414005411818,0.866438228174611,
2.05208493830347));
#27294=CARTESIAN_POINT('Ctrl Pts',(-0.770101205975101,1.01509505045675,
2.04423438726579));
#27295=CARTESIAN_POINT('Ctrl Pts',(-0.681237893770622,1.15020176258845,
2.03638383622811));
#27296=CARTESIAN_POINT('Ctrl Pts',(-0.519517932367091,1.15062854349327,
2.02853328519044));
#27297=CARTESIAN_POINT('Ctrl Pts',(-0.429977328488155,1.01591976127225,
2.02068273415276));
#27298=CARTESIAN_POINT('Ctrl Pts',(-0.492914923533471,0.867028771893199,
2.01283218311508));
#27299=CARTESIAN_POINT('Ctrl Pts',(-0.651892817203601,0.837201675931786,
2.0049816320774));
#27300=CARTESIAN_POINT('Ctrl Pts',(-0.764329038309151,0.95375831308653,
1.99713108103972));
#27301=CARTESIAN_POINT('Ctrl Pts',(-0.741000605841356,1.05850455157603,
1.99189738034794));
#27302=CARTESIAN_POINT('Ctrl Pts',(-0.709879644719091,1.09463771598849,
1.98928053000205));
#27303=CARTESIAN_POINT('Ctrl Pts',(-0.635056132297313,0.868871797975679,
2.41071946999795));
#27304=CARTESIAN_POINT('Ctrl Pts',(-0.678176738438398,0.880399765646142,
2.40810261965206));
#27305=CARTESIAN_POINT('Ctrl Pts',(-0.751456736091222,0.949093418718895,
2.40286891896028));
#27306=CARTESIAN_POINT('Ctrl Pts',(-0.725983267276729,1.09851903383873,
2.3950183679226));
#27307=CARTESIAN_POINT('Ctrl Pts',(-0.587321089598503,1.15929635946738,
2.38716781688492));
#27308=CARTESIAN_POINT('Ctrl Pts',(-0.460131718190347,1.07735615867206,
2.37931726584724));
#27309=CARTESIAN_POINT('Ctrl Pts',(-0.458327757321973,0.925968792387711,
2.37146671480957));
#27310=CARTESIAN_POINT('Ctrl Pts',(-0.583605177065917,0.841011131332347,
2.36361616377189));
#27311=CARTESIAN_POINT('Ctrl Pts',(-0.72357245622037,0.898619763467331,
2.35576561273421));
#27312=CARTESIAN_POINT('Ctrl Pts',(-0.752723842712768,1.04715812112138,
2.34791506169653));
#27313=CARTESIAN_POINT('Ctrl Pts',(-0.644905383184573,1.15339910973961,
2.34006451065885));
#27314=CARTESIAN_POINT('Ctrl Pts',(-0.496816476117644,1.12207059575698,
2.33221395962118));
#27315=CARTESIAN_POINT('Ctrl Pts',(-0.441264106639905,0.981265014401455,
2.3243634085835));
#27316=CARTESIAN_POINT('Ctrl Pts',(-0.528070317959361,0.857262052296277,
2.31651285754582));
#27317=CARTESIAN_POINT('Ctrl Pts',(-0.679384545107962,0.861269549983572,
2.30866230650814));
#27318=CARTESIAN_POINT('Ctrl Pts',(-0.759504943560701,0.989693978841561,
2.30081175547046));
#27319=CARTESIAN_POINT('Ctrl Pts',(-0.696577456243827,1.12736100826881,
2.29296120443279));
#27320=CARTESIAN_POINT('Ctrl Pts',(-0.547037040896711,1.15080770050942,
2.28511065339511));
#27321=CARTESIAN_POINT('Ctrl Pts',(-0.444995050756889,1.03900643986939,
2.27726010235743));
#27322=CARTESIAN_POINT('Ctrl Pts',(-0.481965192089592,0.892223287733,2.26940955131975));
#27323=CARTESIAN_POINT('Ctrl Pts',(-0.624791751222149,0.842096847750981,
2.26155900028208));
#27324=CARTESIAN_POINT('Ctrl Pts',(-0.745384480530408,0.933581711514867,
2.2537084492444));
#27325=CARTESIAN_POINT('Ctrl Pts',(-0.735592950331409,1.08463207393244,
2.24585789820672));
#27326=CARTESIAN_POINT('Ctrl Pts',(-0.604198439271435,1.15978238118065,
2.23800734716904));
#27327=CARTESIAN_POINT('Ctrl Pts',(-0.469038667788838,1.09163604999709,
2.23015679613136));
#27328=CARTESIAN_POINT('Ctrl Pts',(-0.451328132598973,0.941308330848865,
2.22230624509368));
#27329=CARTESIAN_POINT('Ctrl Pts',(-0.56695006249535,0.843616695807582,
2.21445569405601));
#27330=CARTESIAN_POINT('Ctrl Pts',(-0.712211962098838,0.886173325824406,
2.20660514301833));
#27331=CARTESIAN_POINT('Ctrl Pts',(-0.756839506387522,1.0308124232748,2.19875459198065));
#27332=CARTESIAN_POINT('Ctrl Pts',(-0.660809652710606,1.14781820705317,
2.19090404094297));
#27333=CARTESIAN_POINT('Ctrl Pts',(-0.51024425681279,1.13225710850146,2.1830534899053));
#27334=CARTESIAN_POINT('Ctrl Pts',(-0.440173945225492,0.998084690937051,
2.17520293886762));
#27335=CARTESIAN_POINT('Ctrl Pts',(-0.513439439211253,0.865629967835047,
2.16735238782994));
#27336=CARTESIAN_POINT('Ctrl Pts',(-0.664334501961606,0.853681484510555,
2.15950183679226));
#27337=CARTESIAN_POINT('Ctrl Pts',(-0.757532853908686,0.972954923483646,
2.15165128575458));
#27338=CARTESIAN_POINT('Ctrl Pts',(-0.709451997299263,1.11648303183743,
2.1438007347169));
#27339=CARTESIAN_POINT('Ctrl Pts',(-0.563211987522275,1.15554638447572,
2.13595018367923));
#27340=CARTESIAN_POINT('Ctrl Pts',(-0.449964341757637,1.05511204856404,
2.12809963264155));
#27341=CARTESIAN_POINT('Ctrl Pts',(-0.471272241517894,0.905251903628159,
2.12024908160387));
#27342=CARTESIAN_POINT('Ctrl Pts',(-0.608026254784307,0.840364130860531,
2.11239853056619));
#27343=CARTESIAN_POINT('Ctrl Pts',(-0.737582133180516,0.918641547938033,
2.10454797952851));
#27344=CARTESIAN_POINT('Ctrl Pts',(-0.7437510812886,1.06988326260355,2.09669742849084));
#27345=CARTESIAN_POINT('Ctrl Pts',(-0.621000646973074,1.15845180245062,
2.08884687745316));
#27346=CARTESIAN_POINT('Ctrl Pts',(-0.479416323833351,1.10491739878753,
2.08099632641548));
#27347=CARTESIAN_POINT('Ctrl Pts',(-0.445974326577002,0.957289791901268,
2.0731457753778));
#27348=CARTESIAN_POINT('Ctrl Pts',(-0.550666178876061,0.847967258785586,
2.06529522434013));
#27349=CARTESIAN_POINT('Ctrl Pts',(-0.699601845773343,0.87498826919366,
2.05744467330245));
#27350=CARTESIAN_POINT('Ctrl Pts',(-0.759212070044963,1.01412873128603,
2.04959412226477));
#27351=CARTESIAN_POINT('Ctrl Pts',(-0.676037398789558,1.14058650207107,
2.04174357122709));
#27352=CARTESIAN_POINT('Ctrl Pts',(-0.524670042661485,1.14098596232722,
2.03389302018941));
#27353=CARTESIAN_POINT('Ctrl Pts',(-0.440861436985121,1.01490064771879,
2.02604246915174));
#27354=CARTESIAN_POINT('Ctrl Pts',(-0.49977004220855,0.875541008883831,
2.01819191811406));
#27355=CARTESIAN_POINT('Ctrl Pts',(-0.648570865797738,0.847623313273011,
2.01034136707638));
#27356=CARTESIAN_POINT('Ctrl Pts',(-0.753809411330851,0.956718503824468,
2.0024908160387));
#27357=CARTESIAN_POINT('Ctrl Pts',(-0.731974363173429,1.05475934582637,
1.99725711534692));
#27358=CARTESIAN_POINT('Ctrl Pts',(-0.702845629995664,1.08857942294107,
1.99464026500102));
#27359=CARTESIAN_POINT('Ctrl Pts',(-0.632658506353108,0.877840168374445,
2.41607920499693));
#27360=CARTESIAN_POINT('Ctrl Pts',(-0.672829925654731,0.888579693265874,
2.41346235465104));
#27361=CARTESIAN_POINT('Ctrl Pts',(-0.74109801777064,0.952575118838442,
2.40822865395925));
#27362=CARTESIAN_POINT('Ctrl Pts',(-0.717366779080126,1.09178093194185,
2.40037810292158));
#27363=CARTESIAN_POINT('Ctrl Pts',(-0.588188249850668,1.1484014586541,2.3925275518839));
#27364=CARTESIAN_POINT('Ctrl Pts',(-0.469697856816082,1.07206546854677,
2.38467700084622));
#27365=CARTESIAN_POINT('Ctrl Pts',(-0.468017275884308,0.931032076110704,
2.37682644980854));
#27366=CARTESIAN_POINT('Ctrl Pts',(-0.584726483104016,0.851885001647656,
2.36897589877086));
#27367=CARTESIAN_POINT('Ctrl Pts',(-0.715120852817283,0.905553554202683,
2.36112534773319));
#27368=CARTESIAN_POINT('Ctrl Pts',(-0.742278462016426,1.04393279284724,
2.35327479669551));
#27369=CARTESIAN_POINT('Ctrl Pts',(-0.641834128465295,1.14290754489126,
2.34542424565783));
#27370=CARTESIAN_POINT('Ctrl Pts',(-0.50387360072502,1.1137217104627,2.33757369462015));
#27371=CARTESIAN_POINT('Ctrl Pts',(-0.452120674984892,0.98254637331334,
2.32972314358248));
#27372=CARTESIAN_POINT('Ctrl Pts',(-0.532989870132326,0.867024458591828,
2.32187259254479));
#27373=CARTESIAN_POINT('Ctrl Pts',(-0.673955125704091,0.870757867844471,
2.31402204150712));
#27374=CARTESIAN_POINT('Ctrl Pts',(-0.748595776865795,0.990398847921281,
2.30617149046944));
#27375=CARTESIAN_POINT('Ctrl Pts',(-0.689972146429509,1.11865029097931,
2.29832093943176));
#27376=CARTESIAN_POINT('Ctrl Pts',(-0.550659384735185,1.14049337226976,
2.29047038839408));
#27377=CARTESIAN_POINT('Ctrl Pts',(-0.455596445247116,1.0363386369461,2.28261983735641));
#27378=CARTESIAN_POINT('Ctrl Pts',(-0.490038054074624,0.899594558451655,
2.27476928631873));
#27379=CARTESIAN_POINT('Ctrl Pts',(-0.623096146429573,0.852896461675674,
2.26691873528105));
#27380=CARTESIAN_POINT('Ctrl Pts',(-0.735441067507883,0.938124317935081,
2.25906818424337));
#27381=CARTESIAN_POINT('Ctrl Pts',(-0.726319218340423,1.07884375551639,
2.25121763320569));
#27382=CARTESIAN_POINT('Ctrl Pts',(-0.603911291595331,1.14885423944223,
2.24336708216802));
#27383=CARTESIAN_POINT('Ctrl Pts',(-0.477995625308683,1.08536870227504,
2.23551653113034));
#27384=CARTESIAN_POINT('Ctrl Pts',(-0.461496382862034,0.945322483564629,
2.22766598009266));
#27385=CARTESIAN_POINT('Ctrl Pts',(-0.569210476934212,0.854312361381646,
2.21981542905498));
#27386=CARTESIAN_POINT('Ctrl Pts',(-0.704537347304013,0.893958377091083,
2.21196487801731));
#27387=CARTESIAN_POINT('Ctrl Pts',(-0.746112639361755,1.02870504118196,
2.20411432697963));
#27388=CARTESIAN_POINT('Ctrl Pts',(-0.656650642818685,1.1377083419588,2.19626377594195));
#27389=CARTESIAN_POINT('Ctrl Pts',(-0.516383003000816,1.12321152777512,
2.18841322490427));
#27390=CARTESIAN_POINT('Ctrl Pts',(-0.451105073971734,0.998215686412011,
2.18056267386659));
#27391=CARTESIAN_POINT('Ctrl Pts',(-0.519359654383078,0.874820059671476,
2.17271212282892));
#27392=CARTESIAN_POINT('Ctrl Pts',(-0.659934413848564,0.863688779835656,
2.16486157179123));
#27393=CARTESIAN_POINT('Ctrl Pts',(-0.746758566135216,0.974804642002754,
2.15701102075356));
#27394=CARTESIAN_POINT('Ctrl Pts',(-0.701966147287513,1.1085163018849,2.14916046971588));
#27395=CARTESIAN_POINT('Ctrl Pts',(-0.565728063523024,1.14490795911313,
2.1413099186782));
#27396=CARTESIAN_POINT('Ctrl Pts',(-0.46022586700825,1.0513427200952,2.13345936764053));
#27397=CARTESIAN_POINT('Ctrl Pts',(-0.48007643619797,0.91173209636872,2.12560881660285));
#27398=CARTESIAN_POINT('Ctrl Pts',(-0.607477307839948,0.851282252067638,
2.11775826556517));
#27399=CARTESIAN_POINT('Ctrl Pts',(-0.728172353197516,0.924205970555728,
2.10990771452749));
#27400=CARTESIAN_POINT('Ctrl Pts',(-0.733919382826205,1.06510367305662,
2.10205716348981));
#27401=CARTESIAN_POINT('Ctrl Pts',(-0.619564330621895,1.14761466419362,
2.09420661245214));
#27402=CARTESIAN_POINT('Ctrl Pts',(-0.487663512883551,1.09774168769659,
2.08635606141446));
#27403=CARTESIAN_POINT('Ctrl Pts',(-0.456508744565289,0.960210910014111,
2.07850551037678));
#27404=CARTESIAN_POINT('Ctrl Pts',(-0.554040311779553,0.858365372348507,
2.0706549593391));
#27405=CARTESIAN_POINT('Ctrl Pts',(-0.692789686134866,0.883538310212708,
2.06280440830143));
#27406=CARTESIAN_POINT('Ctrl Pts',(-0.748322934114825,1.01316241211532,
2.05495385726374));
#27407=CARTESIAN_POINT('Ctrl Pts',(-0.670836903808495,1.13097124155368,
2.04710330622607));
#27408=CARTESIAN_POINT('Ctrl Pts',(-0.529822152955879,1.13134338116118,
2.03925275518839));
#27409=CARTESIAN_POINT('Ctrl Pts',(-0.451745545482087,1.01388153416533,
2.03140220415071));
#27410=CARTESIAN_POINT('Ctrl Pts',(-0.506625160883627,0.884053245874464,
2.02355165311303));
#27411=CARTESIAN_POINT('Ctrl Pts',(-0.645248914391877,0.858044950614234,
2.01570110207536));
#27412=CARTESIAN_POINT('Ctrl Pts',(-0.743289784352549,0.959678694562408,
2.00785055103768));
#27413=CARTESIAN_POINT('Ctrl Pts',(-0.722948120505502,1.0510141400767,2.00261685034589));
#27414=CARTESIAN_POINT('Ctrl Pts',(-0.695811615272238,1.08252112989365,
2.));
#27415=CARTESIAN_POINT('Ctrl Pts',(-0.695811615272238,1.08252112989365,
2.));
#27416=CARTESIAN_POINT('Ctrl Pts',(-0.702493043757975,1.07628156364939,
2.));
#27417=CARTESIAN_POINT('Ctrl Pts',(-0.708395726655653,1.06931034161853,
2.));
#27418=CARTESIAN_POINT('Ctrl Pts',(-0.713512684042454,1.06178682515746,
2.));
#27419=CARTESIAN_POINT('Ctrl Pts',(-0.717502373507965,1.05592074262065,
2.));
#27420=CARTESIAN_POINT('Ctrl Pts',(-0.721014109525759,1.04971755287119,
2.));
#27421=CARTESIAN_POINT('Ctrl Pts',(-0.724031985841351,1.04324617113496,
2.));
#27422=CARTESIAN_POINT('Ctrl Pts',(-0.72532920883522,1.04046447158453,2.));
#27423=CARTESIAN_POINT('Ctrl Pts',(-0.726532666614568,1.03763771042115,
2.));
#27424=CARTESIAN_POINT('Ctrl Pts',(-0.727638826408048,1.0347790826819,2.));
#27425=CARTESIAN_POINT('Ctrl Pts',(-0.731193005346523,1.0255940855742,2.));
#27426=CARTESIAN_POINT('Ctrl Pts',(-0.733756270098347,1.01606060371262,
2.));
#27427=CARTESIAN_POINT('Ctrl Pts',(-0.73529467500939,1.0063604242084,2.));
#27428=CARTESIAN_POINT('Ctrl Pts',(-0.736007760405585,1.00186417208695,
2.));
#27429=CARTESIAN_POINT('Ctrl Pts',(-0.736500058162718,0.997331645993815,
2.));
#27430=CARTESIAN_POINT('Ctrl Pts',(-0.736764718140032,0.992779414308968,
2.));
#27431=CARTESIAN_POINT('Ctrl Pts',(-0.736959136386439,0.989435361647935,
2.));
#27432=CARTESIAN_POINT('Ctrl Pts',(-0.737030047799371,0.986088140051384,
2.));
#27433=CARTESIAN_POINT('Ctrl Pts',(-0.736976193579456,0.982751455795261,
2.));
#27434=CARTESIAN_POINT('Ctrl Pts',(-0.73686292459887,0.975733568899372,
2.));
#27435=CARTESIAN_POINT('Ctrl Pts',(-0.736199092496592,0.968753171717965,
2.));
#27436=CARTESIAN_POINT('Ctrl Pts',(-0.734968654150234,0.961871622922131,
2.));
#27437=CARTESIAN_POINT('Ctrl Pts',(-0.733610341240648,0.954274902131536,
2.));
#27438=CARTESIAN_POINT('Ctrl Pts',(-0.731561985767923,0.946798189069373,
2.));
#27439=CARTESIAN_POINT('Ctrl Pts',(-0.728883458720402,0.939498582185105,
2.));
#27440=CARTESIAN_POINT('Ctrl Pts',(-0.727748853408495,0.936406519794552,
2.));
#27441=CARTESIAN_POINT('Ctrl Pts',(-0.726503727419379,0.933354179904992,
2.));
#27442=CARTESIAN_POINT('Ctrl Pts',(-0.725155499563838,0.930349726147835,
2.));
#27443=CARTESIAN_POINT('Ctrl Pts',(-0.721333577255107,0.921832776440231,
2.));
#27444=CARTESIAN_POINT('Ctrl Pts',(-0.716682008196949,0.913689860477865,
2.));
#27445=CARTESIAN_POINT('Ctrl Pts',(-0.711310122504209,0.906016289602163,
2.));
#27446=CARTESIAN_POINT('Ctrl Pts',(-0.708434363463016,0.901908357660524,
2.));
#27447=CARTESIAN_POINT('Ctrl Pts',(-0.705351534711708,0.897934993684464,
2.));
#27448=CARTESIAN_POINT('Ctrl Pts',(-0.702074554712817,0.894112147617013,
2.));
#27449=CARTESIAN_POINT('Ctrl Pts',(-0.699663476442214,0.891299441684046,
2.));
#27450=CARTESIAN_POINT('Ctrl Pts',(-0.69714655627776,0.888568031452597,
2.));
#27451=CARTESIAN_POINT('Ctrl Pts',(-0.694540241228364,0.885935594383534,
2.));
#27452=CARTESIAN_POINT('Ctrl Pts',(-0.68996701323731,0.881316530816482,
2.));
#27453=CARTESIAN_POINT('Ctrl Pts',(-0.685111619991385,0.87699300942471,
2.));
#27454=CARTESIAN_POINT('Ctrl Pts',(-0.680004202609246,0.872997619450478,
2.));
#27455=CARTESIAN_POINT('Ctrl Pts',(-0.67522861092298,0.869261807450647,
2.));
#27456=CARTESIAN_POINT('Ctrl Pts',(-0.670227038735164,0.865810222770729,
2.));
#27457=CARTESIAN_POINT('Ctrl Pts',(-0.66504978274748,0.862688963354369,
2.));
#27458=CARTESIAN_POINT('Ctrl Pts',(-0.659173901912074,0.859146517620461,
2.));
#27459=CARTESIAN_POINT('Ctrl Pts',(-0.653067296294555,0.856024686886556,
2.));
#27460=CARTESIAN_POINT('Ctrl Pts',(-0.64676194038029,0.853364152629858,
2.));
#27461=CARTESIAN_POINT('Ctrl Pts',(-0.644516589878667,0.85241673078578,
2.));
#27462=CARTESIAN_POINT('Ctrl Pts',(-0.642245983976318,0.851527865406908,
2.));
#27463=CARTESIAN_POINT('Ctrl Pts',(-0.639952236162157,0.850696980524378,
2.));
#27464=CARTESIAN_POINT('Ctrl Pts',(-0.726369333664333,1.00010094057762,
2.35565803263806));
#27465=CARTESIAN_POINT('Ctrl Pts',(-0.726467565903334,1.01274184217687,
2.35486362065721));
#27466=CARTESIAN_POINT('Ctrl Pts',(-0.724719482090242,1.02535623071191,
2.35406920867636));
#27467=CARTESIAN_POINT('Ctrl Pts',(-0.721011471558047,1.03736537841382,
2.35327479669551));
#27468=CARTESIAN_POINT('Ctrl Pts',(-0.708797017499383,1.07692437686191,
2.35065794634961));
#27469=CARTESIAN_POINT('Ctrl Pts',(-0.675315572982339,1.10991596087659,
2.34804109600372));
#27470=CARTESIAN_POINT('Ctrl Pts',(-0.635581429433771,1.12154744714583,
2.34542424565783));
#27471=CARTESIAN_POINT('Ctrl Pts',(-0.595847285885203,1.13317893341507,
2.34280739531194));
#27472=CARTESIAN_POINT('Ctrl Pts',(-0.549860443305111,1.12345032193889,
2.34019054496604));
#27473=CARTESIAN_POINT('Ctrl Pts',(-0.518241534391711,1.09672346000923,
2.33757369462015));
#27474=CARTESIAN_POINT('Ctrl Pts',(-0.486622625478311,1.06999659807958,
2.33495684427426));
#27475=CARTESIAN_POINT('Ctrl Pts',(-0.469371650231601,1.02627148569646,
2.33233999392837));
#27476=CARTESIAN_POINT('Ctrl Pts',(-0.474224361799485,0.985155277051315,
2.32972314358247));
#27477=CARTESIAN_POINT('Ctrl Pts',(-0.47907707336737,0.944039068406169,
2.32710629323658));
#27478=CARTESIAN_POINT('Ctrl Pts',(-0.506033471749848,0.905531763498998,
2.32448944289069));
#27479=CARTESIAN_POINT('Ctrl Pts',(-0.543005880203048,0.886900345920854,
2.3218725925448));
#27480=CARTESIAN_POINT('Ctrl Pts',(-0.579978288656248,0.868268928342709,
2.3192557421989));
#27481=CARTESIAN_POINT('Ctrl Pts',(-0.62696670718017,0.86951339809359,2.31663889185301));
#27482=CARTESIAN_POINT('Ctrl Pts',(-0.662901024969081,0.890075796315165,
2.31402204150712));
#27483=CARTESIAN_POINT('Ctrl Pts',(-0.698835342757992,0.910638194536741,
2.31140519116123));
#27484=CARTESIAN_POINT('Ctrl Pts',(-0.723715559811894,0.950518521229011,
2.30878834081533));
#27485=CARTESIAN_POINT('Ctrl Pts',(-0.72638506326613,0.991833925084817,
2.30617149046944));
#27486=CARTESIAN_POINT('Ctrl Pts',(-0.726559659603113,0.994536119817981,
2.30600033785898));
#27487=CARTESIAN_POINT('Ctrl Pts',(-0.726639245398498,0.997244453365998,
2.30582918524852));
#27488=CARTESIAN_POINT('Ctrl Pts',(-0.726626272216059,0.999953562434948,
2.30565803263806));
#27489=CARTESIAN_POINT('Ctrl Pts',(-0.639851384185722,0.850935057178148,
2.4));
#27490=CARTESIAN_POINT('Ctrl Pts',(-0.649880557039356,0.854599675659919,
2.4));
#27491=CARTESIAN_POINT('Ctrl Pts',(-0.659434997625568,0.85936263163469,
2.4));
#27492=CARTESIAN_POINT('Ctrl Pts',(-0.668403171068605,0.865074092345247,
2.4));
#27493=CARTESIAN_POINT('Ctrl Pts',(-0.672868373471587,0.86791779605496,
2.4));
#27494=CARTESIAN_POINT('Ctrl Pts',(-0.67718781684999,0.870997354370473,
2.4));
#27495=CARTESIAN_POINT('Ctrl Pts',(-0.681344478651501,0.874297577803816,
2.4));
#27496=CARTESIAN_POINT('Ctrl Pts',(-0.684149819111287,0.8765249060701,2.4));
#27497=CARTESIAN_POINT('Ctrl Pts',(-0.686880965099162,0.878852785859471,
2.4));
#27498=CARTESIAN_POINT('Ctrl Pts',(-0.689531958931665,0.88127688968642,
2.4));
#27499=CARTESIAN_POINT('Ctrl Pts',(-0.691903137355438,0.883445126602317,
2.4));
#27500=CARTESIAN_POINT('Ctrl Pts',(-0.694203487834536,0.885684268626149,
2.4));
#27501=CARTESIAN_POINT('Ctrl Pts',(-0.696428596284293,0.887989081198335,
2.4));
#27502=CARTESIAN_POINT('Ctrl Pts',(-0.703655665265446,0.895475026186606,
2.4));
#27503=CARTESIAN_POINT('Ctrl Pts',(-0.710097115492295,0.903656379805453,
2.4));
#27504=CARTESIAN_POINT('Ctrl Pts',(-0.715619698888934,0.91241311638882,
2.4));
#27505=CARTESIAN_POINT('Ctrl Pts',(-0.717914152011463,0.916051254584994,
2.4));
#27506=CARTESIAN_POINT('Ctrl Pts',(-0.720049438182606,0.919788953917886,
2.4));
#27507=CARTESIAN_POINT('Ctrl Pts',(-0.722013340315698,0.923618244020841,
2.4));
#27508=CARTESIAN_POINT('Ctrl Pts',(-0.723497106826098,0.926511347662634,
2.4));
#27509=CARTESIAN_POINT('Ctrl Pts',(-0.724882791677009,0.929457049049758,
2.4));
#27510=CARTESIAN_POINT('Ctrl Pts',(-0.726159625039968,0.932438198899027,
2.4));
#27511=CARTESIAN_POINT('Ctrl Pts',(-0.7293219265251,0.939821538706109,2.4));
#27512=CARTESIAN_POINT('Ctrl Pts',(-0.731828922840258,0.947441945091078,
2.4));
#27513=CARTESIAN_POINT('Ctrl Pts',(-0.733609784156052,0.955243638029731,
2.4));
#27514=CARTESIAN_POINT('Ctrl Pts',(-0.735247937517986,0.962420148296355,
2.4));
#27515=CARTESIAN_POINT('Ctrl Pts',(-0.736271216774028,0.969750560405923,
2.4));
#27516=CARTESIAN_POINT('Ctrl Pts',(-0.736691013623241,0.977159425155101,
2.4));
#27517=CARTESIAN_POINT('Ctrl Pts',(-0.736867157952635,0.980268141943398,
2.4));
#27518=CARTESIAN_POINT('Ctrl Pts',(-0.736936476729183,0.983387171734525,
2.4));
#27519=CARTESIAN_POINT('Ctrl Pts',(-0.736900577814768,0.986501043637764,
2.4));
#27520=CARTESIAN_POINT('Ctrl Pts',(-0.73680325432052,0.994942883710025,
2.4));
#27521=CARTESIAN_POINT('Ctrl Pts',(-0.735935887531182,1.00336876050526,
2.4));
#27522=CARTESIAN_POINT('Ctrl Pts',(-0.73432454218896,1.01166505164342,2.4));
#27523=CARTESIAN_POINT('Ctrl Pts',(-0.733128713302574,1.01782198419718,
2.4));
#27524=CARTESIAN_POINT('Ctrl Pts',(-0.731522518607655,1.02390757353733,
2.4));
#27525=CARTESIAN_POINT('Ctrl Pts',(-0.729508194962256,1.0298701636783,2.4));
#27526=CARTESIAN_POINT('Ctrl Pts',(-0.728322998806314,1.03337845735825,
2.4));
#27527=CARTESIAN_POINT('Ctrl Pts',(-0.726998704692332,1.03683671166907,
2.4));
#27528=CARTESIAN_POINT('Ctrl Pts',(-0.72553907497761,1.04022912662095,2.4));
#27529=CARTESIAN_POINT('Ctrl Pts',(-0.723248641788982,1.04555246288699,
2.4));
#27530=CARTESIAN_POINT('Ctrl Pts',(-0.720623684757818,1.05071851440316,
2.4));
#27531=CARTESIAN_POINT('Ctrl Pts',(-0.717666939943194,1.055684952745,2.4));
#27532=CARTESIAN_POINT('Ctrl Pts',(-0.715625486572472,1.05911397788213,
2.4));
#27533=CARTESIAN_POINT('Ctrl Pts',(-0.713425317203702,1.06244758415869,
2.4));
#27534=CARTESIAN_POINT('Ctrl Pts',(-0.711075718450412,1.06565920682025,
2.4));
#27535=CARTESIAN_POINT('Ctrl Pts',(-0.707783291943712,1.07015956313241,
2.4));
#27536=CARTESIAN_POINT('Ctrl Pts',(-0.704194030655052,1.07442716580257,
2.4));
#27537=CARTESIAN_POINT('Ctrl Pts',(-0.700309061659577,1.07842077162732,
2.4));
#27538=CARTESIAN_POINT('Ctrl Pts',(-0.69890728532317,1.07986174635546,2.4));
#27539=CARTESIAN_POINT('Ctrl Pts',(-0.697466969165074,1.08126698735129,
2.4));
#27540=CARTESIAN_POINT('Ctrl Pts',(-0.695989827719556,1.08263574823442,
2.4));
#27541=CARTESIAN_POINT('Origin',(0.,0.,2.));
#27542=CARTESIAN_POINT('',(-0.8,0.6,2.));
#27543=CARTESIAN_POINT('',(0.8,0.6,2.));
#27544=CARTESIAN_POINT('Origin',(0.,0.,2.));
#27545=CARTESIAN_POINT('',(-1.8,0.6,2.));
#27546=CARTESIAN_POINT('',(-1.8,0.6,2.));
#27547=CARTESIAN_POINT('',(-1.8,1.4,2.));
#27548=CARTESIAN_POINT('',(-1.8,1.4,2.));
#27549=CARTESIAN_POINT('',(1.8,1.4,2.));
#27550=CARTESIAN_POINT('',(1.8,1.4,2.));
#27551=CARTESIAN_POINT('',(1.8,0.6,2.));
#27552=CARTESIAN_POINT('',(1.8,0.6,2.));
#27553=CARTESIAN_POINT('',(-1.8,0.6,2.));
#27554=CARTESIAN_POINT('Ctrl Pts',(0.504188384727762,1.08252112989365,2.));
#27555=CARTESIAN_POINT('Ctrl Pts',(0.497506952411728,1.07628156007241,2.));
#27556=CARTESIAN_POINT('Ctrl Pts',(0.491604265140002,1.06931033514179,2.));
#27557=CARTESIAN_POINT('Ctrl Pts',(0.486487303479808,1.06178681610824,2.));
#27558=CARTESIAN_POINT('Ctrl Pts',(0.482497614326221,1.0559207369233,2.));
#27559=CARTESIAN_POINT('Ctrl Pts',(0.478985877807952,1.04971755133896,2.));
#27560=CARTESIAN_POINT('Ctrl Pts',(0.47596800043997,1.04324617422688,2.));
#27561=CARTESIAN_POINT('Ctrl Pts',(0.474670775798635,1.04046447410142,2.));
#27562=CARTESIAN_POINT('Ctrl Pts',(0.473467316455455,1.03763771239116,2.));
#27563=CARTESIAN_POINT('Ctrl Pts',(0.472361155190705,1.03477908408591,2.));
#27564=CARTESIAN_POINT('Ctrl Pts',(0.468806973334995,1.02559408983729,2.));
#27565=CARTESIAN_POINT('Ctrl Pts',(0.466243705645806,1.01606061108597,2.));
#27566=CARTESIAN_POINT('Ctrl Pts',(0.464705298489784,1.00636043426204,2.));
#27567=CARTESIAN_POINT('Ctrl Pts',(0.463992209982944,1.00186417033063,2.));
#27568=CARTESIAN_POINT('Ctrl Pts',(0.463499910544365,0.997331632125338,
2.));
#27569=CARTESIAN_POINT('Ctrl Pts',(0.463235250450622,0.992779388102766,
2.));
#27570=CARTESIAN_POINT('Ctrl Pts',(0.463040833672037,0.989435353096635,
2.));
#27571=CARTESIAN_POINT('Ctrl Pts',(0.46296992260639,0.986088149337579,2.));
#27572=CARTESIAN_POINT('Ctrl Pts',(0.46302377604218,0.982751482606387,2.));
#27573=CARTESIAN_POINT('Ctrl Pts',(0.463137043908312,0.975733599437203,
2.));
#27574=CARTESIAN_POINT('Ctrl Pts',(0.463800875129207,0.968753205425666,
2.));
#27575=CARTESIAN_POINT('Ctrl Pts',(0.465031313050322,0.961871658945486,
2.));
#27576=CARTESIAN_POINT('Ctrl Pts',(0.466389625771061,0.954274939141924,
2.));
#27577=CARTESIAN_POINT('Ctrl Pts',(0.468437981894213,0.946798226077515,
2.));
#27578=CARTESIAN_POINT('Ctrl Pts',(0.471116510174533,0.93949861845872,2.));
#27579=CARTESIAN_POINT('Ctrl Pts',(0.472251116178103,0.936406555295212,
2.));
#27580=CARTESIAN_POINT('Ctrl Pts',(0.473496242998671,0.933354214505235,
2.));
#27581=CARTESIAN_POINT('Ctrl Pts',(0.474844471797333,0.930349759755262,
2.));
#27582=CARTESIAN_POINT('Ctrl Pts',(0.478666396590115,0.921832807655503,
2.));
#27583=CARTESIAN_POINT('Ctrl Pts',(0.483317968956197,0.913689888494062,
2.));
#27584=CARTESIAN_POINT('Ctrl Pts',(0.488689858313544,0.906016314077791,
2.));
#27585=CARTESIAN_POINT('Ctrl Pts',(0.491565612706781,0.90190838968258,2.));
#27586=CARTESIAN_POINT('Ctrl Pts',(0.494648435962255,0.897935032536209,
2.));
#27587=CARTESIAN_POINT('Ctrl Pts',(0.497925409635587,0.894112192538158,
2.));
#27588=CARTESIAN_POINT('Ctrl Pts',(0.500336494700513,0.891299477715359,
2.));
#27589=CARTESIAN_POINT('Ctrl Pts',(0.502853422244813,0.888568058918467,
2.));
#27590=CARTESIAN_POINT('Ctrl Pts',(0.505459745106002,0.885935613780059,
2.));
#27591=CARTESIAN_POINT('Ctrl Pts',(0.510032972332535,0.881316550670653,
2.));
#27592=CARTESIAN_POINT('Ctrl Pts',(0.514888364383629,0.876993029350264,
2.));
#27593=CARTESIAN_POINT('Ctrl Pts',(0.519995780056594,0.872997639132679,
2.));
#27594=CARTESIAN_POINT('Ctrl Pts',(0.52477137880872,0.869261820127707,2.));
#27595=CARTESIAN_POINT('Ctrl Pts',(0.529772958435197,0.865810229192487,
2.));
#27596=CARTESIAN_POINT('Ctrl Pts',(0.534950221975527,0.862688964531106,
2.));
#27597=CARTESIAN_POINT('Ctrl Pts',(0.540826105312277,0.859146516504166,
2.));
#27598=CARTESIAN_POINT('Ctrl Pts',(0.546932713096854,0.856024683905292,
2.));
#27599=CARTESIAN_POINT('Ctrl Pts',(0.553238070670066,0.853364148387157,
2.));
#27600=CARTESIAN_POINT('Ctrl Pts',(0.55548342158471,0.852416726168872,2.));
#27601=CARTESIAN_POINT('Ctrl Pts',(0.55775402783163,0.851527860483116,2.));
#27602=CARTESIAN_POINT('Ctrl Pts',(0.560047775926793,0.850696975355778,
2.));
#27603=CARTESIAN_POINT('Ctrl Pts',(0.639851384185725,0.850935057178149,
2.));
#27604=CARTESIAN_POINT('Ctrl Pts',(0.649880550625801,0.854599673316433,
2.));
#27605=CARTESIAN_POINT('Ctrl Pts',(0.659434984589242,0.859362630571034,
2.));
#27606=CARTESIAN_POINT('Ctrl Pts',(0.668403151796856,0.865074094293816,
2.));
#27607=CARTESIAN_POINT('Ctrl Pts',(0.672868418174611,0.867917842223432,
2.));
#27608=CARTESIAN_POINT('Ctrl Pts',(0.677187921251714,0.870997452272092,
2.));
#27609=CARTESIAN_POINT('Ctrl Pts',(0.68134463777063,0.874297734044997,2.));
#27610=CARTESIAN_POINT('Ctrl Pts',(0.684149977150149,0.876525071506887,
2.));
#27611=CARTESIAN_POINT('Ctrl Pts',(0.686881121795098,0.878852960779101,
2.));
#27612=CARTESIAN_POINT('Ctrl Pts',(0.689532114008666,0.881277074288136,
2.));
#27613=CARTESIAN_POINT('Ctrl Pts',(0.691903244332041,0.883445277204446,
2.));
#27614=CARTESIAN_POINT('Ctrl Pts',(0.694203548662863,0.885684381973589,
2.));
#27615=CARTESIAN_POINT('Ctrl Pts',(0.696428614090338,0.88798915510679,2.));
#27616=CARTESIAN_POINT('Ctrl Pts',(0.703655681573731,0.895475115187732,
2.));
#27617=CARTESIAN_POINT('Ctrl Pts',(0.710097129721786,0.903656484453022,
2.));
#27618=CARTESIAN_POINT('Ctrl Pts',(0.715619710640267,0.912413235085866,
2.));
#27619=CARTESIAN_POINT('Ctrl Pts',(0.717914173550032,0.916051396270592,
2.));
#27620=CARTESIAN_POINT('Ctrl Pts',(0.720049467939456,0.919789119253813,
2.));
#27621=CARTESIAN_POINT('Ctrl Pts',(0.722013376555431,0.923618433392056,
2.));
#27622=CARTESIAN_POINT('Ctrl Pts',(0.723497129119939,0.926511518450447,
2.));
#27623=CARTESIAN_POINT('Ctrl Pts',(0.724882801444961,0.929457199976584,
2.));
#27624=CARTESIAN_POINT('Ctrl Pts',(0.726159624011702,0.932438329054375,
2.));
#27625=CARTESIAN_POINT('Ctrl Pts',(0.729321918563565,0.939821663659088,
2.));
#27626=CARTESIAN_POINT('Ctrl Pts',(0.731828910123054,0.947442062000798,
2.));
#27627=CARTESIAN_POINT('Ctrl Pts',(0.733609769329411,0.955243743262114,
2.));
#27628=CARTESIAN_POINT('Ctrl Pts',(0.735247922763181,0.962420251602462,
2.));
#27629=CARTESIAN_POINT('Ctrl Pts',(0.736271202825978,0.969750659080777,
2.));
#27630=CARTESIAN_POINT('Ctrl Pts',(0.736691001072906,0.977159517273332,
2.));
#27631=CARTESIAN_POINT('Ctrl Pts',(0.736867146035702,0.980268232138734,
2.));
#27632=CARTESIAN_POINT('Ctrl Pts',(0.736936465492878,0.983387259690693,
2.));
#27633=CARTESIAN_POINT('Ctrl Pts',(0.736900567292279,0.986501129084147,
2.));
#27634=CARTESIAN_POINT('Ctrl Pts',(0.736803245735092,0.994942962189629,
2.));
#27635=CARTESIAN_POINT('Ctrl Pts',(0.73593588116366,1.00336883005034,2.));
#27636=CARTESIAN_POINT('Ctrl Pts',(0.734324538110121,1.01166511142386,2.));
#27637=CARTESIAN_POINT('Ctrl Pts',(0.733128714763866,1.01782201695168,2.));
#27638=CARTESIAN_POINT('Ctrl Pts',(0.731522528281544,1.02390757926145,2.));
#27639=CARTESIAN_POINT('Ctrl Pts',(0.729508215420297,1.02987014335002,2.));
#27640=CARTESIAN_POINT('Ctrl Pts',(0.728323015262132,1.03337845233062,2.));
#27641=CARTESIAN_POINT('Ctrl Pts',(0.726998715515976,1.03683672165704,2.));
#27642=CARTESIAN_POINT('Ctrl Pts',(0.725539078662676,1.04022915093548,2.));
#27643=CARTESIAN_POINT('Ctrl Pts',(0.723248638897094,1.04555249893377,2.));
#27644=CARTESIAN_POINT('Ctrl Pts',(0.72062367285432,1.05071856137362,2.));
#27645=CARTESIAN_POINT('Ctrl Pts',(0.717666916538866,1.05568500977016,2.));
#27646=CARTESIAN_POINT('Ctrl Pts',(0.71562546757316,1.05911402111255,2.));
#27647=CARTESIAN_POINT('Ctrl Pts',(0.713425303385499,1.06244761425647,2.));
#27648=CARTESIAN_POINT('Ctrl Pts',(0.711075710473028,1.06565922484506,2.));
#27649=CARTESIAN_POINT('Ctrl Pts',(0.707783289804617,1.0701595674468,2.));
#27650=CARTESIAN_POINT('Ctrl Pts',(0.704194035235276,1.07442715810878,2.));
#27651=CARTESIAN_POINT('Ctrl Pts',(0.700309073757905,1.07842075422663,2.));
#27652=CARTESIAN_POINT('Ctrl Pts',(0.698907297616712,1.07986172804018,2.));
#27653=CARTESIAN_POINT('Ctrl Pts',(0.697466981619643,1.08126696829348,2.));
#27654=CARTESIAN_POINT('Ctrl Pts',(0.695989840302895,1.08263572859343,2.));
#27655=CARTESIAN_POINT('Origin',(0.6,1.,2.51042117235887));
#27656=CARTESIAN_POINT('Ctrl Pts',(0.445511859130131,1.0000741974826,2.38542117235887));
#27657=CARTESIAN_POINT('Ctrl Pts',(0.445481645904189,1.00486660347515,2.38517311518799));
#27658=CARTESIAN_POINT('Ctrl Pts',(0.447840382858598,1.06018738535655,2.38230820767121));
#27659=CARTESIAN_POINT('Ctrl Pts',(0.514365803623529,1.16027111832567,2.37682644980854));
#27660=CARTESIAN_POINT('Ctrl Pts',(0.686438402045863,1.1598170503231,2.36897589877086));
#27661=CARTESIAN_POINT('Ctrl Pts',(0.780990355889297,1.01606136385454,2.36112534773319));
#27662=CARTESIAN_POINT('Ctrl Pts',(0.713226176840859,0.857888178208998,
2.35327479669551));
#27663=CARTESIAN_POINT('Ctrl Pts',(0.54391790721615,0.827171013394288,2.34542424565783));
#27664=CARTESIAN_POINT('Ctrl Pts',(0.453699048722976,0.921380393628473,
2.33947303754562));
#27665=CARTESIAN_POINT('Ctrl Pts',(0.445641803334383,0.985947130304853,
2.3361386797793));
#27666=CARTESIAN_POINT('Ctrl Pts',(0.445758404806891,0.999869526120069,
2.33542117235887));
#27667=CARTESIAN_POINT('Ctrl Pts',(0.445864724392684,0.99983533609866,2.38957882764113));
#27668=CARTESIAN_POINT('Ctrl Pts',(0.446099244735942,1.0340318743782,2.38781885106897));
#27669=CARTESIAN_POINT('Ctrl Pts',(0.47398874803022,1.11953643095444,2.38344202415091));
#27670=CARTESIAN_POINT('Ctrl Pts',(0.614413228882944,1.18108612135922,2.37644834688697));
#27671=CARTESIAN_POINT('Ctrl Pts',(0.759000551270414,1.08793755388759,2.36859779584929));
#27672=CARTESIAN_POINT('Ctrl Pts',(0.761051274433651,0.91584221771742,2.36074724481161));
#27673=CARTESIAN_POINT('Ctrl Pts',(0.618637433005314,0.819263404514795,
2.35289669377393));
#27674=CARTESIAN_POINT('Ctrl Pts',(0.475625295654385,0.878125251073759,
2.34584055471711));
#27675=CARTESIAN_POINT('Ctrl Pts',(0.446073423867575,0.964737113217481,
2.34140126600617));
#27676=CARTESIAN_POINT('Ctrl Pts',(0.445798439227784,1.00012317213786,2.33957882764113));
#27677=CARTESIAN_POINT('Ctrl Pts',(0.695811615272236,1.08252112989365,2.4));
#27678=CARTESIAN_POINT('Ctrl Pts',(0.7229481205055,1.0510141400767,2.39738314965411));
#27679=CARTESIAN_POINT('Ctrl Pts',(0.743289653273766,0.959678556377187,
2.39214944896232));
#27680=CARTESIAN_POINT('Ctrl Pts',(0.645248987396393,0.85804501052042,2.38429889792465));
#27681=CARTESIAN_POINT('Ctrl Pts',(0.506625118128944,0.884053189554221,
2.37644834688697));
#27682=CARTESIAN_POINT('Ctrl Pts',(0.45174554898112,1.01388156392493,2.36859779584929));
#27683=CARTESIAN_POINT('Ctrl Pts',(0.529822137836651,1.13134337597071,2.36074724481161));
#27684=CARTESIAN_POINT('Ctrl Pts',(0.670836914703171,1.13097126385843,2.35289669377393));
#27685=CARTESIAN_POINT('Ctrl Pts',(0.748322945574864,1.01316240738436,2.34504614273625));
#27686=CARTESIAN_POINT('Ctrl Pts',(0.692789695797321,0.883538302880933,
2.33719559169858));
#27687=CARTESIAN_POINT('Ctrl Pts',(0.554040306983033,0.858365357379829,
2.3293450406609));
#27688=CARTESIAN_POINT('Ctrl Pts',(0.456508731628746,0.960210907421746,
2.32149448962322));
#27689=CARTESIAN_POINT('Ctrl Pts',(0.487663502390397,1.09774169610628,2.31364393858554));
#27690=CARTESIAN_POINT('Ctrl Pts',(0.619564332496711,1.14761467812196,2.30579338754787));
#27691=CARTESIAN_POINT('Ctrl Pts',(0.733919395128131,1.0651036788751,2.29794283651019));
#27692=CARTESIAN_POINT('Ctrl Pts',(0.728172365024857,0.924205963670542,
2.29009228547251));
#27693=CARTESIAN_POINT('Ctrl Pts',(0.607477308519567,0.851282238312653,
2.28224173443483));
#27694=CARTESIAN_POINT('Ctrl Pts',(0.480076425153724,0.911732088265042,
2.27439118339715));
#27695=CARTESIAN_POINT('Ctrl Pts',(0.46022585412805,1.05134272481009,2.26654063235948));
#27696=CARTESIAN_POINT('Ctrl Pts',(0.565728060366633,1.14490797247226,2.2586900813218));
#27697=CARTESIAN_POINT('Ctrl Pts',(0.701966156681371,1.1085163118784,2.25083953028412));
#27698=CARTESIAN_POINT('Ctrl Pts',(0.746758579656851,0.974804639683806,
2.24298897924644));
#27699=CARTESIAN_POINT('Ctrl Pts',(0.659934419370361,0.863688767275607,
2.23513842820876));
#27700=CARTESIAN_POINT('Ctrl Pts',(0.519359646953508,0.874820048138925,
2.22728787717109));
#27701=CARTESIAN_POINT('Ctrl Pts',(0.451105060253533,0.998215686247253,
2.21943732613341));
#27702=CARTESIAN_POINT('Ctrl Pts',(0.516382995296938,1.12321153912718,2.21158677509573));
#27703=CARTESIAN_POINT('Ctrl Pts',(0.656650648038066,1.13770835464619,2.20373622405805));
#27704=CARTESIAN_POINT('Ctrl Pts',(0.746112652823594,1.02870504382673,2.19588567302037));
#27705=CARTESIAN_POINT('Ctrl Pts',(0.704537356935342,0.893958367321059,
2.1880351219827));
#27706=CARTESIAN_POINT('Ctrl Pts',(0.569210474097529,0.854312347959086,
2.18018457094502));
#27707=CARTESIAN_POINT('Ctrl Pts',(0.461496370101168,0.945322478526838,
2.17233401990734));
#27708=CARTESIAN_POINT('Ctrl Pts',(0.477995614068202,1.08536871014064,2.16448346886966));
#27709=CARTESIAN_POINT('Ctrl Pts',(0.603911291955373,1.14885425315604,2.15663291783199));
#27710=CARTESIAN_POINT('Ctrl Pts',(0.726319229979197,1.07884376278165,2.14878236679431));
#27711=CARTESIAN_POINT('Ctrl Pts',(0.73544107998541,0.938124312232147,2.14093181575663));
#27712=CARTESIAN_POINT('Ctrl Pts',(0.623096148559508,0.852896448126576,
2.13308126471895));
#27713=CARTESIAN_POINT('Ctrl Pts',(0.490038043939787,0.899594549193445,
2.12523071368128));
#27714=CARTESIAN_POINT('Ctrl Pts',(0.455596431949525,1.03633864030821,2.11738016264359));
#27715=CARTESIAN_POINT('Ctrl Pts',(0.550659380176962,1.14049338518748,2.10952961160592));
#27716=CARTESIAN_POINT('Ctrl Pts',(0.689972154741195,1.11865030196008,2.10167906056824));
#27717=CARTESIAN_POINT('Ctrl Pts',(0.748595790516416,0.990398846945399,
2.09382850953056));
#27718=CARTESIAN_POINT('Ctrl Pts',(0.673955132588938,0.870757856106032,
2.08597795849288));
#27719=CARTESIAN_POINT('Ctrl Pts',(0.532989863833319,0.867024446028552,
2.0781274074552));
#27720=CARTESIAN_POINT('Ctrl Pts',(0.45212066157753,0.982546372277999,2.07027685641753));
#27721=CARTESIAN_POINT('Ctrl Pts',(0.503873591498137,1.11372171989345,2.06242630537985));
#27722=CARTESIAN_POINT('Ctrl Pts',(0.641834132936712,1.14290755996024,2.05457575434217));
#27723=CARTESIAN_POINT('Ctrl Pts',(0.742278474130153,1.04393279346011,2.04672520330449));
#27724=CARTESIAN_POINT('Ctrl Pts',(0.71512086495066,0.905553551654031,2.03887465226682));
#27725=CARTESIAN_POINT('Ctrl Pts',(0.584726479537104,0.851884977081971,
2.03102410122914));
#27726=CARTESIAN_POINT('Ctrl Pts',(0.468017266318098,0.931032088917713,
2.02317355019146));
#27727=CARTESIAN_POINT('Ctrl Pts',(0.469697842938816,1.07206544198931,2.01532299915378));
#27728=CARTESIAN_POINT('Ctrl Pts',(0.588188246262365,1.1484015292732,2.0074724481161));
#27729=CARTESIAN_POINT('Ctrl Pts',(0.717366805638866,1.09178084131602,1.99962189707843));
#27730=CARTESIAN_POINT('Ctrl Pts',(0.741097987339953,0.952575306856465,
1.99177134604075));
#27731=CARTESIAN_POINT('Ctrl Pts',(0.672829925654733,0.888579693265875,
1.98653764534896));
#27732=CARTESIAN_POINT('Ctrl Pts',(0.63265850635311,0.877840168374445,1.98392079500307));
#27733=CARTESIAN_POINT('Ctrl Pts',(0.702845629995662,1.08857942294107,2.40535973499898));
#27734=CARTESIAN_POINT('Ctrl Pts',(0.731974363173428,1.05475934582637,2.40274288465309));
#27735=CARTESIAN_POINT('Ctrl Pts',(0.753809270628911,0.956718355494374,
2.3975091839613));
#27736=CARTESIAN_POINT('Ctrl Pts',(0.648570944161886,0.84762337757721,2.38965863292362));
#27737=CARTESIAN_POINT('Ctrl Pts',(0.499769996315029,0.875540948428836,
2.38180808188594));
#27738=CARTESIAN_POINT('Ctrl Pts',(0.440861440741036,1.01490067966319,2.37395753084827));
#27739=CARTESIAN_POINT('Ctrl Pts',(0.524670026432277,1.1409859567557,2.36610697981059));
#27740=CARTESIAN_POINT('Ctrl Pts',(0.676037410484068,1.14058652601332,2.35825642877291));
#27741=CARTESIAN_POINT('Ctrl Pts',(0.759212082346341,1.01412872620776,2.35040587773524));
#27742=CARTESIAN_POINT('Ctrl Pts',(0.699601856145167,0.87498826132362,2.34255532669755));
#27743=CARTESIAN_POINT('Ctrl Pts',(0.550666173727406,0.847967242717983,
2.33470477565988));
#27744=CARTESIAN_POINT('Ctrl Pts',(0.445974312690722,0.957289789118585,
2.32685422462219));
#27745=CARTESIAN_POINT('Ctrl Pts',(0.479416312569843,1.10491740781463,2.31900367358452));
#27746=CARTESIAN_POINT('Ctrl Pts',(0.62100064898553,1.15845181740151,2.31115312254684));
#27747=CARTESIAN_POINT('Ctrl Pts',(0.743751094493674,1.06988326884919,2.30330257150917));
#27748=CARTESIAN_POINT('Ctrl Pts',(0.737582145876161,0.918641540547371,
2.29545202047149));
#27749=CARTESIAN_POINT('Ctrl Pts',(0.608026255513821,0.840364116095719,
2.28760146943381));
#27750=CARTESIAN_POINT('Ctrl Pts',(0.471272229662835,0.905251894929553,
2.27975091839613));
#27751=CARTESIAN_POINT('Ctrl Pts',(0.449964327931837,1.05511205362507,2.27190036735845));
#27752=CARTESIAN_POINT('Ctrl Pts',(0.563211984134157,1.15554639881562,2.26404981632078));
#27753=CARTESIAN_POINT('Ctrl Pts',(0.709452007382772,1.11648304256461,2.2561992652831));
#27754=CARTESIAN_POINT('Ctrl Pts',(0.757532868423012,0.972954920994454,
2.24834871424542));
#27755=CARTESIAN_POINT('Ctrl Pts',(0.664334507888787,0.853681471028408,
2.24049816320774));
#27756=CARTESIAN_POINT('Ctrl Pts',(0.513439431236242,0.865629955455834,
2.23264761217006));
#27757=CARTESIAN_POINT('Ctrl Pts',(0.440173930500167,0.998084690760198,
2.22479706113238));
#27758=CARTESIAN_POINT('Ctrl Pts',(0.510244248543333,1.13225712068693,2.21694651009471));
#27759=CARTESIAN_POINT('Ctrl Pts',(0.660809658313168,1.14781822067201,2.20909595905703));
#27760=CARTESIAN_POINT('Ctrl Pts',(0.756839520837664,1.03081242611373,2.20124540801935));
#27761=CARTESIAN_POINT('Ctrl Pts',(0.71221197243725,0.886173315337117,2.19339485698167));
#27762=CARTESIAN_POINT('Ctrl Pts',(0.566950059450412,0.843616681399604,
2.18554430594399));
#27763=CARTESIAN_POINT('Ctrl Pts',(0.451328118901268,0.941308325441225,
2.17769375490632));
#27764=CARTESIAN_POINT('Ctrl Pts',(0.469038655723137,1.09163605844015,2.16984320386864));
#27765=CARTESIAN_POINT('Ctrl Pts',(0.604198439657909,1.15978239590126,2.16199265283096));
#27766=CARTESIAN_POINT('Ctrl Pts',(0.735592962824645,1.08463208173108,2.15414210179328));
#27767=CARTESIAN_POINT('Ctrl Pts',(0.745384493923972,0.933581705393252,
2.14629155075561));
#27768=CARTESIAN_POINT('Ctrl Pts',(0.624791753508452,0.842096833207175,
2.13844099971793));
#27769=CARTESIAN_POINT('Ctrl Pts',(0.481965181210706,0.892223277795097,
2.13059044868025));
#27770=CARTESIAN_POINT('Ctrl Pts',(0.444995036483054,1.03900644347833,2.12273989764257));
#27771=CARTESIAN_POINT('Ctrl Pts',(0.547037036003845,1.15080771437549,2.11488934660489));
#27772=CARTESIAN_POINT('Ctrl Pts',(0.696577465165717,1.12736102005574,2.10703879556722));
#27773=CARTESIAN_POINT('Ctrl Pts',(0.759504958213481,0.989693977794033,
2.09918824452954));
#27774=CARTESIAN_POINT('Ctrl Pts',(0.679384552498262,0.861269537383356,
2.09133769349186));
#27775=CARTESIAN_POINT('Ctrl Pts',(0.52807031119791,0.857262038810666,2.08348714245418));
#27776=CARTESIAN_POINT('Ctrl Pts',(0.441264092248243,0.981265013290105,
2.07563659141651));
#27777=CARTESIAN_POINT('Ctrl Pts',(0.496816466213367,1.12207060588009,2.06778604037882));
#27778=CARTESIAN_POINT('Ctrl Pts',(0.644905387984261,1.15339912591488,2.05993548934115));
#27779=CARTESIAN_POINT('Ctrl Pts',(0.752723855715824,1.04715812177925,2.05208493830347));
#27780=CARTESIAN_POINT('Ctrl Pts',(0.723572469244521,0.89861976073157,2.04423438726579));
#27781=CARTESIAN_POINT('Ctrl Pts',(0.583605173237138,0.84101110496317,2.03638383622811));
#27782=CARTESIAN_POINT('Ctrl Pts',(0.458327747053459,0.92596880613495,2.02853328519044));
#27783=CARTESIAN_POINT('Ctrl Pts',(0.460131703294282,1.07735613016487,2.02068273415276));
#27784=CARTESIAN_POINT('Ctrl Pts',(0.587321085746765,1.15929643527098,2.01283218311508));
#27785=CARTESIAN_POINT('Ctrl Pts',(0.72598329578528,1.09851893655959,2.0049816320774));
#27786=CARTESIAN_POINT('Ctrl Pts',(0.751456703426463,0.949093620540274,
1.99713108103973));
#27787=CARTESIAN_POINT('Ctrl Pts',(0.6781767384384,0.880399765646143,1.99189738034794));
#27788=CARTESIAN_POINT('Ctrl Pts',(0.635056132297315,0.86887179797568,1.98928053000205));
#27789=CARTESIAN_POINT('Ctrl Pts',(0.709879644719089,1.09463771598849,2.41071946999795));
#27790=CARTESIAN_POINT('Ctrl Pts',(0.741000605841355,1.05850455157604,2.40810261965206));
#27791=CARTESIAN_POINT('Ctrl Pts',(0.764328887984058,0.953758154611561,
2.40286891896028));
#27792=CARTESIAN_POINT('Ctrl Pts',(0.651892900927377,0.837201744634001,
2.3950183679226));
#27793=CARTESIAN_POINT('Ctrl Pts',(0.492914874501113,0.867028707303451,
2.38716781688492));
#27794=CARTESIAN_POINT('Ctrl Pts',(0.429977332500953,1.01591979540145,2.37931726584724));
#27795=CARTESIAN_POINT('Ctrl Pts',(0.519517915027903,1.15062853754068,2.37146671480957));
#27796=CARTESIAN_POINT('Ctrl Pts',(0.681237906264966,1.15020178816821,2.36361616377189));
#27797=CARTESIAN_POINT('Ctrl Pts',(0.770101219117818,1.01509504503115,2.35576561273421));
#27798=CARTESIAN_POINT('Ctrl Pts',(0.706414016493014,0.866438219766308,
2.34791506169653));
#27799=CARTESIAN_POINT('Ctrl Pts',(0.547292040471776,0.837569128056136,
2.34006451065885));
#27800=CARTESIAN_POINT('Ctrl Pts',(0.435439893752698,0.954368670815423,
2.33221395962117));
#27801=CARTESIAN_POINT('Ctrl Pts',(0.471169122749288,1.11209311952297,2.3243634085835));
#27802=CARTESIAN_POINT('Ctrl Pts',(0.622436965474348,1.16928895668105,2.31651285754582));
#27803=CARTESIAN_POINT('Ctrl Pts',(0.753582793859216,1.07466285882328,2.30866230650814));
#27804=CARTESIAN_POINT('Ctrl Pts',(0.746991926727465,0.913077117424199,
2.30081175547046));
#27805=CARTESIAN_POINT('Ctrl Pts',(0.608575202508074,0.829445993878789,
2.29296120443279));
#27806=CARTESIAN_POINT('Ctrl Pts',(0.462468034171945,0.898771701594062,
2.28511065339511));
#27807=CARTESIAN_POINT('Ctrl Pts',(0.439702801735622,1.05888138244004,2.27726010235743));
#27808=CARTESIAN_POINT('Ctrl Pts',(0.560695907901683,1.16618482515898,2.26940955131976));
#27809=CARTESIAN_POINT('Ctrl Pts',(0.716937858084172,1.12444977325082,2.26155900028207));
#27810=CARTESIAN_POINT('Ctrl Pts',(0.768307157189173,0.9711052023051,2.2537084492444));
#27811=CARTESIAN_POINT('Ctrl Pts',(0.668734596407212,0.843674174781211,
2.24585789820672));
#27812=CARTESIAN_POINT('Ctrl Pts',(0.507519215518976,0.856439862772741,
2.23800734716904));
#27813=CARTESIAN_POINT('Ctrl Pts',(0.429242800746802,0.997953695273144,
2.23015679613136));
#27814=CARTESIAN_POINT('Ctrl Pts',(0.504105501789727,1.14130270224668,2.22230624509369));
#27815=CARTESIAN_POINT('Ctrl Pts',(0.664968668588271,1.15792808669784,2.214455694056));
#27816=CARTESIAN_POINT('Ctrl Pts',(0.767566388851732,1.03291980840074,2.20660514301833));
#27817=CARTESIAN_POINT('Ctrl Pts',(0.71988658793916,0.878388263353175,2.19875459198065));
#27818=CARTESIAN_POINT('Ctrl Pts',(0.564689644803295,0.832921014840122,
2.19090404094297));
#27819=CARTESIAN_POINT('Ctrl Pts',(0.441159867701366,0.937294172355611,
2.1830534899053));
#27820=CARTESIAN_POINT('Ctrl Pts',(0.460081697378071,1.09790340673965,2.17520293886761));
#27821=CARTESIAN_POINT('Ctrl Pts',(0.604485587360446,1.17071053864647,2.16735238782994));
#27822=CARTESIAN_POINT('Ctrl Pts',(0.744866695670093,1.09042040068052,2.15950183679226));
#27823=CARTESIAN_POINT('Ctrl Pts',(0.755327907862536,0.929039098554358,
2.15165128575458));
#27824=CARTESIAN_POINT('Ctrl Pts',(0.626487358457396,0.831297218287773,
2.1438007347169));
#27825=CARTESIAN_POINT('Ctrl Pts',(0.473892318481626,0.884852006396751,
2.13595018367923));
#27826=CARTESIAN_POINT('Ctrl Pts',(0.434393641016582,1.04167424664844,2.12809963264155));
#27827=CARTESIAN_POINT('Ctrl Pts',(0.54341469183073,1.1611220435635,2.12024908160387));
#27828=CARTESIAN_POINT('Ctrl Pts',(0.703182775590238,1.1360717381514,2.11239853056619));
#27829=CARTESIAN_POINT('Ctrl Pts',(0.770414125910549,0.988989108642668,
2.10454797952851));
#27830=CARTESIAN_POINT('Ctrl Pts',(0.684813972407585,0.851781218660681,
2.09669742849084));
#27831=CARTESIAN_POINT('Ctrl Pts',(0.523150758562502,0.84749963159278,2.08884687745316));
#27832=CARTESIAN_POINT('Ctrl Pts',(0.430407522918953,0.979983654302211,
2.08099632641548));
#27833=CARTESIAN_POINT('Ctrl Pts',(0.489759340928599,1.13041949186674,2.0731457753778));
#27834=CARTESIAN_POINT('Ctrl Pts',(0.647976643031809,1.16389069186952,2.06529522434013));
#27835=CARTESIAN_POINT('Ctrl Pts',(0.763169237301496,1.05038345009838,2.05744467330245));
#27836=CARTESIAN_POINT('Ctrl Pts',(0.732024073538381,0.89168596980911,2.04959412226477));
#27837=CARTESIAN_POINT('Ctrl Pts',(0.582483866937173,0.830137232844369,
2.04174357122709));
#27838=CARTESIAN_POINT('Ctrl Pts',(0.448638227788819,0.920905523352185,
2.03389302018941));
#27839=CARTESIAN_POINT('Ctrl Pts',(0.450565563649749,1.08264681834044,2.02604246915174));
#27840=CARTESIAN_POINT('Ctrl Pts',(0.586453925231163,1.17019134126876,2.01819191811406));
#27841=CARTESIAN_POINT('Ctrl Pts',(0.734599785931696,1.10525703180317,2.01034136707638));
#27842=CARTESIAN_POINT('Ctrl Pts',(0.761815419512973,0.945611934224082,
2.0024908160387));
#27843=CARTESIAN_POINT('Ctrl Pts',(0.683523551222068,0.872219838026411,
1.99725711534692));
#27844=CARTESIAN_POINT('Ctrl Pts',(0.63745375824152,0.859903427576914,1.99464026500102));
#27845=CARTESIAN_POINT('Ctrl Pts',(0.716913659442515,1.10069600903591,2.41607920499693));
#27846=CARTESIAN_POINT('Ctrl Pts',(0.750026848509282,1.0622497573257,2.41346235465104));
#27847=CARTESIAN_POINT('Ctrl Pts',(0.774848505339203,0.950797953728747,
2.40822865395925));
#27848=CARTESIAN_POINT('Ctrl Pts',(0.65521485769287,0.826780111690792,2.40037810292158));
#27849=CARTESIAN_POINT('Ctrl Pts',(0.486059752687198,0.858516466178065,
2.3925275518839));
#27850=CARTESIAN_POINT('Ctrl Pts',(0.419093224260869,1.01693891113971,2.38467700084622));
#27851=CARTESIAN_POINT('Ctrl Pts',(0.514365803623529,1.16027111832567,2.37682644980854));
#27852=CARTESIAN_POINT('Ctrl Pts',(0.686438402045863,1.1598170503231,2.36897589877086));
#27853=CARTESIAN_POINT('Ctrl Pts',(0.780990355889297,1.01606136385454,2.36112534773319));
#27854=CARTESIAN_POINT('Ctrl Pts',(0.713226176840859,0.857888178208998,
2.35327479669551));
#27855=CARTESIAN_POINT('Ctrl Pts',(0.54391790721615,0.827171013394288,2.34542424565783));
#27856=CARTESIAN_POINT('Ctrl Pts',(0.424905474814674,0.951447552512262,
2.33757369462016));
#27857=CARTESIAN_POINT('Ctrl Pts',(0.462921932928734,1.11926883123131,2.32972314358247));
#27858=CARTESIAN_POINT('Ctrl Pts',(0.623873281963166,1.1801260959606,2.3218725925448));
#27859=CARTESIAN_POINT('Ctrl Pts',(0.76341449322476,1.07944244879737,2.31402204150712));
#27860=CARTESIAN_POINT('Ctrl Pts',(0.756401707578768,0.907512694301026,
2.30617149046944));
#27861=CARTESIAN_POINT('Ctrl Pts',(0.609124149502328,0.818527871661859,
2.29832093943176));
#27862=CARTESIAN_POINT('Ctrl Pts',(0.453663838681055,0.892291508258571,
2.29047038839408));
#27863=CARTESIAN_POINT('Ctrl Pts',(0.429441275539409,1.06265071125502,2.28261983735641));
#27864=CARTESIAN_POINT('Ctrl Pts',(0.558179831669208,1.17682325150234,2.27476928631873));
#27865=CARTESIAN_POINT('Ctrl Pts',(0.724423708785572,1.13241650393702,2.26691873528105));
#27866=CARTESIAN_POINT('Ctrl Pts',(0.779081445955335,0.969255483615749,
2.25906818424337));
#27867=CARTESIAN_POINT('Ctrl Pts',(0.673134684925636,0.833666878534013,
2.25121763320569));
#27868=CARTESIAN_POINT('Ctrl Pts',(0.50159899980171,0.84724977008965,2.24336708216802));
#27869=CARTESIAN_POINT('Ctrl Pts',(0.418311670993437,0.997822699786089,
2.23551653113034));
#27870=CARTESIAN_POINT('Ctrl Pts',(0.497966755036121,1.15034828380644,2.22766598009266));
#27871=CARTESIAN_POINT('Ctrl Pts',(0.669127678863374,1.16803795272366,2.21981542905498));
#27872=CARTESIAN_POINT('Ctrl Pts',(0.778293256865801,1.03502719068774,2.21196487801731));
#27873=CARTESIAN_POINT('Ctrl Pts',(0.727561203441069,0.870603211369231,
2.20411432697963));
#27874=CARTESIAN_POINT('Ctrl Pts',(0.562429230156179,0.822225348280642,
2.19626377594195));
#27875=CARTESIAN_POINT('Ctrl Pts',(0.430991616501465,0.933280019269996,
2.18841322490427));
#27876=CARTESIAN_POINT('Ctrl Pts',(0.451124739033006,1.10417075503916,2.18056267386659));
#27877=CARTESIAN_POINT('Ctrl Pts',(0.604772735062981,1.18163868139168,2.17271212282892));
#27878=CARTESIAN_POINT('Ctrl Pts',(0.754140428515542,1.09620871962996,2.16486157179123));
#27879=CARTESIAN_POINT('Ctrl Pts',(0.765271321801097,0.924496491715462,
2.15701102075356));
#27880=CARTESIAN_POINT('Ctrl Pts',(0.628182963406343,0.820497603368372,
2.14916046971588));
#27881=CARTESIAN_POINT('Ctrl Pts',(0.465819455752544,0.877480734998406,
2.1413099186782));
#27882=CARTESIAN_POINT('Ctrl Pts',(0.423792245550112,1.04434204981856,2.13345936764053));
#27883=CARTESIAN_POINT('Ctrl Pts',(0.539792347657613,1.17143637275151,2.12560881660284));
#27884=CARTESIAN_POINT('Ctrl Pts',(0.70978808601476,1.14478245624706,2.11775826556517));
#27885=CARTESIAN_POINT('Ctrl Pts',(0.781323293607615,0.988284239491303,
2.10990771452749));
#27886=CARTESIAN_POINT('Ctrl Pts',(0.690243392316909,0.842292899938004,
2.10205716348982));
#27887=CARTESIAN_POINT('Ctrl Pts',(0.518231205927094,0.837737224374896,
2.09420661245213));
#27888=CARTESIAN_POINT('Ctrl Pts',(0.419550953589664,0.978702295314315,
2.08635606141446));
#27889=CARTESIAN_POINT('Ctrl Pts',(0.482702215643831,1.13876837785338,2.07850551037678));
#27890=CARTESIAN_POINT('Ctrl Pts',(0.651047898079357,1.17438225782416,2.0706549593391));
#27891=CARTESIAN_POINT('Ctrl Pts',(0.773614618887169,1.05360877841752,2.06280440830142));
#27892=CARTESIAN_POINT('Ctrl Pts',(0.740475677832241,0.884752178886651,
2.05495385726374));
#27893=CARTESIAN_POINT('Ctrl Pts',(0.581362560637208,0.819263360725568,
2.04710330622607));
#27894=CARTESIAN_POINT('Ctrl Pts',(0.438948708524181,0.915842240569421,
2.03925275518839));
#27895=CARTESIAN_POINT('Ctrl Pts',(0.440999424005214,1.08793750651601,2.03140220415071));
#27896=CARTESIAN_POINT('Ctrl Pts',(0.585586764715563,1.18108624726655,2.02355165311303));
#27897=CARTESIAN_POINT('Ctrl Pts',(0.74321627607811,1.11199512704675,2.01570110207536));
#27898=CARTESIAN_POINT('Ctrl Pts',(0.772174135599484,0.94213024790789,2.00785055103768));
#27899=CARTESIAN_POINT('Ctrl Pts',(0.688870364005735,0.864039910406678,
2.00261685034589));
#27900=CARTESIAN_POINT('Ctrl Pts',(0.639851384185725,0.850935057178149,
2.));
#27901=CARTESIAN_POINT('Ctrl Pts',(0.695811615272236,1.08252112989365,2.4));
#27902=CARTESIAN_POINT('Ctrl Pts',(0.702493035444011,1.07628157141353,2.4));
#27903=CARTESIAN_POINT('Ctrl Pts',(0.708395708847424,1.0693103556765,2.4));
#27904=CARTESIAN_POINT('Ctrl Pts',(0.713512656958279,1.06178684479855,2.4));
#27905=CARTESIAN_POINT('Ctrl Pts',(0.717502347100726,1.05592075498562,2.4));
#27906=CARTESIAN_POINT('Ctrl Pts',(0.721014082031974,1.04971755619462,2.4));
#27907=CARTESIAN_POINT('Ctrl Pts',(0.724031956062882,1.04324616442023,2.4));
#27908=CARTESIAN_POINT('Ctrl Pts',(0.725329175480596,1.04046446611758,2.4));
#27909=CARTESIAN_POINT('Ctrl Pts',(0.726532629865294,1.03763770614082,2.4));
#27910=CARTESIAN_POINT('Ctrl Pts',(0.727638786465014,1.03477907962968,2.4));
#27911=CARTESIAN_POINT('Ctrl Pts',(0.731192959070153,1.02559407631572,2.4));
#27912=CARTESIAN_POINT('Ctrl Pts',(0.733756217444906,1.01606058770234,2.4));
#27913=CARTESIAN_POINT('Ctrl Pts',(0.735294617481607,1.0063604023791,2.4));
#27914=CARTESIAN_POINT('Ctrl Pts',(0.736007696124321,1.00186417589745,2.4));
#27915=CARTESIAN_POINT('Ctrl Pts',(0.736499990230692,0.997331676100057,
2.4));
#27916=CARTESIAN_POINT('Ctrl Pts',(0.736764649954775,0.992779471200463,
2.4));
#27917=CARTESIAN_POINT('Ctrl Pts',(0.736959071387571,0.989435380209583,
2.4));
#27918=CARTESIAN_POINT('Ctrl Pts',(0.737029983554064,0.98608811988667,2.4));
#27919=CARTESIAN_POINT('Ctrl Pts',(0.736976127631269,0.982751397582665,
2.4));
#27920=CARTESIAN_POINT('Ctrl Pts',(0.736862856230108,0.975733502594741,
2.4));
#27921=CARTESIAN_POINT('Ctrl Pts',(0.736199022212823,0.968753098529686,
2.4));
#27922=CARTESIAN_POINT('Ctrl Pts',(0.73496858294117,0.96187154470407,2.4));
#27923=CARTESIAN_POINT('Ctrl Pts',(0.733610269619415,0.954274821768571,
2.4));
#27924=CARTESIAN_POINT('Ctrl Pts',(0.731561915556015,0.946798108708432,
2.4));
#27925=CARTESIAN_POINT('Ctrl Pts',(0.728883391181877,0.939498503415491,
2.4));
#27926=CARTESIAN_POINT('Ctrl Pts',(0.727748787370213,0.936406442701396,
2.4));
#27927=CARTESIAN_POINT('Ctrl Pts',(0.726503663184753,0.933354104764928,
2.4));
#27928=CARTESIAN_POINT('Ctrl Pts',(0.725155437375267,0.93034965316141,2.4));
#27929=CARTESIAN_POINT('Ctrl Pts',(0.721333520454809,0.921832708641144,
2.4));
#27930=CARTESIAN_POINT('Ctrl Pts',(0.716681958573065,0.913689799617633,
2.4));
#27931=CARTESIAN_POINT('Ctrl Pts',(0.711310080831161,0.906016236422445,
2.4));
#27932=CARTESIAN_POINT('Ctrl Pts',(0.708434311712215,0.901908288116612,
2.4));
#27933=CARTESIAN_POINT('Ctrl Pts',(0.705351471044678,0.897934909331024,
2.4));
#27934=CARTESIAN_POINT('Ctrl Pts',(0.702074477330367,0.894112050103086,
2.4));
#27935=CARTESIAN_POINT('Ctrl Pts',(0.699663413790917,0.891299363444374,
2.4));
#27936=CARTESIAN_POINT('Ctrl Pts',(0.697146509627061,0.888567971784173,
2.4));
#27937=CARTESIAN_POINT('Ctrl Pts',(0.694540211514707,0.885935552211034,
2.4));
#27938=CARTESIAN_POINT('Ctrl Pts',(0.689966981858787,0.881316487645227,
2.4));
#27939=CARTESIAN_POINT('Ctrl Pts',(0.685111586013864,0.876992966093948,
2.4));
#27940=CARTESIAN_POINT('Ctrl Pts',(0.680004164916354,0.87299757664439,2.4));
#27941=CARTESIAN_POINT('Ctrl Pts',(0.67522858856925,0.869261779852135,2.4));
#27942=CARTESIAN_POINT('Ctrl Pts',(0.670227032530533,0.865810208752244,
2.4));
#27943=CARTESIAN_POINT('Ctrl Pts',(0.665049792940119,0.862688960723077,
2.4));
#27944=CARTESIAN_POINT('Ctrl Pts',(0.659173917535639,0.859146519967616,
2.4));
#27945=CARTESIAN_POINT('Ctrl Pts',(0.653067316624201,0.856024693283448,
2.4));
#27946=CARTESIAN_POINT('Ctrl Pts',(0.646761964313973,0.85336416176701,2.4));
#27947=CARTESIAN_POINT('Ctrl Pts',(0.644516614709207,0.852416740735641,
2.4));
#27948=CARTESIAN_POINT('Ctrl Pts',(0.642246009555221,0.851527876023459,
2.4));
#27949=CARTESIAN_POINT('Ctrl Pts',(0.63995226235153,0.850696991672974,2.4));
#27950=CARTESIAN_POINT('Ctrl Pts',(0.473597863174539,0.999893075682974,
2.31934196736194));
#27951=CARTESIAN_POINT('Ctrl Pts',(0.473502307398787,0.988483568548598,
2.32005947478237));
#27952=CARTESIAN_POINT('Ctrl Pts',(0.474923175284874,0.977097443610316,
2.3207769822028));
#27953=CARTESIAN_POINT('Ctrl Pts',(0.477956455981403,0.966158447195516,
2.32149448962322));
#27954=CARTESIAN_POINT('Ctrl Pts',(0.489019256746842,0.926262390741107,
2.32411133996911));
#27955=CARTESIAN_POINT('Ctrl Pts',(0.521529781864938,0.892313874060468,
2.32672819031501));
#27956=CARTESIAN_POINT('Ctrl Pts',(0.5609099425597,0.879535106636999,2.3293450406609));
#27957=CARTESIAN_POINT('Ctrl Pts',(0.600290103254463,0.86675633921353,2.33196189100679));
#27958=CARTESIAN_POINT('Ctrl Pts',(0.646539899525892,0.875147321047232,
2.33457874135269));
#27959=CARTESIAN_POINT('Ctrl Pts',(0.678920339291197,0.90094682938132,2.33719559169858));
#27960=CARTESIAN_POINT('Ctrl Pts',(0.711300779056502,0.926746337715409,
2.33981244204447));
#27961=CARTESIAN_POINT('Ctrl Pts',(0.729811862315683,0.969954372549885,
2.34242929239036));
#27962=CARTESIAN_POINT('Ctrl Pts',(0.726153065466658,1.01119319937947,2.34504614273626));
#27963=CARTESIAN_POINT('Ctrl Pts',(0.722494268617633,1.05243202620905,2.34766299308215));
#27964=CARTESIAN_POINT('Ctrl Pts',(0.696665591660402,1.09170164503374,2.35027984342804));
#27965=CARTESIAN_POINT('Ctrl Pts',(0.6602487903707,1.11139847313147,2.35289669377393));
#27966=CARTESIAN_POINT('Ctrl Pts',(0.623831989080998,1.13109530122919,2.35551354411983));
#27967=CARTESIAN_POINT('Ctrl Pts',(0.576827063458825,1.13121933859995,2.35813039446572));
#27968=CARTESIAN_POINT('Ctrl Pts',(0.540311835838483,1.11170438861103,2.36074724481161));
#27969=CARTESIAN_POINT('Ctrl Pts',(0.503796608218141,1.09218943862212,2.3633640951575));
#27970=CARTESIAN_POINT('Ctrl Pts',(0.477771078599631,1.05303550127352,2.3659809455034));
#27971=CARTESIAN_POINT('Ctrl Pts',(0.473904908648346,1.01182047020411,2.36859779584929));
#27972=CARTESIAN_POINT('Ctrl Pts',(0.473538425642629,1.00791360406595,2.36884585302017));
#27973=CARTESIAN_POINT('Ctrl Pts',(0.473371057191087,1.00398821781876,2.36909391019106));
#27974=CARTESIAN_POINT('Ctrl Pts',(0.473395817154925,1.00006080538999,2.36934196736194));
#27975=CARTESIAN_POINT('Ctrl Pts',(0.560148615814278,0.850935057178148,
2.4));
#27976=CARTESIAN_POINT('Ctrl Pts',(0.511129635994267,0.864039910406677,
2.39738314965411));
#27977=CARTESIAN_POINT('Ctrl Pts',(0.427825810157124,0.942129912787787,
2.39214944896232));
#27978=CARTESIAN_POINT('Ctrl Pts',(0.456783771264579,1.11199528864852,2.38429889792464));
#27979=CARTESIAN_POINT('Ctrl Pts',(0.614413228882944,1.18108612135922,2.37644834688697));
#27980=CARTESIAN_POINT('Ctrl Pts',(0.759000551270414,1.08793755388759,2.36859779584929));
#27981=CARTESIAN_POINT('Ctrl Pts',(0.761051274433651,0.91584221771742,2.36074724481161));
#27982=CARTESIAN_POINT('Ctrl Pts',(0.618637433005314,0.819263404514795,
2.35289669377393));
#27983=CARTESIAN_POINT('Ctrl Pts',(0.459524343787705,0.884752183415202,
2.34504614273626));
#27984=CARTESIAN_POINT('Ctrl Pts',(0.426385402694383,1.05360877733288,2.33719559169858));
#27985=CARTESIAN_POINT('Ctrl Pts',(0.548952109888326,1.17438223097154,2.3293450406609));
#27986=CARTESIAN_POINT('Ctrl Pts',(0.717297767916034,1.1387683610531,2.32149448962322));
#27987=CARTESIAN_POINT('Ctrl Pts',(0.780449022522885,0.978702297157564,
2.31364393858554));
#27988=CARTESIAN_POINT('Ctrl Pts',(0.681768782849741,0.837737246759644,
2.30579338754786));
#27989=CARTESIAN_POINT('Ctrl Pts',(0.509756619949943,0.842292920851884,
2.29794283651019));
#27990=CARTESIAN_POINT('Ctrl Pts',(0.418676730713559,0.988284241230286,
2.29009228547251));
#27991=CARTESIAN_POINT('Ctrl Pts',(0.490211928794195,1.14478243668251,2.28224173443483));
#27992=CARTESIAN_POINT('Ctrl Pts',(0.660207644220989,1.17143634973614,2.27439118339715));
#27993=CARTESIAN_POINT('Ctrl Pts',(0.776207730757634,1.04434204382826,2.26654063235948));
#27994=CARTESIAN_POINT('Ctrl Pts',(0.734180526190243,0.87748075149375,2.2586900813218));
#27995=CARTESIAN_POINT('Ctrl Pts',(0.571817040388558,0.820497627508739,
2.25083953028412));
#27996=CARTESIAN_POINT('Ctrl Pts',(0.434728700430063,0.92449650187637,2.24298897924644));
#27997=CARTESIAN_POINT('Ctrl Pts',(0.445859592221225,1.09620870668547,2.23513842820877));
#27998=CARTESIAN_POINT('Ctrl Pts',(0.595227265578502,1.18163865695784,2.22728787717108));
#27999=CARTESIAN_POINT('Ctrl Pts',(0.748875240939872,1.10417074102503,2.21943732613341));
#28000=CARTESIAN_POINT('Ctrl Pts',(0.769008360762544,0.933280028245809,
2.21158677509573));
#28001=CARTESIAN_POINT('Ctrl Pts',(0.637570764789711,0.822225372195567,
2.20373622405805));
#28002=CARTESIAN_POINT('Ctrl Pts',(0.472438813719035,0.870603228776448,
2.19588567302037));
#28003=CARTESIAN_POINT('Ctrl Pts',(0.421706767119107,1.03502718597557,2.1880351219827));
#28004=CARTESIAN_POINT('Ctrl Pts',(0.530872330435983,1.16803793011858,2.18018457094502));
#28005=CARTESIAN_POINT('Ctrl Pts',(0.702033231237909,1.1503482635805,2.17233401990734));
#28006=CARTESIAN_POINT('Ctrl Pts',(0.781688304564893,0.997822700079642,
2.16448346886966));
#28007=CARTESIAN_POINT('Ctrl Pts',(0.698400986961052,0.847249790637147,
2.15663291783198));
#28008=CARTESIAN_POINT('Ctrl Pts',(0.526865324912526,0.833666900912216,
2.14878236679431));
#28009=CARTESIAN_POINT('Ctrl Pts',(0.420918578136115,0.969255487747401,
2.14093181575663));
#28010=CARTESIAN_POINT('Ctrl Pts',(0.475576307951429,1.13241648613165,2.13308126471895));
#28011=CARTESIAN_POINT('Ctrl Pts',(0.641820162707069,1.17682322770038,2.12523071368128));
#28012=CARTESIAN_POINT('Ctrl Pts',(0.770558701511974,1.06265070285456,2.11738016264359));
#28013=CARTESIAN_POINT('Ctrl Pts',(0.746336141641471,0.892291522696776,
2.10952961160592));
#28014=CARTESIAN_POINT('Ctrl Pts',(0.590875851708506,0.818527896169216,
2.10167906056824));
#28015=CARTESIAN_POINT('Ctrl Pts',(0.443598313494032,0.907512706568079,
2.09382850953057));
#28016=CARTESIAN_POINT('Ctrl Pts',(0.436585528693405,1.07944243843108,2.08597795849288));
#28017=CARTESIAN_POINT('Ctrl Pts',(0.57612672137744,1.18012607114374,2.07812740745521));
#28018=CARTESIAN_POINT('Ctrl Pts',(0.737078048375186,1.11926881624917,2.07027685641753));
#28019=CARTESIAN_POINT('Ctrl Pts',(0.775094502137202,0.951447557128672,
2.06242630537985));
#28020=CARTESIAN_POINT('Ctrl Pts',(0.656082084236305,0.827171040068,2.05457575434217));
#28021=CARTESIAN_POINT('Ctrl Pts',(0.48677384037764,0.857888191265152,2.04672520330449));
#28022=CARTESIAN_POINT('Ctrl Pts',(0.419009664523655,1.01606137229499,2.03887465226682));
#28023=CARTESIAN_POINT('Ctrl Pts',(0.513561617374857,1.15981701056446,2.03102410122914));
#28024=CARTESIAN_POINT('Ctrl Pts',(0.685634169421134,1.1602711276025,2.02317355019146));
#28025=CARTESIAN_POINT('Ctrl Pts',(0.780906782004492,1.01693885807272,2.01532299915378));
#28026=CARTESIAN_POINT('Ctrl Pts',(0.713940171081941,0.858516566589665,
2.0074724481161));
#28027=CARTESIAN_POINT('Ctrl Pts',(0.544785272473601,0.826780004858426,
1.99962189707843));
#28028=CARTESIAN_POINT('Ctrl Pts',(0.425151261024703,0.95079820002532,1.99177134604075));
#28029=CARTESIAN_POINT('Ctrl Pts',(0.449973151490716,1.0622497573257,1.98653764534896));
#28030=CARTESIAN_POINT('Ctrl Pts',(0.483086340557483,1.10069600903591,1.98392079500307));
#28031=CARTESIAN_POINT('Ctrl Pts',(0.562546241758482,0.859903427576914,
2.40535973499898));
#28032=CARTESIAN_POINT('Ctrl Pts',(0.516476448777934,0.872219838026409,
2.40274288465309));
#28033=CARTESIAN_POINT('Ctrl Pts',(0.438184529507143,0.945611619266206,
2.3975091839613));
#28034=CARTESIAN_POINT('Ctrl Pts',(0.46540025856266,1.1052571836823,2.38965863292362));
#28035=CARTESIAN_POINT('Ctrl Pts',(0.613546068752483,1.17019122293655,2.38180808188594));
#28036=CARTESIAN_POINT('Ctrl Pts',(0.749434413113403,1.08264686286195,2.37395753084827));
#28037=CARTESIAN_POINT('Ctrl Pts',(0.751361756194339,0.920905501875057,
2.36610697981059));
#28038=CARTESIAN_POINT('Ctrl Pts',(0.617516127087842,0.830137273999053,
2.35825642877291));
#28039=CARTESIAN_POINT('Ctrl Pts',(0.467975946780819,0.891685974065206,
2.35040587773523));
#28040=CARTESIAN_POINT('Ctrl Pts',(0.436830782981619,1.050383449079,2.34255532669756));
#28041=CARTESIAN_POINT('Ctrl Pts',(0.552023364456505,1.16389066663247,2.33470477565987));
#28042=CARTESIAN_POINT('Ctrl Pts',(0.710240643620372,1.13041947607723,2.3268542246222));
#28043=CARTESIAN_POINT('Ctrl Pts',(0.769592454630765,0.979983656034563,
2.31900367358452));
#28044=CARTESIAN_POINT('Ctrl Pts',(0.676849230889565,0.847499652630768,
2.31115312254684));
#28045=CARTESIAN_POINT('Ctrl Pts',(0.515186039121242,0.851781238316293,
2.30330257150916));
#28046=CARTESIAN_POINT('Ctrl Pts',(0.429585896947362,0.988989110277028,
2.29545202047149));
#28047=CARTESIAN_POINT('Ctrl Pts',(0.496817238327747,1.13607171976393,2.28760146943381));
#28048=CARTESIAN_POINT('Ctrl Pts',(0.65658530053649,1.16112202193283,2.27975091839613));
#28049=CARTESIAN_POINT('Ctrl Pts',(0.765606336716589,1.04167424101854,2.27190036735845));
#28050=CARTESIAN_POINT('Ctrl Pts',(0.726107664547559,0.884852021899667,
2.26404981632077));
#28051=CARTESIAN_POINT('Ctrl Pts',(0.573512645109186,0.831297240975754,
2.2561992652831));
#28052=CARTESIAN_POINT('Ctrl Pts',(0.444672113031105,0.929039108103942,
2.24834871424542));
#28053=CARTESIAN_POINT('Ctrl Pts',(0.455133323819063,1.09042038851482,2.24049816320774));
#28054=CARTESIAN_POINT('Ctrl Pts',(0.595514413242444,1.17071051568267,2.23264761217006));
#28055=CARTESIAN_POINT('Ctrl Pts',(0.739918283799722,1.09790339356867,2.22479706113239));
#28056=CARTESIAN_POINT('Ctrl Pts',(0.758840110930535,0.9372941807914,2.21694651009471));
#28057=CARTESIAN_POINT('Ctrl Pts',(0.635310350446671,0.832921037316226,
2.20909595905703));
#28058=CARTESIAN_POINT('Ctrl Pts',(0.480113428188521,0.878388279713101,
2.20124540801935));
#28059=CARTESIAN_POINT('Ctrl Pts',(0.432433633690143,1.03291980397207,2.19339485698167));
#28060=CARTESIAN_POINT('Ctrl Pts',(0.535031340151599,1.15792806545277,2.185544305944));
#28061=CARTESIAN_POINT('Ctrl Pts',(0.695894485310114,1.14130268323763,2.17769375490632));
#28062=CARTESIAN_POINT('Ctrl Pts',(0.770757176282041,0.997953695549035,
2.16984320386864));
#28063=CARTESIAN_POINT('Ctrl Pts',(0.692480772040193,0.856439882084015,
2.16199265283096));
#28064=CARTESIAN_POINT('Ctrl Pts',(0.531265412839046,0.843674195813048,
2.15414210179328));
#28065=CARTESIAN_POINT('Ctrl Pts',(0.431692865452835,0.971105206188175,
2.1462915507556));
#28066=CARTESIAN_POINT('Ctrl Pts',(0.483062157645861,1.12444975651669,2.13844099971793));
#28067=CARTESIAN_POINT('Ctrl Pts',(0.639304086812941,1.16618480278905,2.13059044868025));
#28068=CARTESIAN_POINT('Ctrl Pts',(0.760297176696446,1.05888137454499,2.12273989764257));
#28069=CARTESIAN_POINT('Ctrl Pts',(0.73753194733446,0.898771715163604,2.11488934660489));
#28070=CARTESIAN_POINT('Ctrl Pts',(0.591424798629911,0.829446016911682,
2.10703879556722));
#28071=CARTESIAN_POINT('Ctrl Pts',(0.453008093077508,0.913077128953215,
2.09918824452954));
#28072=CARTESIAN_POINT('Ctrl Pts',(0.44641722674026,1.07466284908066,2.09133769349186));
#28073=CARTESIAN_POINT('Ctrl Pts',(0.577563037665274,1.16928893335727,2.08348714245418));
#28074=CARTESIAN_POINT('Ctrl Pts',(0.728830859679466,1.11209310544222,2.0756365914165));
#28075=CARTESIAN_POINT('Ctrl Pts',(0.76456008458585,0.954368675154091,2.06778604037883));
#28076=CARTESIAN_POINT('Ctrl Pts',(0.652707951494933,0.837569153125047,
2.05993548934115));
#28077=CARTESIAN_POINT('Ctrl Pts',(0.493585999689548,0.866438232036949,
2.05208493830347));
#28078=CARTESIAN_POINT('Ctrl Pts',(0.429898800067004,1.01509505296379,2.04423438726579));
#28079=CARTESIAN_POINT('Ctrl Pts',(0.518762111987321,1.15020175080161,2.03638383622811));
#28080=CARTESIAN_POINT('Ctrl Pts',(0.680482059638507,1.15062854625939,2.02853328519044));
#28081=CARTESIAN_POINT('Ctrl Pts',(0.770022673387457,1.01591974552719,2.02068273415276));
#28082=CARTESIAN_POINT('Ctrl Pts',(0.707085053854394,0.867028801673869,
2.01283218311508));
#28083=CARTESIAN_POINT('Ctrl Pts',(0.548107221407733,0.837201644229118,
2.0049816320774));
#28084=CARTESIAN_POINT('Ctrl Pts',(0.435670892436373,0.953758386089901,
1.99713108103972));
#28085=CARTESIAN_POINT('Ctrl Pts',(0.458999394158644,1.05850455157603,1.99189738034794));
#28086=CARTESIAN_POINT('Ctrl Pts',(0.490120355280909,1.09463771598849,1.98928053000205));
#28087=CARTESIAN_POINT('Ctrl Pts',(0.564943867702687,0.868871797975679,
2.41071946999795));
#28088=CARTESIAN_POINT('Ctrl Pts',(0.521823261561601,0.880399765646142,
2.40810261965206));
#28089=CARTESIAN_POINT('Ctrl Pts',(0.448543248857163,0.949093325744624,
2.40286891896027));
#28090=CARTESIAN_POINT('Ctrl Pts',(0.474016745860739,1.09851907871609,2.3950183679226));
#28091=CARTESIAN_POINT('Ctrl Pts',(0.612678908622024,1.15929632451388,2.38716781688491));
#28092=CARTESIAN_POINT('Ctrl Pts',(0.739868274956389,1.07735617183631,2.37931726584725));
#28093=CARTESIAN_POINT('Ctrl Pts',(0.741672237955028,0.925968786032693,
2.37146671480956));
#28094=CARTESIAN_POINT('Ctrl Pts',(0.616394821170369,0.841011143483312,
2.36361616377189));
#28095=CARTESIAN_POINT('Ctrl Pts',(0.476427549773933,0.898619764715207,
2.35576561273421));
#28096=CARTESIAN_POINT('Ctrl Pts',(0.447276163268855,1.04715812082513,2.34791506169653));
#28097=CARTESIAN_POINT('Ctrl Pts',(0.555094619024684,1.15339910229339,2.34006451065885));
#28098=CARTESIAN_POINT('Ctrl Pts',(0.703183519324712,1.12207059110137,2.33221395962117));
#28099=CARTESIAN_POINT('Ctrl Pts',(0.758735886738644,0.981265014911558,
2.3243634085835));
#28100=CARTESIAN_POINT('Ctrl Pts',(0.67192967892939,0.857262058501895,2.31651285754582));
#28101=CARTESIAN_POINT('Ctrl Pts',(0.52061545829254,0.861269555780702,2.30866230650814));
#28102=CARTESIAN_POINT('Ctrl Pts',(0.440495063181165,0.989693979323769,
2.30081175547046));
#28103=CARTESIAN_POINT('Ctrl Pts',(0.5034225478613,1.12736100284536,2.29296120443278));
#28104=CARTESIAN_POINT('Ctrl Pts',(0.652962956851991,1.15080769412952,2.28511065339511));
#28105=CARTESIAN_POINT('Ctrl Pts',(0.755004942675543,1.03900643820883,2.27726010235743));
#28106=CARTESIAN_POINT('Ctrl Pts',(0.718034802904875,0.892223292305585,
2.26940955131975));
#28107=CARTESIAN_POINT('Ctrl Pts',(0.575208249829814,0.84209685444277,2.26155900028207));
#28108=CARTESIAN_POINT('Ctrl Pts',(0.454615525632148,0.933581714331513,
2.25370844924439));
#28109=CARTESIAN_POINT('Ctrl Pts',(0.4644070554169,1.08463207034418,2.24585789820672));
#28110=CARTESIAN_POINT('Ctrl Pts',(0.595801560906386,1.1597823744075,2.23800734716904));
#28111=CARTESIAN_POINT('Ctrl Pts',(0.730961326659572,1.09163604611232,2.23015679613136));
#28112=CARTESIAN_POINT('Ctrl Pts',(0.748671861098526,0.941308333336992,
2.22230624509368));
#28113=CARTESIAN_POINT('Ctrl Pts',(0.63304993610363,0.843616702436886,2.214455694056));
#28114=CARTESIAN_POINT('Ctrl Pts',(0.487788042658006,0.886173330649751,
2.20660514301833));
#28115=CARTESIAN_POINT('Ctrl Pts',(0.443160500261181,1.03081242196857,2.19875459198065));
#28116=CARTESIAN_POINT('Ctrl Pts',(0.539190349867211,1.14781820078696,2.19090404094297));
#28117=CARTESIAN_POINT('Ctrl Pts',(0.689755739382323,1.13225710289476,2.18305348990529));
#28118=CARTESIAN_POINT('Ctrl Pts',(0.759826047999188,0.998084691018425,
2.17520293886762));
#28119=CARTESIAN_POINT('Ctrl Pts',(0.686560557119336,0.865629973530885,
2.16735238782994));
#28120=CARTESIAN_POINT('Ctrl Pts',(0.535665500765565,0.853681490713878,
2.15950183679226));
#28121=CARTESIAN_POINT('Ctrl Pts',(0.442467152769555,0.972954924628952,
2.15165128575459));
#28122=CARTESIAN_POINT('Ctrl Pts',(0.490548007340293,1.11648302690173,2.1438007347169));
#28123=CARTESIAN_POINT('Ctrl Pts',(0.636788010918814,1.15554637787772,2.13595018367923));
#28124=CARTESIAN_POINT('Ctrl Pts',(0.750035651880915,1.05511204623542,2.12809963264155));
#28125=CARTESIAN_POINT('Ctrl Pts',(0.728727753027451,0.905251907630433,
2.12024908160387));
#28126=CARTESIAN_POINT('Ctrl Pts',(0.591973745551315,0.840364137654146,
2.11239853056619));
#28127=CARTESIAN_POINT('Ctrl Pts',(0.462417872660985,0.918641551338351,
2.10454797952851));
#28128=CARTESIAN_POINT('Ctrl Pts',(0.456248924787112,1.06988325973025,2.09669742849084));
#28129=CARTESIAN_POINT('Ctrl Pts',(0.578999353953109,1.15845179557081,2.08884687745316));
#28130=CARTESIAN_POINT('Ctrl Pts',(0.720583670983745,1.10491739463527,2.08099632641548));
#28131=CARTESIAN_POINT('Ctrl Pts',(0.754025667034497,0.957289793179509,
2.0731457753778));
#28132=CARTESIAN_POINT('Ctrl Pts',(0.649333818753561,0.847967266182092,
2.06529522434013));
#28133=CARTESIAN_POINT('Ctrl Pts',(0.500398159001457,0.874988272808748,
2.05744467330245));
#28134=CARTESIAN_POINT('Ctrl Pts',(0.440787935610353,1.01412873363258,2.04959412226477));
#28135=CARTESIAN_POINT('Ctrl Pts',(0.523962606599787,1.14058649103877,2.04174357122709));
#28136=CARTESIAN_POINT('Ctrl Pts',(0.675329949855879,1.14098596491627,2.03389302018941));
#28137=CARTESIAN_POINT('Ctrl Pts',(0.759138564770422,1.01490063298166,2.02604246915174));
#28138=CARTESIAN_POINT('Ctrl Pts',(0.700229936626846,0.875541036758072,
2.01819191811406));
#28139=CARTESIAN_POINT('Ctrl Pts',(0.551429170341866,0.847623283599809,
2.01034136707638));
#28140=CARTESIAN_POINT('Ctrl Pts',(0.446190523848043,0.956718572154482,
2.0024908160387));
#28141=CARTESIAN_POINT('Ctrl Pts',(0.468025636826571,1.05475934582637,1.99725711534692));
#28142=CARTESIAN_POINT('Ctrl Pts',(0.497154370004336,1.08857942294107,1.99464026500102));
#28143=CARTESIAN_POINT('Ctrl Pts',(0.567341493646892,0.877840168374445,
2.41607920499693));
#28144=CARTESIAN_POINT('Ctrl Pts',(0.527170074345269,0.888579693265874,
2.41346235465104));
#28145=CARTESIAN_POINT('Ctrl Pts',(0.458901968207183,0.952575032223043,
2.40822865395925));
#28146=CARTESIAN_POINT('Ctrl Pts',(0.482633233158821,1.09178097374987,2.40037810292158));
#28147=CARTESIAN_POINT('Ctrl Pts',(0.611811748491563,1.14840142609121,2.3925275518839));
#28148=CARTESIAN_POINT('Ctrl Pts',(0.730302136799378,1.07206548081067,2.38467700084622));
#28149=CARTESIAN_POINT('Ctrl Pts',(0.731982719715716,0.931032070190328,
2.37682644980854));
#28150=CARTESIAN_POINT('Ctrl Pts',(0.615273515252898,0.85188501296757,2.36897589877086));
#28151=CARTESIAN_POINT('Ctrl Pts',(0.484879152767046,0.905553555365211,
2.36112534773319));
#28152=CARTESIAN_POINT('Ctrl Pts',(0.457721543556091,1.04393279257125,2.35327479669551));
#28153=CARTESIAN_POINT('Ctrl Pts',(0.558165873592863,1.14290753795432,2.34542424565783));
#28154=CARTESIAN_POINT('Ctrl Pts',(0.69612639502905,1.1137217061255,2.33757369462015));
#28155=CARTESIAN_POINT('Ctrl Pts',(0.747879318846525,0.982546373788555,
2.32972314358248));
#28156=CARTESIAN_POINT('Ctrl Pts',(0.667010126969215,0.86702446437302,2.32187259254479));
#28157=CARTESIAN_POINT('Ctrl Pts',(0.526044877463838,0.870757873245112,
2.31402204150712));
#28158=CARTESIAN_POINT('Ctrl Pts',(0.451404229414968,0.99039884837051,2.30617149046944));
#28159=CARTESIAN_POINT('Ctrl Pts',(0.510027857394853,1.11865028592679,2.29832093943177));
#28160=CARTESIAN_POINT('Ctrl Pts',(0.649340613167492,1.14049336632621,2.29047038839408));
#28161=CARTESIAN_POINT('Ctrl Pts',(0.744403548634497,1.03633863539911,2.28261983735641));
#28162=CARTESIAN_POINT('Ctrl Pts',(0.709961941262192,0.899594562711502,
2.27476928631873));
#28163=CARTESIAN_POINT('Ctrl Pts',(0.576903854550442,0.852896467909786,
2.26691873528105));
#28164=CARTESIAN_POINT('Ctrl Pts',(0.464558938233191,0.938124320559086,
2.25906818424337));
#28165=CARTESIAN_POINT('Ctrl Pts',(0.473680787014737,1.07884375217354,2.2512176332057));
#28166=CARTESIAN_POINT('Ctrl Pts',(0.596088708570328,1.14885423313233,2.24336708216801));
#28167=CARTESIAN_POINT('Ctrl Pts',(0.722004369519422,1.08536869865596,2.23551653113034));
#28168=CARTESIAN_POINT('Ctrl Pts',(0.738503611266517,0.945322485882583,
2.22766598009266));
#28169=CARTESIAN_POINT('Ctrl Pts',(0.63078952176059,0.854312367557547,2.21981542905498));
#28170=CARTESIAN_POINT('Ctrl Pts',(0.495462657127491,0.893958381586401,
2.21196487801731));
#28171=CARTESIAN_POINT('Ctrl Pts',(0.453887366832218,1.02870503996507,2.20411432697962));
#28172=CARTESIAN_POINT('Ctrl Pts',(0.543349359582825,1.13770833612116,2.19626377594195));
#28173=CARTESIAN_POINT('Ctrl Pts',(0.683616993454529,1.12321152255188,2.18841322490427));
#28174=CARTESIAN_POINT('Ctrl Pts',(0.748894919716335,0.998215686487819,
2.18056267386659));
#28175=CARTESIAN_POINT('Ctrl Pts',(0.680640342198477,0.874820064977753,
2.17271212282892));
#28176=CARTESIAN_POINT('Ctrl Pts',(0.540065588692086,0.863688785614711,
2.16486157179124));
#28177=CARTESIAN_POINT('Ctrl Pts',(0.453241440086272,0.974804643069725,
2.15701102075356));
#28178=CARTESIAN_POINT('Ctrl Pts',(0.498033857034726,1.10851629728676,2.14916046971588));
#28179=CARTESIAN_POINT('Ctrl Pts',(0.634271935024686,1.14490795296639,2.1413099186782));
#28180=CARTESIAN_POINT('Ctrl Pts',(0.739774127065386,1.05134271792586,2.13345936764053));
#28181=CARTESIAN_POINT('Ctrl Pts',(0.719923558720441,0.911732100097261,
2.12560881660285));
#28182=CARTESIAN_POINT('Ctrl Pts',(0.592522692472719,0.851282258396612,
2.11775826556517));
#28183=CARTESIAN_POINT('Ctrl Pts',(0.471827652244461,0.924205973723485,
2.10990771452749));
#28184=CARTESIAN_POINT('Ctrl Pts',(0.466080622833967,1.06510367037984,2.10205716348981));
#28185=CARTESIAN_POINT('Ctrl Pts',(0.580435670240942,1.14761465778435,2.09420661245214));
#28186=CARTESIAN_POINT('Ctrl Pts',(0.712336482288025,1.09774168382831,2.08635606141445));
#28187=CARTESIAN_POINT('Ctrl Pts',(0.743491249483144,0.960210911204929,
2.07850551037678));
#28188=CARTESIAN_POINT('Ctrl Pts',(0.645959686012189,0.858365379239137,
2.0706549593391));
#28189=CARTESIAN_POINT('Ctrl Pts',(0.507210318313367,0.883538313580547,
2.06280440830142));
#28190=CARTESIAN_POINT('Ctrl Pts',(0.451677071153702,1.01316241430137,2.05495385726375));
#28191=CARTESIAN_POINT('Ctrl Pts',(0.529163101212253,1.13097123127593,2.04710330622607));
#28192=CARTESIAN_POINT('Ctrl Pts',(0.670177840073251,1.13134338357315,2.03925275518839));
#28193=CARTESIAN_POINT('Ctrl Pts',(0.748254456153389,1.01388152043613,2.03140220415071));
#28194=CARTESIAN_POINT('Ctrl Pts',(0.693374819399297,0.884053271842277,
2.02355165311304));
#28195=CARTESIAN_POINT('Ctrl Pts',(0.554751119276,0.858044922970499,2.01570110207535));
#28196=CARTESIAN_POINT('Ctrl Pts',(0.456710155259713,0.959678758219065,
2.00785055103768));
#28197=CARTESIAN_POINT('Ctrl Pts',(0.477051879494498,1.0510141400767,2.00261685034589));
#28198=CARTESIAN_POINT('Ctrl Pts',(0.504188384727762,1.08252112989365,2.));
#28199=CARTESIAN_POINT('Ctrl Pts',(0.473630671680838,1.00010094048498,2.35565803263806));
#28200=CARTESIAN_POINT('Ctrl Pts',(0.473532439388447,1.01274184176985,2.35486362065721));
#28201=CARTESIAN_POINT('Ctrl Pts',(0.475280523076927,1.02535622997532,2.35406920867636));
#28202=CARTESIAN_POINT('Ctrl Pts',(0.478988533430712,1.03736537726742,2.35327479669551));
#28203=CARTESIAN_POINT('Ctrl Pts',(0.491202986901682,1.0769243743656,2.35065794634962));
#28204=CARTESIAN_POINT('Ctrl Pts',(0.524684430247273,1.10991595615996,2.34804109600373));
#28205=CARTESIAN_POINT('Ctrl Pts',(0.564418572159433,1.12154744175234,2.34542424565783));
#28206=CARTESIAN_POINT('Ctrl Pts',(0.604152714071593,1.13317892734471,2.34280739531194));
#28207=CARTESIAN_POINT('Ctrl Pts',(0.650139554550321,1.12345031673511,2.34019054496604));
#28208=CARTESIAN_POINT('Ctrl Pts',(0.681758462092598,1.09672345604081,2.33757369462015));
#28209=CARTESIAN_POINT('Ctrl Pts',(0.713377369634875,1.06999659534652,2.33495684427426));
#28210=CARTESIAN_POINT('Ctrl Pts',(0.7306283442407,1.02627148456754,2.33233999392837));
#28211=CARTESIAN_POINT('Ctrl Pts',(0.725775632897394,0.98515527760879,2.32972314358247));
#28212=CARTESIAN_POINT('Ctrl Pts',(0.720922921554088,0.944039070650043,
2.32710629323658));
#28213=CARTESIAN_POINT('Ctrl Pts',(0.693966524261651,0.905531767511531,
2.32448944289069));
#28214=CARTESIAN_POINT('Ctrl Pts',(0.656994117364537,0.886900350754291,
2.32187259254479));
#28215=CARTESIAN_POINT('Ctrl Pts',(0.620021710467422,0.86826893399705,2.3192557421989));
#28216=CARTESIAN_POINT('Ctrl Pts',(0.57303329396563,0.869513403621081,2.31663889185301));
#28217=CARTESIAN_POINT('Ctrl Pts',(0.537098977706589,0.890075800953996,
2.31402204150712));
#28218=CARTESIAN_POINT('Ctrl Pts',(0.501164661447548,0.910638198286911,
2.31140519116123));
#28219=CARTESIAN_POINT('Ctrl Pts',(0.476284445431258,0.95051852332871,2.30878834081533));
#28220=CARTESIAN_POINT('Ctrl Pts',(0.473614942086427,0.991833925442323,
2.30617149046944));
#28221=CARTESIAN_POINT('Ctrl Pts',(0.4734403457566,0.99453612006154,2.30600033785898));
#28222=CARTESIAN_POINT('Ctrl Pts',(0.4733607599644,0.997244453495218,2.30582918524852));
#28223=CARTESIAN_POINT('Ctrl Pts',(0.473373733146151,0.999953562449677,
2.30565803263806));
#28224=CARTESIAN_POINT('Ctrl Pts',(0.560148615814278,0.850935057178148,
2.4));
#28225=CARTESIAN_POINT('Ctrl Pts',(0.550119440006157,0.854599676739477,
2.4));
#28226=CARTESIAN_POINT('Ctrl Pts',(0.540564996368976,0.859362632124605,
2.4));
#28227=CARTESIAN_POINT('Ctrl Pts',(0.531596820053353,0.865074091447543,
2.4));
#28228=CARTESIAN_POINT('Ctrl Pts',(0.527131647122934,0.867917774785653,
2.4));
#28229=CARTESIAN_POINT('Ctrl Pts',(0.522812231247153,0.870997309268362,
2.4));
#28230=CARTESIAN_POINT('Ctrl Pts',(0.518655594653448,0.874297505825464,
2.4));
#28231=CARTESIAN_POINT('Ctrl Pts',(0.515850253684945,0.876524829864272,
2.4));
#28232=CARTESIAN_POINT('Ctrl Pts',(0.513119107067925,0.878852705294647,
2.4));
#28233=CARTESIAN_POINT('Ctrl Pts',(0.510468112479774,0.881276804671575,
2.4));
#28234=CARTESIAN_POINT('Ctrl Pts',(0.508096911905004,0.883445057244236,
2.4));
#28235=CARTESIAN_POINT('Ctrl Pts',(0.505796540173907,0.885684216423859,
2.4));
#28236=CARTESIAN_POINT('Ctrl Pts',(0.503571411911721,0.887989047157772,
2.4));
#28237=CARTESIAN_POINT('Ctrl Pts',(0.496344342241171,0.895474985193744,
2.4));
#28238=CARTESIAN_POINT('Ctrl Pts',(0.489902891057215,0.903656331605307,
2.4));
#28239=CARTESIAN_POINT('Ctrl Pts',(0.484380306519488,0.912413061717332,
2.4));
#28240=CARTESIAN_POINT('Ctrl Pts',(0.482085857904318,0.91605118932619,2.4));
#28241=CARTESIAN_POINT('Ctrl Pts',(0.479950575517979,0.919788877767087,
2.4));
#28242=CARTESIAN_POINT('Ctrl Pts',(0.477986676370491,0.923618156800881,
2.4));
#28243=CARTESIAN_POINT('Ctrl Pts',(0.476502903437523,0.92651126900086,2.4));
#28244=CARTESIAN_POINT('Ctrl Pts',(0.475117212818011,0.929456979534617,
2.4));
#28245=CARTESIAN_POINT('Ctrl Pts',(0.473840374483033,0.932438138949923,
2.4));
#28246=CARTESIAN_POINT('Ctrl Pts',(0.470678069804683,0.939821481153613,
2.4));
#28247=CARTESIAN_POINT('Ctrl Pts',(0.468171071299299,0.947441891244077,
2.4));
#28248=CARTESIAN_POINT('Ctrl Pts',(0.466390209012142,0.955243589562609,
2.4));
#28249=CARTESIAN_POINT('Ctrl Pts',(0.464752055683344,0.962420100718438,
2.4));
#28250=CARTESIAN_POINT('Ctrl Pts',(0.46372877679908,0.9697505149636,2.4));
#28251=CARTESIAN_POINT('Ctrl Pts',(0.463308980593947,0.977159382735458,
2.4));
#28252=CARTESIAN_POINT('Ctrl Pts',(0.463132836556449,0.980268100410063,
2.4));
#28253=CARTESIAN_POINT('Ctrl Pts',(0.463063518093533,0.983387131233213,
2.4));
#28254=CARTESIAN_POINT('Ctrl Pts',(0.463099417336848,0.986501004293148,
2.4));
#28255=CARTESIAN_POINT('Ctrl Pts',(0.463196741723633,0.994942847577307,
2.4));
#28256=CARTESIAN_POINT('Ctrl Pts',(0.464064109534936,1.00336872849097,2.4));
#28257=CARTESIAN_POINT('Ctrl Pts',(0.46567545593174,1.01166502412979,2.4));
#28258=CARTESIAN_POINT('Ctrl Pts',(0.466871287371351,1.0178219691398,2.4));
#28259=CARTESIAN_POINT('Ctrl Pts',(0.468477485851221,1.02390757093803,2.4));
#28260=CARTESIAN_POINT('Ctrl Pts',(0.47049181446679,1.02987017308613,2.4));
#28261=CARTESIAN_POINT('Ctrl Pts',(0.471677008778134,1.0333784597143,2.4));
#28262=CARTESIAN_POINT('Ctrl Pts',(0.473001300296321,1.03683670710464,2.4));
#28263=CARTESIAN_POINT('Ctrl Pts',(0.474460926720988,1.04022911545352,2.4));
#28264=CARTESIAN_POINT('Ctrl Pts',(0.476751356878834,1.04555244631317,2.4));
#28265=CARTESIAN_POINT('Ctrl Pts',(0.479376309757289,1.05071849279536,2.4));
#28266=CARTESIAN_POINT('Ctrl Pts',(0.482333049272134,1.05568492650343,2.4));
#28267=CARTESIAN_POINT('Ctrl Pts',(0.48437450467299,1.05911395799755,2.4));
#28268=CARTESIAN_POINT('Ctrl Pts',(0.486574676429565,1.06244757032586,2.4));
#28269=CARTESIAN_POINT('Ctrl Pts',(0.4889242778747,1.06565919855071,2.4));
#28270=CARTESIAN_POINT('Ctrl Pts',(0.492216707071327,1.07015956117947,2.4));
#28271=CARTESIAN_POINT('Ctrl Pts',(0.495805971455815,1.07442716938164,2.4));
#28272=CARTESIAN_POINT('Ctrl Pts',(0.499690943915119,1.07842077967776,2.4));
#28273=CARTESIAN_POINT('Ctrl Pts',(0.501092720341441,1.07986175482692,2.4));
#28274=CARTESIAN_POINT('Ctrl Pts',(0.502533036573698,1.08126699616446,2.4));
#28275=CARTESIAN_POINT('Ctrl Pts',(0.504010178078511,1.08263575731582,2.4));
#28276=CARTESIAN_POINT('Origin',(-0.6,1.,2.15));
#28277=CARTESIAN_POINT('Origin',(0.6,1.,2.15));
#28278=CARTESIAN_POINT('Origin',(-4.61329551933804E-18,0.,7.7));
#28279=CARTESIAN_POINT('Ctrl Pts',(-0.163512932725147,-0.0319230454628249,
7.7));
#28280=CARTESIAN_POINT('Ctrl Pts',(-0.162868713187189,-0.0402193670799747,
7.7));
#28281=CARTESIAN_POINT('Ctrl Pts',(-0.161555734105899,-0.0484297746987163,
7.7));
#28282=CARTESIAN_POINT('Ctrl Pts',(-0.159632542759909,-0.0565029299462262,
7.7));
#28283=CARTESIAN_POINT('Ctrl Pts',(-0.158570730810153,-0.0609601945506607,
7.7));
#28284=CARTESIAN_POINT('Ctrl Pts',(-0.157322623531278,-0.0653756867109852,
7.7));
#28285=CARTESIAN_POINT('Ctrl Pts',(-0.155896079860197,-0.0697409359454714,
7.7));
#28286=CARTESIAN_POINT('Ctrl Pts',(-0.154356538303328,-0.0744519607383432,
7.7));
#28287=CARTESIAN_POINT('Ctrl Pts',(-0.152611566158709,-0.0790965634596896,
7.7));
#28288=CARTESIAN_POINT('Ctrl Pts',(-0.150674785237903,-0.0836580319983892,
7.7));
#28289=CARTESIAN_POINT('Ctrl Pts',(-0.147454105252843,-0.0912433144984649,
7.7));
#28290=CARTESIAN_POINT('Ctrl Pts',(-0.143701880264036,-0.0986043779779707,
7.7));
#28291=CARTESIAN_POINT('Ctrl Pts',(-0.139461085361289,-0.105692986452679,
7.7));
#28292=CARTESIAN_POINT('Ctrl Pts',(-0.137608088276184,-0.10879032342424,
7.7));
#28293=CARTESIAN_POINT('Ctrl Pts',(-0.135661951863532,-0.111834721508838,
7.7));
#28294=CARTESIAN_POINT('Ctrl Pts',(-0.13363213961135,-0.11481369464043,
7.7));
#28295=CARTESIAN_POINT('Ctrl Pts',(-0.126756583131934,-0.124904331345827,
7.7));
#28296=CARTESIAN_POINT('Ctrl Pts',(-0.118909175019161,-0.134272394153242,
7.7));
#28297=CARTESIAN_POINT('Ctrl Pts',(-0.110223618856625,-0.142769381443324,
7.7));
#28298=CARTESIAN_POINT('Ctrl Pts',(-0.105993896729624,-0.146907273649781,
7.7));
#28299=CARTESIAN_POINT('Ctrl Pts',(-0.101564626738699,-0.150838400565212,
7.7));
#28300=CARTESIAN_POINT('Ctrl Pts',(-0.0969473135927398,-0.154543558394273,
7.7));
#28301=CARTESIAN_POINT('Ctrl Pts',(-0.0930422781223282,-0.157677149790086,
7.7));
#28302=CARTESIAN_POINT('Ctrl Pts',(-0.08899818904879,-0.160651578311767,
7.7));
#28303=CARTESIAN_POINT('Ctrl Pts',(-0.0848474066780018,-0.163437744444605,
7.7));
#28304=CARTESIAN_POINT('Ctrl Pts',(-0.079772253597363,-0.166844384053503,
7.7));
#28305=CARTESIAN_POINT('Ctrl Pts',(-0.0745321224498625,-0.169974878347106,
7.7));
#28306=CARTESIAN_POINT('Ctrl Pts',(-0.0691422613850421,-0.172811109554059,
7.7));
#28307=CARTESIAN_POINT('Ctrl Pts',(-0.0615696806179204,-0.176795922823006,
7.7));
#28308=CARTESIAN_POINT('Ctrl Pts',(-0.0537018592997504,-0.18020049056539,
7.7));
#28309=CARTESIAN_POINT('Ctrl Pts',(-0.0456056057838966,-0.183040542196704,
7.7));
#28310=CARTESIAN_POINT('Ctrl Pts',(-0.0396967750000661,-0.18511327676139,
7.7));
#28311=CARTESIAN_POINT('Ctrl Pts',(-0.0336660415152703,-0.186885115293174,
7.7));
#28312=CARTESIAN_POINT('Ctrl Pts',(-0.0275371423493659,-0.188358530007864,
7.7));
#28313=CARTESIAN_POINT('Ctrl Pts',(-0.024009864278576,-0.189206503399434,
7.7));
#28314=CARTESIAN_POINT('Ctrl Pts',(-0.0204545422857024,-0.189954336779538,
7.7));
#28315=CARTESIAN_POINT('Ctrl Pts',(-0.0168840012680182,-0.190601758687094,
7.7));
#28316=CARTESIAN_POINT('Ctrl Pts',(-0.00536605034748104,-0.192690230355445,
7.7));
#28317=CARTESIAN_POINT('Ctrl Pts',(0.00633317552139851,-0.193742280465429,
7.7));
#28318=CARTESIAN_POINT('Ctrl Pts',(0.0180567949009463,-0.193791221918947,
7.7));
#28319=CARTESIAN_POINT('Ctrl Pts',(0.0247195011198704,-0.193819036070547,
7.7));
#28320=CARTESIAN_POINT('Ctrl Pts',(0.0313904746155388,-0.193522273036976,
7.7));
#28321=CARTESIAN_POINT('Ctrl Pts',(0.0380425876903635,-0.192902235229704,
7.7));
#28322=CARTESIAN_POINT('Ctrl Pts',(0.0421423475916298,-0.192520100092953,
7.7));
#28323=CARTESIAN_POINT('Ctrl Pts',(0.0462370105106329,-0.192014780875721,
7.7));
#28324=CARTESIAN_POINT('Ctrl Pts',(0.0503137405327971,-0.191386921964521,
7.7));
#28325=CARTESIAN_POINT('Ctrl Pts',(0.0635704399020003,-0.189345252099999,
7.7));
#28326=CARTESIAN_POINT('Ctrl Pts',(0.0765507573577913,-0.186026204674558,
7.7));
#28327=CARTESIAN_POINT('Ctrl Pts',(0.0890404097591069,-0.181462425248743,
7.7));
#28328=CARTESIAN_POINT('Ctrl Pts',(0.0993752126604044,-0.177686038257715,
7.7));
#28329=CARTESIAN_POINT('Ctrl Pts',(0.10937505445883,-0.17305651193581,7.7));
#28330=CARTESIAN_POINT('Ctrl Pts',(0.118916725392593,-0.167565356836862,
7.7));
#28331=CARTESIAN_POINT('Ctrl Pts',(0.120071034691086,-0.166901061093047,
7.7));
#28332=CARTESIAN_POINT('Ctrl Pts',(0.121218627187633,-0.166224125239918,
7.7));
#28333=CARTESIAN_POINT('Ctrl Pts',(0.122359422806361,-0.16553471763581,
7.7));
#28334=CARTESIAN_POINT('Ctrl Pts',(0.188262750966371,-0.0823232180103171,
7.7));
#28335=CARTESIAN_POINT('Ctrl Pts',(0.190918677948539,-0.0742706170903244,
7.7));
#28336=CARTESIAN_POINT('Ctrl Pts',(0.193028141056754,-0.0660604186529042,
7.7));
#28337=CARTESIAN_POINT('Ctrl Pts',(0.194603503553809,-0.057743966976229,
7.7));
#28338=CARTESIAN_POINT('Ctrl Pts',(0.195790000725462,-0.0514803632589782,
7.7));
#28339=CARTESIAN_POINT('Ctrl Pts',(0.196673340762519,-0.0451564294165951,
7.7));
#28340=CARTESIAN_POINT('Ctrl Pts',(0.197255694122567,-0.038794370326094,
7.7));
#28341=CARTESIAN_POINT('Ctrl Pts',(0.197691802090699,-0.0340300041294915,
7.7));
#28342=CARTESIAN_POINT('Ctrl Pts',(0.197958654381779,-0.0292456271837883,
7.7));
#28343=CARTESIAN_POINT('Ctrl Pts',(0.198057134112497,-0.0244628264544613,
7.7));
#28344=CARTESIAN_POINT('Ctrl Pts',(0.1982631637461,-0.0144567198712174,
7.7));
#28345=CARTESIAN_POINT('Ctrl Pts',(0.197734824507455,-0.00444255766703843,
7.7));
#28346=CARTESIAN_POINT('Ctrl Pts',(0.196479778415613,0.00549131122160059,
7.7));
#28347=CARTESIAN_POINT('Ctrl Pts',(0.195824459991882,0.0106782500471663,
7.7));
#28348=CARTESIAN_POINT('Ctrl Pts',(0.194969728524037,0.0158462023683286,
7.7));
#28349=CARTESIAN_POINT('Ctrl Pts',(0.193921197678987,0.020957521647447,
7.7));
#28350=CARTESIAN_POINT('Ctrl Pts',(0.191354737801022,0.0334683561310013,
7.7));
#28351=CARTESIAN_POINT('Ctrl Pts',(0.187627993625845,0.0456724030605818,
7.7));
#28352=CARTESIAN_POINT('Ctrl Pts',(0.182754547435098,0.0573811610434715,
7.7));
#28353=CARTESIAN_POINT('Ctrl Pts',(0.180516962808123,0.0627570974625973,
7.7));
#28354=CARTESIAN_POINT('Ctrl Pts',(0.178037027139388,0.0680282734604574,
7.7));
#28355=CARTESIAN_POINT('Ctrl Pts',(0.17531313072872,0.0731739851680651,
7.7));
#28356=CARTESIAN_POINT('Ctrl Pts',(0.173532663111309,0.0765374658893014,
7.7));
#28357=CARTESIAN_POINT('Ctrl Pts',(0.171646852120024,0.0798490434275999,
7.7));
#28358=CARTESIAN_POINT('Ctrl Pts',(0.169658294487776,0.0830968889931883,
7.7));
#28359=CARTESIAN_POINT('Ctrl Pts',(0.165386261266014,0.0900742598927501,
7.7));
#28360=CARTESIAN_POINT('Ctrl Pts',(0.160657770577514,0.0967310568420072,
7.7));
#28361=CARTESIAN_POINT('Ctrl Pts',(0.155474920208509,0.103014960516334,
7.7));
#28362=CARTESIAN_POINT('Ctrl Pts',(0.149769902176698,0.109931962015469,
7.7));
#28363=CARTESIAN_POINT('Ctrl Pts',(0.143514168159607,0.116397450963363,
7.7));
#28364=CARTESIAN_POINT('Ctrl Pts',(0.136780000787126,0.122378418898736,
7.7));
#28365=CARTESIAN_POINT('Ctrl Pts',(0.13253962121023,0.126144522840088,7.7));
#28366=CARTESIAN_POINT('Ctrl Pts',(0.128109373210913,0.129718271038147,
7.7));
#28367=CARTESIAN_POINT('Ctrl Pts',(0.123506439942429,0.133088658006456,
7.7));
#28368=CARTESIAN_POINT('Ctrl Pts',(0.120698151327833,0.135144959672763,
7.7));
#28369=CARTESIAN_POINT('Ctrl Pts',(0.117828933115805,0.137122882548733,
7.7));
#28370=CARTESIAN_POINT('Ctrl Pts',(0.11490983233649,0.139016243048957,7.7));
#28371=CARTESIAN_POINT('Ctrl Pts',(0.10629614374237,0.144603175114098,7.7));
#28372=CARTESIAN_POINT('Ctrl Pts',(0.0972315481938087,0.14946836034174,
7.7));
#28373=CARTESIAN_POINT('Ctrl Pts',(0.087825129619459,0.153560681874093,
7.7));
#28374=CARTESIAN_POINT('Ctrl Pts',(0.0790043519078121,0.157398216667612,
7.7));
#28375=CARTESIAN_POINT('Ctrl Pts',(0.0698823201879155,0.160556069597663,
7.7));
#28376=CARTESIAN_POINT('Ctrl Pts',(0.0605484824963349,0.162970283178604,
7.7));
#28377=CARTESIAN_POINT('Ctrl Pts',(0.0570499058412824,0.163875196200845,
7.7));
#28378=CARTESIAN_POINT('Ctrl Pts',(0.0535300157362907,0.164673163118735,
7.7));
#28379=CARTESIAN_POINT('Ctrl Pts',(0.0499970990922767,0.165361152486414,
7.7));
#28380=CARTESIAN_POINT('Ctrl Pts',(0.0389156579059496,0.167519118406066,
7.7));
#28381=CARTESIAN_POINT('Ctrl Pts',(0.027694369523137,0.1686015574444,7.7));
#28382=CARTESIAN_POINT('Ctrl Pts',(0.0164838938501993,0.168511920108317,
7.7));
#28383=CARTESIAN_POINT('Ctrl Pts',(0.0102987918414279,0.168462464930531,
7.7));
#28384=CARTESIAN_POINT('Ctrl Pts',(0.00411708598692211,0.168055390254949,
7.7));
#28385=CARTESIAN_POINT('Ctrl Pts',(-0.00203360988862401,0.167267947758606,
7.7));
#28386=CARTESIAN_POINT('Ctrl Pts',(-0.00310929540839016,0.167130233179946,
7.7));
#28387=CARTESIAN_POINT('Ctrl Pts',(-0.00418402611025386,0.166980872543433,
7.7));
#28388=CARTESIAN_POINT('Ctrl Pts',(-0.00525764907570514,0.166819936918742,
7.7));
#28389=CARTESIAN_POINT('Origin',(0.,0.,8.75459252805377));
#28390=CARTESIAN_POINT('Ctrl Pts',(-0.205656479110814,0.000149599810560778,
8.57959252805377));
#28391=CARTESIAN_POINT('Ctrl Pts',(-0.205738361598484,0.00997856061592459,
8.57905813053169));
#28392=CARTESIAN_POINT('Ctrl Pts',(-0.200629066917608,0.0878617486383526,
8.57481913665734));
#28393=CARTESIAN_POINT('Ctrl Pts',(-0.101094553526346,0.220843047088143,
8.56687554643072));
#28394=CARTESIAN_POINT('Ctrl Pts',(0.130699637719291,0.204687395831059,
8.55576175737394));
#28395=CARTESIAN_POINT('Ctrl Pts',(0.242861169103291,0.00121341226084251,
8.5446479683171));
#28396=CARTESIAN_POINT('Ctrl Pts',(0.132730025418579,-0.203388545171364,
8.53353417926033));
#28397=CARTESIAN_POINT('Ctrl Pts',(-0.0988908732032454,-0.221817926612619,
8.5224203902035));
#28398=CARTESIAN_POINT('Ctrl Pts',(-0.200214859662634,-0.089261959020885,
8.51443983980133));
#28399=CARTESIAN_POINT('Ctrl Pts',(-0.205728077932475,-0.0106740791790422,
8.51016388575142));
#28400=CARTESIAN_POINT('Ctrl Pts',(-0.205637856381221,-0.000160393794940828,
8.50959252805377));
#28401=CARTESIAN_POINT('Ctrl Pts',(-0.205267617401664,-0.000235214789251429,
8.58540747194623));
#28402=CARTESIAN_POINT('Ctrl Pts',(-0.204912371893322,0.0467865688130083,
8.58286245525962));
#28403=CARTESIAN_POINT('Ctrl Pts',(-0.165653744048178,0.162957645782203,
8.57661284222074));
#28404=CARTESIAN_POINT('Ctrl Pts',(0.027212997215315,0.241280498724425,
8.56665863282958));
#28405=CARTESIAN_POINT('Ctrl Pts',(0.217474198098902,0.108094945242369,
8.5555448437728));
#28406=CARTESIAN_POINT('Ctrl Pts',(0.208761552554325,-0.124138522922833,
8.54443105471596));
#28407=CARTESIAN_POINT('Ctrl Pts',(0.00892537992430322,-0.24269250748312,
8.53331726565919));
#28408=CARTESIAN_POINT('Ctrl Pts',(-0.172124770298785,-0.152545548970925,
8.52364273806925));
#28409=CARTESIAN_POINT('Ctrl Pts',(-0.204991280139091,-0.0417919262244986,
8.51767280683161));
#28410=CARTESIAN_POINT('Ctrl Pts',(-0.205208153945529,0.00011616087473525,
8.51540747194623));
#28411=CARTESIAN_POINT('Ctrl Pts',(0.126907087985233,0.107935865304858,
8.6));
#28412=CARTESIAN_POINT('Ctrl Pts',(0.162798331100656,0.0657362393039593,
8.59629540364773));
#28413=CARTESIAN_POINT('Ctrl Pts',(0.188528583981656,-0.0565786457595969,
8.5888862109432));
#28414=CARTESIAN_POINT('Ctrl Pts',(0.0545086267819675,-0.189344482047467,
8.57777242188639));
#28415=CARTESIAN_POINT('Ctrl Pts',(-0.129420383958987,-0.148353651561752,
8.56665863282959));
#28416=CARTESIAN_POINT('Ctrl Pts',(-0.194878571858316,0.0282081923545751,
8.55554484377279));
#28417=CARTESIAN_POINT('Ctrl Pts',(-0.0819678920427756,0.179060477648788,
8.54443105471597));
#28418=CARTESIAN_POINT('Ctrl Pts',(0.105971819657057,0.165961407205034,
8.53331726565919));
#28419=CARTESIAN_POINT('Ctrl Pts',(0.196912864205418,0.00098383979878997,
8.52220347660236));
#28420=CARTESIAN_POINT('Ctrl Pts',(0.107618066600488,-0.164908293590701,
8.51108968754557));
#28421=CARTESIAN_POINT('Ctrl Pts',(-0.0801811387062207,-0.179850914094962,
8.49997589848876));
#28422=CARTESIAN_POINT('Ctrl Pts',(-0.194589451459316,-0.0301775235439226,
8.48886210943196));
#28423=CARTESIAN_POINT('Ctrl Pts',(-0.130887926765565,0.147119496537145,
8.47774832037516));
#28424=CARTESIAN_POINT('Ctrl Pts',(0.0526168491933447,0.189755465499352,
8.46663453131834));
#28425=CARTESIAN_POINT('Ctrl Pts',(0.187960802408794,0.0587065624392284,
8.45552074226155));
#28426=CARTESIAN_POINT('Ctrl Pts',(0.151262113639308,-0.126077353665056,
8.44440695320474));
#28427=CARTESIAN_POINT('Ctrl Pts',(-0.0238885092637228,-0.195461121852156,
8.43329316414793));
#28428=CARTESIAN_POINT('Ctrl Pts',(-0.177173705652972,-0.0859371671587494,
8.42217937509113));
#28429=CARTESIAN_POINT('Ctrl Pts',(-0.168289801519644,0.102246080788216,
8.41106558603433));
#28430=CARTESIAN_POINT('Ctrl Pts',(-0.00536833273875009,0.196842316537561,
8.39995179697752));
#28431=CARTESIAN_POINT('Ctrl Pts',(0.162466831485467,0.111266555129785,
8.38883800792072));
#28432=CARTESIAN_POINT('Ctrl Pts',(0.181594262550234,-0.0761527498248231,
8.37772421886392));
#28433=CARTESIAN_POINT('Ctrl Pts',(0.0345064055837472,-0.193868577324089,
8.36661042980711));
#28434=CARTESIAN_POINT('Ctrl Pts',(-0.144165555692373,-0.134134298342242,
8.3554966407503));
#28435=CARTESIAN_POINT('Ctrl Pts',(-0.190881148920086,0.0483746255840866,
8.34438285169351));
#28436=CARTESIAN_POINT('Ctrl Pts',(-0.0628810617889658,0.186605705863002,
8.3332690626367));
#28437=CARTESIAN_POINT('Ctrl Pts',(0.122674774310876,0.154034467436257,
8.3221552735799));
#28438=CARTESIAN_POINT('Ctrl Pts',(0.195944998260667,-0.019526265966773,
8.31104148452309));
#28439=CARTESIAN_POINT('Ctrl Pts',(0.0898645431334079,-0.175214386656136,
8.29992769546628));
#28440=CARTESIAN_POINT('Ctrl Pts',(-0.0984699474562653,-0.170526792188656,
8.28881390640949));
#28441=CARTESIAN_POINT('Ctrl Pts',(-0.19667377841448,-0.00975409091757148,
8.27770011735268));
#28442=CARTESIAN_POINT('Ctrl Pts',(-0.114859869557362,0.159946640385262,
8.26658632829587));
#28443=CARTESIAN_POINT('Ctrl Pts',(0.0720865805050185,0.183246397827218,
8.25547253923907));
#28444=CARTESIAN_POINT('Ctrl Pts',(0.193051365913784,0.0388186491814046,
8.24435875018227));
#28445=CARTESIAN_POINT('Ctrl Pts',(0.13731404675024,-0.141140249293057,
8.23324496112546));
#28446=CARTESIAN_POINT('Ctrl Pts',(-0.0441083766509897,-0.19191187695055,
8.22213117206866));
#28447=CARTESIAN_POINT('Ctrl Pts',(-0.185157902680562,-0.0670243872063616,
8.21101738301184));
#28448=CARTESIAN_POINT('Ctrl Pts',(-0.156730300553177,0.119211284255993,
8.19990359395506));
#28449=CARTESIAN_POINT('Ctrl Pts',(0.0151543231130278,0.196331515290955,
8.18878980489823));
#28450=CARTESIAN_POINT('Ctrl Pts',(0.173168022972167,0.0937472838292696,
8.17767601584145));
#28451=CARTESIAN_POINT('Ctrl Pts',(0.17267906754593,-0.0946448996878474,
8.16656222678463));
#28452=CARTESIAN_POINT('Ctrl Pts',(0.014135003281085,-0.196407533174517,
8.15544843772784));
#28453=CARTESIAN_POINT('Ctrl Pts',(-0.157346989788777,-0.118396124133627,
8.14433464867103));
#28454=CARTESIAN_POINT('Ctrl Pts',(-0.184807498668741,0.0679846000301397,
8.13322085961422));
#28455=CARTESIAN_POINT('Ctrl Pts',(-0.0431116081576236,0.192138248788519,
8.12210707055742));
#28456=CARTESIAN_POINT('Ctrl Pts',(0.138044826219057,0.14042557943482,8.11099328150061));
#28457=CARTESIAN_POINT('Ctrl Pts',(0.192847265622626,-0.0398202153099506,
8.09987949244382));
#28458=CARTESIAN_POINT('Ctrl Pts',(0.0711344157650659,-0.183618115389575,
8.08876570338701));
#28459=CARTESIAN_POINT('Ctrl Pts',(-0.115688571561406,-0.159348272082047,
8.0776519143302));
#28460=CARTESIAN_POINT('Ctrl Pts',(-0.196620497340079,0.0107748517944625,
8.06653812527341));
#28461=CARTESIAN_POINT('Ctrl Pts',(-0.0975834520752944,0.171035631628434,
8.05542433621659));
#28462=CARTESIAN_POINT('Ctrl Pts',(0.0907728335456545,0.174745558156785,
8.0443105471598));
#28463=CARTESIAN_POINT('Ctrl Pts',(0.196043715188255,0.0185088935550664,
8.03319675810298));
#28464=CARTESIAN_POINT('Ctrl Pts',(0.121873561032224,-0.154669171223235,
8.02208296904619));
#28465=CARTESIAN_POINT('Ctrl Pts',(-0.0638488456770328,-0.186276789512212,
8.01096917998937));
#28466=CARTESIAN_POINT('Ctrl Pts',(-0.19112967984246,-0.0473831498401582,
7.99985539093258));
#28467=CARTESIAN_POINT('Ctrl Pts',(-0.143467350491047,0.134880824245969,
7.98874160187577));
#28468=CARTESIAN_POINT('Ctrl Pts',(0.0355122717971353,0.193686850239423,
7.97762781281897));
#28469=CARTESIAN_POINT('Ctrl Pts',(0.181987108969079,0.075209105665833,
7.96651402376217));
#28470=CARTESIAN_POINT('Ctrl Pts',(0.161887081434908,-0.112108386283467,
7.95540023470535));
#28471=CARTESIAN_POINT('Ctrl Pts',(-0.00639002767582873,-0.196811800811433,
7.94428644564855));
#28472=CARTESIAN_POINT('Ctrl Pts',(-0.168818271957638,-0.101371142179071,
7.93317265659175));
#28473=CARTESIAN_POINT('Ctrl Pts',(-0.176725237445514,0.086855672754766,
7.92205886753494));
#28474=CARTESIAN_POINT('Ctrl Pts',(-0.0228735887833459,0.195582504933715,
7.91094507847814));
#28475=CARTESIAN_POINT('Ctrl Pts',(0.151914514866951,0.125290453226829,
7.89983128942133));
#28476=CARTESIAN_POINT('Ctrl Pts',(0.18765354068678,-0.0596813730664067,
7.88871750036453));
#28477=CARTESIAN_POINT('Ctrl Pts',(0.0516311516775647,-0.190026158074923,
7.87760371130772));
#28478=CARTESIAN_POINT('Ctrl Pts',(-0.131649814209033,-0.146437852861883,
7.86648992225093));
#28479=CARTESIAN_POINT('Ctrl Pts',(-0.194430215690457,0.0311866942884203,
7.85537613319412));
#28480=CARTESIAN_POINT('Ctrl Pts',(-0.0792464287188404,0.180265677725562,
7.84426234413731));
#28481=CARTESIAN_POINT('Ctrl Pts',(0.108472499205164,0.164345499013512,
7.83314855508052));
#28482=CARTESIAN_POINT('Ctrl Pts',(0.196905346153373,-0.00200209185834237,
7.8220347660237));
#28483=CARTESIAN_POINT('Ctrl Pts',(0.105108441749456,-0.166516920998775,
7.8109209769669));
#28484=CARTESIAN_POINT('Ctrl Pts',(-0.0828953023872357,-0.17861736891036,
7.7998071879101));
#28485=CARTESIAN_POINT('Ctrl Pts',(-0.195024252374675,-0.0272264307646135,
7.78869339885329));
#28486=CARTESIAN_POINT('Ctrl Pts',(-0.128644863563789,0.149083417534189,
7.77757960979649));
#28487=CARTESIAN_POINT('Ctrl Pts',(0.0554837771323393,0.188938995522239,
7.76646582073968));
#28488=CARTESIAN_POINT('Ctrl Pts',(0.188829174678946,0.0558496805756237,
7.75535203168288));
#28489=CARTESIAN_POINT('Ctrl Pts',(0.149333740426706,-0.128345818837516,
7.74423824262607));
#28490=CARTESIAN_POINT('Ctrl Pts',(-0.0268419213711513,-0.195092032740585,
7.73312445356928));
#28491=CARTESIAN_POINT('Ctrl Pts',(-0.178462040649008,-0.0832145415948537,
7.72201066451247));
#28492=CARTESIAN_POINT('Ctrl Pts',(-0.166707642915459,0.104723462076886,
7.71089687545566));
#28493=CARTESIAN_POINT('Ctrl Pts',(-0.00241652804585203,0.197019500729453,
7.69978308639886));
#28494=CARTESIAN_POINT('Ctrl Pts',(0.164199550234369,0.108548043911206,
7.68866929734206));
#28495=CARTESIAN_POINT('Ctrl Pts',(0.174839538171075,-0.0159901738299269,
7.68126010463752));
#28496=CARTESIAN_POINT('Ctrl Pts',(0.15264423560529,-0.0667480137268267,
7.67755550828525));
#28497=CARTESIAN_POINT('Ctrl Pts',(0.136778062465877,0.116331236980981,
8.60748149723825));
#28498=CARTESIAN_POINT('Ctrl Pts',(0.17546096639785,0.0708492771249706,
8.60377690088598));
#28499=CARTESIAN_POINT('Ctrl Pts',(0.203192546971425,-0.0609793957674089,
8.59636770818145));
#28500=CARTESIAN_POINT('Ctrl Pts',(0.0587483684109172,-0.204071906496436,
8.58525391912464));
#28501=CARTESIAN_POINT('Ctrl Pts',(-0.139486845396373,-0.159892763615499,
8.57414013006784));
#28502=CARTESIAN_POINT('Ctrl Pts',(-0.210036443969145,0.0304022569359761,
8.56302634101102));
#28503=CARTESIAN_POINT('Ctrl Pts',(-0.0883434458706326,0.19298800079524,
8.55191255195424));
#28504=CARTESIAN_POINT('Ctrl Pts',(0.114214425677802,0.178870070080376,
8.54079876289742));
#28505=CARTESIAN_POINT('Ctrl Pts',(0.212228965838042,0.00106036395280743,
8.52968497384062));
#28506=CARTESIAN_POINT('Ctrl Pts',(0.115988719539852,-0.177735044117588,
8.51857118478382));
#28507=CARTESIAN_POINT('Ctrl Pts',(-0.0864177168718956,-0.193839918267514,
8.50745739572701));
#28508=CARTESIAN_POINT('Ctrl Pts',(-0.209724835463879,-0.0325247648960035,
8.49634360667021));
#28509=CARTESIAN_POINT('Ctrl Pts',(-0.141068535315007,0.15856261464015,
8.4852298176134));
#28510=CARTESIAN_POINT('Ctrl Pts',(0.0567094462569527,0.204514856698406,
8.4741160285566));
#28511=CARTESIAN_POINT('Ctrl Pts',(0.202580602716201,0.0632728241735722,
8.46300223949979));
#28512=CARTESIAN_POINT('Ctrl Pts',(0.163027449108952,-0.135883790487243,
8.45188845044298));
#28513=CARTESIAN_POINT('Ctrl Pts',(-0.0257465840889073,-0.210664305349561,
8.44077466138619));
#28514=CARTESIAN_POINT('Ctrl Pts',(-0.190954473574659,-0.092621455620727,
8.42966087232938));
#28515=CARTESIAN_POINT('Ctrl Pts',(-0.181379569494986,0.110198894695063,
8.41854708327258));
#28516=CARTESIAN_POINT('Ctrl Pts',(-0.00578588763114495,0.212152930894099,
8.40743329421577));
#28517=CARTESIAN_POINT('Ctrl Pts',(0.175103682373818,0.1199209915657,8.39631950515897));
#28518=CARTESIAN_POINT('Ctrl Pts',(0.195718866305016,-0.082075995421942,
8.38520571610216));
#28519=CARTESIAN_POINT('Ctrl Pts',(0.0371903521965286,-0.208947890936482,
8.37409192704536));
#28520=CARTESIAN_POINT('Ctrl Pts',(-0.155378912990374,-0.144567413284328,
8.36297813798855));
#28521=CARTESIAN_POINT('Ctrl Pts',(-0.205728097027866,0.0521372577761262,
8.35186434893175));
#28522=CARTESIAN_POINT('Ctrl Pts',(-0.067772020726633,0.201120105253607,
8.34075055987495));
#28523=CARTESIAN_POINT('Ctrl Pts',(0.132216554725712,0.166015439668319,
8.32963677081815));
#28524=CARTESIAN_POINT('Ctrl Pts',(0.211185818203411,-0.0210450406555653,
8.31852298176134));
#28525=CARTESIAN_POINT('Ctrl Pts',(0.0968543072676843,-0.188842756566615,
8.30740919270453));
#28526=CARTESIAN_POINT('Ctrl Pts',(-0.106129049511812,-0.183790555786764,
8.29629540364774));
#28527=CARTESIAN_POINT('Ctrl Pts',(-0.211971283688315,-0.0105127749600295,
8.28518161459092));
#28528=CARTESIAN_POINT('Ctrl Pts',(-0.123793797986818,0.172387468006265,
8.27406782553413));
#28529=CARTESIAN_POINT('Ctrl Pts',(0.0776935549290535,0.197499506501754,
8.26295403647731));
#28530=CARTESIAN_POINT('Ctrl Pts',(0.20806711591358,0.0418380068983455,
8.25184024742052));
#28531=CARTESIAN_POINT('Ctrl Pts',(0.147994486060795,-0.152118294893832,
8.24072645836371));
#28532=CARTESIAN_POINT('Ctrl Pts',(-0.0475391752550459,-0.206838996231168,
8.22961266930691));
#28533=CARTESIAN_POINT('Ctrl Pts',(-0.199559690329035,-0.0722376186042153,
8.2184988802501));
#28534=CARTESIAN_POINT('Ctrl Pts',(-0.168920957684039,0.128483670561418,
8.2073850911933));
#28535=CARTESIAN_POINT('Ctrl Pts',(0.0163330432231097,0.211602398958294,
8.19627130213649));
#28536=CARTESIAN_POINT('Ctrl Pts',(0.186637224438839,0.101039051854205,
8.1851575130797));
#28537=CARTESIAN_POINT('Ctrl Pts',(0.186110237515614,-0.102006485272812,
8.17404372402288));
#28538=CARTESIAN_POINT('Ctrl Pts',(0.0152344395607012,-0.211684329597404,
8.16292993496609));
#28539=CARTESIAN_POINT('Ctrl Pts',(-0.169585613694417,-0.127605106377914,
8.15181614590927));
#28540=CARTESIAN_POINT('Ctrl Pts',(-0.199182031503369,0.0732725178496109,
8.14070235685248));
#28541=CARTESIAN_POINT('Ctrl Pts',(-0.0464648769994157,0.20708297552252,
8.12958856779566));
#28542=CARTESIAN_POINT('Ctrl Pts',(0.148782106369649,0.151348037218991,
8.11847477873887));
#28543=CARTESIAN_POINT('Ctrl Pts',(0.207847140474726,-0.0429174759545572,
8.10736098968206));
#28544=CARTESIAN_POINT('Ctrl Pts',(0.0766673297563964,-0.197900136669627,
8.09624720062525));
#28545=CARTESIAN_POINT('Ctrl Pts',(-0.124686957354622,-0.171742557950773,
8.08513341156845));
#28546=CARTESIAN_POINT('Ctrl Pts',(-0.211913858352676,0.0116129317534655,
8.07401962251165));
#28547=CARTESIAN_POINT('Ctrl Pts',(-0.105173601533932,0.184338973324224,
8.06290583345484));
#28548=CARTESIAN_POINT('Ctrl Pts',(0.0978332455186183,0.188337462065038,
8.05179204439804));
#28549=CARTESIAN_POINT('Ctrl Pts',(0.211292213443444,0.0199485358859052,
8.04067825534123));
#28550=CARTESIAN_POINT('Ctrl Pts',(0.131353022186941,-0.166699511421921,
8.02956446628443));
#28551=CARTESIAN_POINT('Ctrl Pts',(-0.06881507992212,-0.200765605423151,
8.01845067722763));
#28552=CARTESIAN_POINT('Ctrl Pts',(-0.205995958961859,-0.0510686639458728,
8.00733688817082));
#28553=CARTESIAN_POINT('Ctrl Pts',(-0.154626400611774,0.145372004803316,
7.99622309911402));
#28554=CARTESIAN_POINT('Ctrl Pts',(0.0382744558029648,0.208752028917009,
7.98510931005722));
#28555=CARTESIAN_POINT('Ctrl Pts',(0.19614226875534,0.0810589535705133,
7.97399552100041));
#28556=CARTESIAN_POINT('Ctrl Pts',(0.174478838719386,-0.120828301283006,
7.96288173194361));
#28557=CARTESIAN_POINT('Ctrl Pts',(-0.0068870511370089,-0.212120041620846,
7.95176794288681));
#28558=CARTESIAN_POINT('Ctrl Pts',(-0.181949144951542,-0.109255902387577,
7.94065415382999));
#28559=CARTESIAN_POINT('Ctrl Pts',(-0.190471123011129,0.0936114036037888,
7.9295403647732));
#28560=CARTESIAN_POINT('Ctrl Pts',(-0.0246527219645235,0.210795129742235,
7.91842657571639));
#28561=CARTESIAN_POINT('Ctrl Pts',(0.163730594829841,0.135035684057547,
7.90731278665958));
#28562=CARTESIAN_POINT('Ctrl Pts',(0.202249441835637,-0.0643234566557557,
7.89619899760278));
#28563=CARTESIAN_POINT('Ctrl Pts',(0.055647080091861,-0.204806604043635,
7.88508520854598));
#28564=CARTESIAN_POINT('Ctrl Pts',(-0.141889683211386,-0.157827951961535,
7.87397141948916));
#28565=CARTESIAN_POINT('Ctrl Pts',(-0.209553214159777,0.033612430063655,
7.86285763043237));
#28566=CARTESIAN_POINT('Ctrl Pts',(-0.0854103041018835,0.194286942674705,
7.85174384137556));
#28567=CARTESIAN_POINT('Ctrl Pts',(0.116909610863029,0.177128474752108,
7.84063005231877));
#28568=CARTESIAN_POINT('Ctrl Pts',(0.212220863023546,-0.00215781679030121,
7.82951626326195));
#28569=CARTESIAN_POINT('Ctrl Pts',(0.113283893276087,-0.179468792354972,
7.81840247420515));
#28570=CARTESIAN_POINT('Ctrl Pts',(-0.0893429912233777,-0.192510426566203,
7.80728868514835));
#28571=CARTESIAN_POINT('Ctrl Pts',(-0.210193455678128,-0.0293441328373914,
7.79617489609154));
#28572=CARTESIAN_POINT('Ctrl Pts',(-0.138651004162113,0.160679291597098,
7.78506110703474));
#28573=CARTESIAN_POINT('Ctrl Pts',(0.0597993670403417,0.203634880778195,
7.77394731797793));
#28574=CARTESIAN_POINT('Ctrl Pts',(0.203516517947542,0.0601937308604925,
7.76283352892113));
#28575=CARTESIAN_POINT('Ctrl Pts',(0.160949084882664,-0.13832869940436,
7.75171973986433));
#28576=CARTESIAN_POINT('Ctrl Pts',(-0.02892971587556,-0.210266508076299,
7.74060595080753));
#28577=CARTESIAN_POINT('Ctrl Pts',(-0.192343016699888,-0.0896870612117004,
7.72949216175072));
#28578=CARTESIAN_POINT('Ctrl Pts',(-0.179674348834503,0.112868969456315,
7.71837837269391));
#28579=CARTESIAN_POINT('Ctrl Pts',(-0.00260448828551292,0.212343896669543,
7.7072645836371));
#28580=CARTESIAN_POINT('Ctrl Pts',(0.176971173914563,0.116991031520346,
7.69615079458031));
#28581=CARTESIAN_POINT('Ctrl Pts',(0.188438751949387,-0.0172339073386072,
7.68874160187577));
#28582=CARTESIAN_POINT('Ctrl Pts',(0.164517074058983,-0.071939748487992,
7.6850370055235));
#28583=CARTESIAN_POINT('Ctrl Pts',(0.146649036946521,0.124726608657104,
8.6149629944765));
#28584=CARTESIAN_POINT('Ctrl Pts',(0.188123601695045,0.0759623149459817,
8.61125839812423));
#28585=CARTESIAN_POINT('Ctrl Pts',(0.217856509961195,-0.0653801457752205,
8.60384920541969));
#28586=CARTESIAN_POINT('Ctrl Pts',(0.0629881100398666,-0.218799330945407,
8.59273541636289));
#28587=CARTESIAN_POINT('Ctrl Pts',(-0.149553306833759,-0.171431875669247,
8.58162162730608));
#28588=CARTESIAN_POINT('Ctrl Pts',(-0.225194316079973,0.0325963215173767,
8.57050783824928));
#28589=CARTESIAN_POINT('Ctrl Pts',(-0.0947189996984894,0.206915523941692,
8.55939404919247));
#28590=CARTESIAN_POINT('Ctrl Pts',(0.122457031698546,0.191778732955717,
8.54828026013568));
#28591=CARTESIAN_POINT('Ctrl Pts',(0.227545067470666,0.00113688810682507,
8.53716647107886));
#28592=CARTESIAN_POINT('Ctrl Pts',(0.124359372479216,-0.190561794644476,
8.52605268202208));
#28593=CARTESIAN_POINT('Ctrl Pts',(-0.0926542950375705,-0.207828922440066,
8.51493889296525));
#28594=CARTESIAN_POINT('Ctrl Pts',(-0.224860219468443,-0.0348720062480843,
8.50382510390846));
#28595=CARTESIAN_POINT('Ctrl Pts',(-0.15124914386445,0.170005732743154,
8.49271131485166));
#28596=CARTESIAN_POINT('Ctrl Pts',(0.0608020433205606,0.219274247897461,
8.48159752579484));
#28597=CARTESIAN_POINT('Ctrl Pts',(0.217200403023608,0.0678390859079159,
8.47048373673806));
#28598=CARTESIAN_POINT('Ctrl Pts',(0.174792784578596,-0.14569022730943,
8.45936994768122));
#28599=CARTESIAN_POINT('Ctrl Pts',(-0.0276046589140918,-0.225867488846965,
8.44825615862445));
#28600=CARTESIAN_POINT('Ctrl Pts',(-0.204735241496347,-0.0993057440827045,
8.43714236956762));
#28601=CARTESIAN_POINT('Ctrl Pts',(-0.194469337470328,0.118151708601909,
8.42602858051083));
#28602=CARTESIAN_POINT('Ctrl Pts',(-0.00620344252353972,0.227463545250637,
8.41491479145402));
#28603=CARTESIAN_POINT('Ctrl Pts',(0.187740533262168,0.128575428001615,
8.40380100239722));
#28604=CARTESIAN_POINT('Ctrl Pts',(0.209843470059799,-0.0879992410190609,
8.39268721334041));
#28605=CARTESIAN_POINT('Ctrl Pts',(0.0398742988093101,-0.224027204548875,
8.38157342428361));
#28606=CARTESIAN_POINT('Ctrl Pts',(-0.166592270288375,-0.155000528226414,
8.3704596352268));
#28607=CARTESIAN_POINT('Ctrl Pts',(-0.220575045135645,0.0558998899681659,
8.35934584617));
#28608=CARTESIAN_POINT('Ctrl Pts',(-0.0726629796643001,0.215634504644212,
8.3482320571132));
#28609=CARTESIAN_POINT('Ctrl Pts',(0.141758335140549,0.17799641190038,8.3371182680564));
#28610=CARTESIAN_POINT('Ctrl Pts',(0.226426638146155,-0.0225638153443574,
8.32600447899959));
#28611=CARTESIAN_POINT('Ctrl Pts',(0.10384407140196,-0.202471126477093,
8.31489068994278));
#28612=CARTESIAN_POINT('Ctrl Pts',(-0.113788151567359,-0.197054319384871,
8.30377690088599));
#28613=CARTESIAN_POINT('Ctrl Pts',(-0.22726878896215,-0.0112714590024876,
8.29266311182917));
#28614=CARTESIAN_POINT('Ctrl Pts',(-0.132727726416275,0.184828295627267,
8.28154932277238));
#28615=CARTESIAN_POINT('Ctrl Pts',(0.0833005293530883,0.21175261517629,
8.27043553371557));
#28616=CARTESIAN_POINT('Ctrl Pts',(0.223082865913377,0.0448573646152865,
8.25932174465876));
#28617=CARTESIAN_POINT('Ctrl Pts',(0.158674925371351,-0.163096340494608,
8.24820795560196));
#28618=CARTESIAN_POINT('Ctrl Pts',(-0.050969973859102,-0.221766115511785,
8.23709416654516));
#28619=CARTESIAN_POINT('Ctrl Pts',(-0.213961477977508,-0.0774508500020691,
8.22598037748835));
#28620=CARTESIAN_POINT('Ctrl Pts',(-0.181111614814901,0.137756056866844,
8.21486658843155));
#28621=CARTESIAN_POINT('Ctrl Pts',(0.0175117633331917,0.226873282625633,
8.20375279937474));
#28622=CARTESIAN_POINT('Ctrl Pts',(0.200106425905512,0.108330819879141,
8.19263901031794));
#28623=CARTESIAN_POINT('Ctrl Pts',(0.199541407485298,-0.109368070857775,
8.18152522126113));
#28624=CARTESIAN_POINT('Ctrl Pts',(0.0163338758403174,-0.226961126020292,
8.17041143220434));
#28625=CARTESIAN_POINT('Ctrl Pts',(-0.181824237600056,-0.136814088622201,
8.15929764314752));
#28626=CARTESIAN_POINT('Ctrl Pts',(-0.213556564337998,0.0785604356690821,
8.14818385409073));
#28627=CARTESIAN_POINT('Ctrl Pts',(-0.0498181458412077,0.22202770225652,
8.13707006503391));
#28628=CARTESIAN_POINT('Ctrl Pts',(0.159519386520241,0.162270495003162,
8.12595627597712));
#28629=CARTESIAN_POINT('Ctrl Pts',(0.222847015326826,-0.0460147365991637,
8.1148424869203));
#28630=CARTESIAN_POINT('Ctrl Pts',(0.0822002437477268,-0.212182157949678,
8.10372869786351));
#28631=CARTESIAN_POINT('Ctrl Pts',(-0.133685343147839,-0.1841368438195,
8.09261490880669));
#28632=CARTESIAN_POINT('Ctrl Pts',(-0.227207219365272,0.0124510117124686,
8.0815011197499));
#28633=CARTESIAN_POINT('Ctrl Pts',(-0.11276375099257,0.197642315020013,
8.07038733069309));
#28634=CARTESIAN_POINT('Ctrl Pts',(0.104893657491582,0.201929365973291,
8.05927354163629));
#28635=CARTESIAN_POINT('Ctrl Pts',(0.226540711698633,0.0213881782167439,
8.04815975257947));
#28636=CARTESIAN_POINT('Ctrl Pts',(0.140832483341659,-0.178729851620607,
8.03704596352269));
#28637=CARTESIAN_POINT('Ctrl Pts',(-0.0737813141672074,-0.21525442133409,
8.02593217446587));
#28638=CARTESIAN_POINT('Ctrl Pts',(-0.220862238081258,-0.0547541780515873,
8.01481838540908));
#28639=CARTESIAN_POINT('Ctrl Pts',(-0.165785450732502,0.155863185360662,
8.00370459635226));
#28640=CARTESIAN_POINT('Ctrl Pts',(0.0410366398087944,0.223817207594595,
7.99259080729547));
#28641=CARTESIAN_POINT('Ctrl Pts',(0.2102974285416,0.0869088014751938,7.98147701823866));
#28642=CARTESIAN_POINT('Ctrl Pts',(0.187070596003864,-0.129548216282546,
7.97036322918185));
#28643=CARTESIAN_POINT('Ctrl Pts',(-0.00738407459818899,-0.227428282430258,
7.95924944012505));
#28644=CARTESIAN_POINT('Ctrl Pts',(-0.195080017945446,-0.117140662596084,
7.94813565106825));
#28645=CARTESIAN_POINT('Ctrl Pts',(-0.204217008576744,0.100367134452811,
7.93702186201144));
#28646=CARTESIAN_POINT('Ctrl Pts',(-0.026431855145701,0.226007754550755,
7.92590807295464));
#28647=CARTESIAN_POINT('Ctrl Pts',(0.175546674792731,0.144780914888265,
7.91479428389783));
#28648=CARTESIAN_POINT('Ctrl Pts',(0.216845342984493,-0.0689655402451044,
7.90368049484103));
#28649=CARTESIAN_POINT('Ctrl Pts',(0.0596630085061574,-0.219587050012348,
7.89256670578422));
#28650=CARTESIAN_POINT('Ctrl Pts',(-0.152129552213739,-0.169218051061186,
7.88145291672742));
#28651=CARTESIAN_POINT('Ctrl Pts',(-0.224676212629098,0.0360381658388899,
7.87033912767062));
#28652=CARTESIAN_POINT('Ctrl Pts',(-0.0915741794849265,0.208308207623847,
7.8592253386138));
#28653=CARTESIAN_POINT('Ctrl Pts',(0.125346722520894,0.189911450490704,
7.84811154955702));
#28654=CARTESIAN_POINT('Ctrl Pts',(0.227536379893719,-0.0023135417222602,
7.8369977605002));
#28655=CARTESIAN_POINT('Ctrl Pts',(0.121459344802718,-0.192420663711169,
7.8258839714434));
#28656=CARTESIAN_POINT('Ctrl Pts',(-0.0957906800595197,-0.206403484222046,
7.8147701823866));
#28657=CARTESIAN_POINT('Ctrl Pts',(-0.22536265898158,-0.0314618349101691,
7.80365639332978));
#28658=CARTESIAN_POINT('Ctrl Pts',(-0.148657144760437,0.172275165660006,
7.79254260427299));
#28659=CARTESIAN_POINT('Ctrl Pts',(0.0641149569483445,0.218330766034152,
7.78142881521618));
#28660=CARTESIAN_POINT('Ctrl Pts',(0.218203861216137,0.0645377811453611,
7.77031502615938));
#28661=CARTESIAN_POINT('Ctrl Pts',(0.172564429338623,-0.148311579971203,
7.75920123710257));
#28662=CARTESIAN_POINT('Ctrl Pts',(-0.0310175103799688,-0.225440983412014,
7.74808744804577));
#28663=CARTESIAN_POINT('Ctrl Pts',(-0.206223992750769,-0.0961595808285469,
7.73697365898897));
#28664=CARTESIAN_POINT('Ctrl Pts',(-0.192641054753548,0.121014476835745,
7.72585986993216));
#28665=CARTESIAN_POINT('Ctrl Pts',(-0.00279244852517366,0.227668292609634,
7.71474608087536));
#28666=CARTESIAN_POINT('Ctrl Pts',(0.189742797594757,0.125434019129486,
7.70363229181855));
#28667=CARTESIAN_POINT('Ctrl Pts',(0.2020379657277,-0.0184776408472874,
7.69622309911402));
#28668=CARTESIAN_POINT('Ctrl Pts',(0.176389912512676,-0.0771314832491572,
7.69251850276175));
#28669=CARTESIAN_POINT('Ctrl Pts',(0.156520011427165,0.133121980333227,
8.62244449171475));
#28670=CARTESIAN_POINT('Ctrl Pts',(0.20078623699224,0.081075352766993,8.61873989536248));
#28671=CARTESIAN_POINT('Ctrl Pts',(0.232520472950965,-0.0697808957830323,
8.61133070265794));
#28672=CARTESIAN_POINT('Ctrl Pts',(0.0672278516688162,-0.233526755394377,
8.60021691360114));
#28673=CARTESIAN_POINT('Ctrl Pts',(-0.159619768271145,-0.182970987722995,
8.58910312454432));
#28674=CARTESIAN_POINT('Ctrl Pts',(-0.240352188190802,0.0347903860987775,
8.57798933548754));
#28675=CARTESIAN_POINT('Ctrl Pts',(-0.101094553526346,0.220843047088143,
8.56687554643072));
#28676=CARTESIAN_POINT('Ctrl Pts',(0.130699637719291,0.204687395831059,
8.55576175737394));
#28677=CARTESIAN_POINT('Ctrl Pts',(0.242861169103291,0.00121341226084251,
8.5446479683171));
#28678=CARTESIAN_POINT('Ctrl Pts',(0.132730025418579,-0.203388545171364,
8.53353417926033));
#28679=CARTESIAN_POINT('Ctrl Pts',(-0.0988908732032454,-0.221817926612619,
8.5224203902035));
#28680=CARTESIAN_POINT('Ctrl Pts',(-0.239995603473007,-0.0372192476001651,
8.51130660114671));
#28681=CARTESIAN_POINT('Ctrl Pts',(-0.161429752413892,0.181448850846158,
8.5001928120899));
#28682=CARTESIAN_POINT('Ctrl Pts',(0.0648946403841687,0.234033639096515,
8.48907902303309));
#28683=CARTESIAN_POINT('Ctrl Pts',(0.231820203331014,0.0724053476422597,
8.4779652339763));
#28684=CARTESIAN_POINT('Ctrl Pts',(0.18655812004824,-0.155496664131617,
8.46685144491948));
#28685=CARTESIAN_POINT('Ctrl Pts',(-0.0294627337392764,-0.241070672344369,
8.45573765586269));
#28686=CARTESIAN_POINT('Ctrl Pts',(-0.218516009418034,-0.105990032544682,
8.44462386680588));
#28687=CARTESIAN_POINT('Ctrl Pts',(-0.207559105445671,0.126104522508756,
8.43351007774908));
#28688=CARTESIAN_POINT('Ctrl Pts',(-0.00662099741593451,0.242774159607174,
8.42239628869227));
#28689=CARTESIAN_POINT('Ctrl Pts',(0.200377384150519,0.13722986443753,8.41128249963547));
#28690=CARTESIAN_POINT('Ctrl Pts',(0.223968073814581,-0.0939224866161797,
8.40016871057866));
#28691=CARTESIAN_POINT('Ctrl Pts',(0.0425582454220915,-0.239106518161268,
8.38905492152186));
#28692=CARTESIAN_POINT('Ctrl Pts',(-0.177805627586376,-0.1654336431685,
8.37794113246506));
#28693=CARTESIAN_POINT('Ctrl Pts',(-0.235421993243425,0.0596625221602054,
8.36682734340825));
#28694=CARTESIAN_POINT('Ctrl Pts',(-0.0775539386019673,0.230148904034816,
8.35571355435145));
#28695=CARTESIAN_POINT('Ctrl Pts',(0.151300115555386,0.189977384132442,
8.34459976529464));
#28696=CARTESIAN_POINT('Ctrl Pts',(0.241667458088899,-0.0240825900331494,
8.33348597623784));
#28697=CARTESIAN_POINT('Ctrl Pts',(0.110833835536237,-0.216099496387572,
8.32237218718103));
#28698=CARTESIAN_POINT('Ctrl Pts',(-0.121447253622906,-0.210318082982978,
8.31125839812424));
#28699=CARTESIAN_POINT('Ctrl Pts',(-0.242566294235986,-0.012030143044946,
8.30014460906742));
#28700=CARTESIAN_POINT('Ctrl Pts',(-0.141661654845732,0.19726912324827,
8.28903082001063));
#28701=CARTESIAN_POINT('Ctrl Pts',(0.088907503777123,0.226005723850825,
8.27791703095381));
#28702=CARTESIAN_POINT('Ctrl Pts',(0.238098615913173,0.0478767223322276,
8.26680324189701));
#28703=CARTESIAN_POINT('Ctrl Pts',(0.169355364681906,-0.174074386095383,
8.2556894528402));
#28704=CARTESIAN_POINT('Ctrl Pts',(-0.0544007724631579,-0.236693234792403,
8.24457566378341));
#28705=CARTESIAN_POINT('Ctrl Pts',(-0.228363265625981,-0.0826640813999228,
8.2334618747266));
#28706=CARTESIAN_POINT('Ctrl Pts',(-0.193302271945763,0.14702844317227,
8.2223480856698));
#28707=CARTESIAN_POINT('Ctrl Pts',(0.0186904834432735,0.242144166292971,
8.21123429661299));
#28708=CARTESIAN_POINT('Ctrl Pts',(0.213575627372185,0.115622587904077,
8.20012050755619));
#28709=CARTESIAN_POINT('Ctrl Pts',(0.212972577454982,-0.11672965644274,
8.18900671849938));
#28710=CARTESIAN_POINT('Ctrl Pts',(0.0174333121199337,-0.24223792244318,
8.17789292944259));
#28711=CARTESIAN_POINT('Ctrl Pts',(-0.194062861505696,-0.146023070866488,
8.16677914038577));
#28712=CARTESIAN_POINT('Ctrl Pts',(-0.227931097172626,0.0838483534885532,
8.15566535132898));
#28713=CARTESIAN_POINT('Ctrl Pts',(-0.0531714146829997,0.236972428990521,
8.14455156227216));
#28714=CARTESIAN_POINT('Ctrl Pts',(0.170256666670833,0.173192952787333,
8.13343777321537));
#28715=CARTESIAN_POINT('Ctrl Pts',(0.237846890178926,-0.0491119972437703,
8.12232398415856));
#28716=CARTESIAN_POINT('Ctrl Pts',(0.0877331577390571,-0.22646417922973,
8.11121019510175));
#28717=CARTESIAN_POINT('Ctrl Pts',(-0.142683728941055,-0.196531129688227,
8.10009640604495));
#28718=CARTESIAN_POINT('Ctrl Pts',(-0.242500580377868,0.0132890916714718,
8.08898261698815));
#28719=CARTESIAN_POINT('Ctrl Pts',(-0.120353900451207,0.210945656715802,
8.07786882793134));
#28720=CARTESIAN_POINT('Ctrl Pts',(0.111954069464546,0.215521269881544,
8.06675503887454));
#28721=CARTESIAN_POINT('Ctrl Pts',(0.241789209953822,0.0228278205475825,
8.05564124981773));
#28722=CARTESIAN_POINT('Ctrl Pts',(0.150311944496376,-0.190760191819292,
8.04452746076093));
#28723=CARTESIAN_POINT('Ctrl Pts',(-0.0787475484122947,-0.229743237245029,
8.03341367170412));
#28724=CARTESIAN_POINT('Ctrl Pts',(-0.235728517200657,-0.0584396921573019,
8.02229988264732));
#28725=CARTESIAN_POINT('Ctrl Pts',(-0.176944500853229,0.166354365918009,
8.01118609359052));
#28726=CARTESIAN_POINT('Ctrl Pts',(0.043798823814624,0.238882386272181,
8.00007230453372));
#28727=CARTESIAN_POINT('Ctrl Pts',(0.224452588327861,0.0927586493798742,
7.98895851547691));
#28728=CARTESIAN_POINT('Ctrl Pts',(0.199662353288342,-0.138268131282085,
7.9778447264201));
#28729=CARTESIAN_POINT('Ctrl Pts',(-0.00788109805936929,-0.242736523239671,
7.96673093736331));
#28730=CARTESIAN_POINT('Ctrl Pts',(-0.20821089093935,-0.12502542280459,
7.95561714830649));
#28731=CARTESIAN_POINT('Ctrl Pts',(-0.217962894142359,0.107122865301834,
7.9445033592497));
#28732=CARTESIAN_POINT('Ctrl Pts',(-0.0282109883268786,0.241220379359275,
7.93338957019289));
#28733=CARTESIAN_POINT('Ctrl Pts',(0.187362754755622,0.154526145718984,
7.92227578113608));
#28734=CARTESIAN_POINT('Ctrl Pts',(0.23144124413335,-0.0736076238344533,
7.91116199207928));
#28735=CARTESIAN_POINT('Ctrl Pts',(0.0636789369204538,-0.234367495981061,
7.90004820302247));
#28736=CARTESIAN_POINT('Ctrl Pts',(-0.162369421216092,-0.180608150160837,
7.88893441396567));
#28737=CARTESIAN_POINT('Ctrl Pts',(-0.239799211098419,0.0384639016141247,
7.87782062490887));
#28738=CARTESIAN_POINT('Ctrl Pts',(-0.0977380548679695,0.222329472572989,
7.86670683585206));
#28739=CARTESIAN_POINT('Ctrl Pts',(0.133783834178758,0.2026944262293,7.85559304679526));
#28740=CARTESIAN_POINT('Ctrl Pts',(0.242851896763891,-0.00246926665421919,
7.84447925773846));
#28741=CARTESIAN_POINT('Ctrl Pts',(0.129634796329349,-0.205372535067366,
7.83336546868165));
#28742=CARTESIAN_POINT('Ctrl Pts',(-0.102238368895662,-0.220296541877889,
7.82225167962484));
#28743=CARTESIAN_POINT('Ctrl Pts',(-0.240531862285032,-0.033579536982947,
7.81113789056804));
#28744=CARTESIAN_POINT('Ctrl Pts',(-0.158663285358761,0.183871039722915,
7.80002410151124));
#28745=CARTESIAN_POINT('Ctrl Pts',(0.0684305468563471,0.233026651290108,
7.78891031245443));
#28746=CARTESIAN_POINT('Ctrl Pts',(0.232891204484732,0.0688818314302299,
7.77779652339763));
#28747=CARTESIAN_POINT('Ctrl Pts',(0.184179773794582,-0.158294460538047,
7.76668273434082));
#28748=CARTESIAN_POINT('Ctrl Pts',(-0.0331053048843776,-0.240615458747729,
7.75556894528403));
#28749=CARTESIAN_POINT('Ctrl Pts',(-0.22010496880165,-0.102632100445394,
7.74445515622721));
#28750=CARTESIAN_POINT('Ctrl Pts',(-0.205607760672592,0.129159984215175,
7.73334136717041));
#28751=CARTESIAN_POINT('Ctrl Pts',(-0.00298040876483471,0.242992688549725,
7.7222275781136));
#28752=CARTESIAN_POINT('Ctrl Pts',(0.202514421274951,0.133877006738626,
7.7111137890568));
#28753=CARTESIAN_POINT('Ctrl Pts',(0.215637179506012,-0.0197213743559677,
7.70370459635227));
#28754=CARTESIAN_POINT('Ctrl Pts',(0.188262750966369,-0.0823232180103224,
7.7));
#28755=CARTESIAN_POINT('Ctrl Pts',(0.126907087985233,0.107935865304858,
8.6));
#28756=CARTESIAN_POINT('Ctrl Pts',(0.135119342222632,0.100274703694019,
8.6));
#28757=CARTESIAN_POINT('Ctrl Pts',(0.142437014324932,0.0917732077732832,
8.6));
#28758=CARTESIAN_POINT('Ctrl Pts',(0.14885561179134,0.0826255492913934,
8.6));
#28759=CARTESIAN_POINT('Ctrl Pts',(0.153626284694708,0.0758264803861984,
8.6));
#28760=CARTESIAN_POINT('Ctrl Pts',(0.157899939952193,0.0686691570742025,
8.6));
#28761=CARTESIAN_POINT('Ctrl Pts',(0.161664554366084,0.0612188846220726,
8.6));
#28762=CARTESIAN_POINT('Ctrl Pts',(0.163881899847797,0.0568306987036657,
8.6));
#28763=CARTESIAN_POINT('Ctrl Pts',(0.165924040766234,0.0523356709836805,
8.6));
#28764=CARTESIAN_POINT('Ctrl Pts',(0.167776061733539,0.0477755770655923,
8.6));
#28765=CARTESIAN_POINT('Ctrl Pts',(0.172334880242679,0.0365507362434885,
8.6));
#28766=CARTESIAN_POINT('Ctrl Pts',(0.175760680768791,0.0249077723450597,
8.6));
#28767=CARTESIAN_POINT('Ctrl Pts',(0.178025304432692,0.0130451206803074,
8.6));
#28768=CARTESIAN_POINT('Ctrl Pts',(0.179464454318053,0.00550650220893073,
8.6));
#28769=CARTESIAN_POINT('Ctrl Pts',(0.180433932781852,-0.002121718043742,
8.6));
#28770=CARTESIAN_POINT('Ctrl Pts',(0.180916947576875,-0.00979373217332476,
8.6));
#28771=CARTESIAN_POINT('Ctrl Pts',(0.181142367724244,-0.0133742157807179,
8.6));
#28772=CARTESIAN_POINT('Ctrl Pts',(0.181261291825179,-0.0169607842651116,
8.6));
#28773=CARTESIAN_POINT('Ctrl Pts',(0.181272571985224,-0.0205386416225958,
8.6));
#28774=CARTESIAN_POINT('Ctrl Pts',(0.181307739490319,-0.0316931213770327,
8.6));
#28775=CARTESIAN_POINT('Ctrl Pts',(0.18030100776568,-0.0427900713202343,
8.6));
#28776=CARTESIAN_POINT('Ctrl Pts',(0.178218613078485,-0.0536884200006557,
8.6));
#28777=CARTESIAN_POINT('Ctrl Pts',(0.177058261266385,-0.0597611970385473,
8.6));
#28778=CARTESIAN_POINT('Ctrl Pts',(0.175563380683853,-0.0657725480180776,
8.6));
#28779=CARTESIAN_POINT('Ctrl Pts',(0.173752707611816,-0.0717063254815672,
8.6));
#28780=CARTESIAN_POINT('Ctrl Pts',(0.172620016542247,-0.0754182803592885,
8.6));
#28781=CARTESIAN_POINT('Ctrl Pts',(0.171363093867741,-0.0791013962971504,
8.6));
#28782=CARTESIAN_POINT('Ctrl Pts',(0.169987642094878,-0.0827468570145976,
8.6));
#28783=CARTESIAN_POINT('Ctrl Pts',(0.165605788263354,-0.094360405615556,
8.6));
#28784=CARTESIAN_POINT('Ctrl Pts',(0.160056570352909,-0.10551119017211,
8.6));
#28785=CARTESIAN_POINT('Ctrl Pts',(0.153505449982331,-0.116076623215971,
8.6));
#28786=CARTESIAN_POINT('Ctrl Pts',(0.14916461185782,-0.123077385217648,
8.6));
#28787=CARTESIAN_POINT('Ctrl Pts',(0.144382694364319,-0.129821293390769,
8.6));
#28788=CARTESIAN_POINT('Ctrl Pts',(0.139196287888346,-0.136270468973621,
8.6));
#28789=CARTESIAN_POINT('Ctrl Pts',(0.136485946091972,-0.139640715832468,
8.6));
#28790=CARTESIAN_POINT('Ctrl Pts',(0.133663744041843,-0.142931788522251,
8.6));
#28791=CARTESIAN_POINT('Ctrl Pts',(0.130738055024136,-0.146133486419774,
8.6));
#28792=CARTESIAN_POINT('Ctrl Pts',(0.124471671826875,-0.15299103887539,
8.6));
#28793=CARTESIAN_POINT('Ctrl Pts',(0.117755782354928,-0.159412890827526,
8.6));
#28794=CARTESIAN_POINT('Ctrl Pts',(0.110644485105481,-0.165348276025604,
8.6));
#28795=CARTESIAN_POINT('Ctrl Pts',(0.106128056396711,-0.169117875743616,
8.6));
#28796=CARTESIAN_POINT('Ctrl Pts',(0.101451886306371,-0.172691180761178,
8.6));
#28797=CARTESIAN_POINT('Ctrl Pts',(0.0966276544344934,-0.176053779769394,
8.6));
#28798=CARTESIAN_POINT('Ctrl Pts',(0.0925453919559805,-0.178899209285654,
8.6));
#28799=CARTESIAN_POINT('Ctrl Pts',(0.0883640473887971,-0.181588757784238,
8.6));
#28800=CARTESIAN_POINT('Ctrl Pts',(0.0840946504162302,-0.184112638937655,
8.6));
#28801=CARTESIAN_POINT('Ctrl Pts',(0.0753694926585074,-0.189270571396691,
8.6));
#28802=CARTESIAN_POINT('Ctrl Pts',(0.0662731702050655,-0.193740352082781,
8.6));
#28803=CARTESIAN_POINT('Ctrl Pts',(0.0568645195540229,-0.197448127710951,
8.6));
#28804=CARTESIAN_POINT('Ctrl Pts',(0.0556251889131679,-0.197936525050361,
8.6));
#28805=CARTESIAN_POINT('Ctrl Pts',(0.0543804239234686,-0.19841168092438,
8.6));
#28806=CARTESIAN_POINT('Ctrl Pts',(0.0531304158592269,-0.198873653475084,
8.6));
#28807=CARTESIAN_POINT('Ctrl Pts',(-0.166732044643443,-0.000130047968060085,
8.48714803633902));
#28808=CARTESIAN_POINT('Ctrl Pts',(-0.166805196659206,-0.00865458859339771,
8.48771939403667));
#28809=CARTESIAN_POINT('Ctrl Pts',(-0.166207891524911,-0.0171688432130046,
8.48829075173431));
#28810=CARTESIAN_POINT('Ctrl Pts',(-0.164904478551508,-0.0255735852889172,
8.48886210943196));
#28811=CARTESIAN_POINT('Ctrl Pts',(-0.156453347208284,-0.0800686537276021,
8.49256670578422));
#28812=CARTESIAN_POINT('Ctrl Pts',(-0.118317242957253,-0.129959783911282,
8.49627130213649));
#28813=CARTESIAN_POINT('Ctrl Pts',(-0.0679493232806182,-0.152414912252412,
8.49997589848876));
#28814=CARTESIAN_POINT('Ctrl Pts',(-0.0175814036039843,-0.174870040593541,
8.50368049484103));
#28815=CARTESIAN_POINT('Ctrl Pts',(0.045018331498252,-0.169889167092121,
8.5073850911933));
#28816=CARTESIAN_POINT('Ctrl Pts',(0.0912006653168583,-0.139750041443162,
8.51108968754557));
#28817=CARTESIAN_POINT('Ctrl Pts',(0.137382999135465,-0.109610915794204,
8.51479428389784));
#28818=CARTESIAN_POINT('Ctrl Pts',(0.167147931670441,-0.054313537997707,
8.5184988802501));
#28819=CARTESIAN_POINT('Ctrl Pts',(0.16687355717987,0.000831412134915374,
8.52220347660237));
#28820=CARTESIAN_POINT('Ctrl Pts',(0.166599182689298,0.0559763622675381,
8.52590807295464));
#28821=CARTESIAN_POINT('Ctrl Pts',(0.136285501173178,0.110968884736286,
8.52961266930691));
#28822=CARTESIAN_POINT('Ctrl Pts',(0.0898053751318118,0.140648324377953,
8.53331726565918));
#28823=CARTESIAN_POINT('Ctrl Pts',(0.0433252490904463,0.170327764019619,
8.53702186201145));
#28824=CARTESIAN_POINT('Ctrl Pts',(-0.0193213214761645,0.174694120834203,
8.54072645836371));
#28825=CARTESIAN_POINT('Ctrl Pts',(-0.0694630533953934,0.15173525169246,
8.54443105471598));
#28826=CARTESIAN_POINT('Ctrl Pts',(-0.119604785314622,0.128776382550717,
8.54813565106824));
#28827=CARTESIAN_POINT('Ctrl Pts',(-0.157241678586469,0.078492287452646,
8.55184024742051));
#28828=CARTESIAN_POINT('Ctrl Pts',(-0.165150427239171,0.023923265917556,
8.55554484377278));
#28829=CARTESIAN_POINT('Ctrl Pts',(-0.166291284509671,0.0160515446508695,
8.55607924129486));
#28830=CARTESIAN_POINT('Ctrl Pts',(-0.166813534699148,0.00809065919753236,
8.55661363881694));
#28831=CARTESIAN_POINT('Ctrl Pts',(-0.166747144031447,0.000121296159821427,
8.55714803633902));
#28832=CARTESIAN_POINT('Ctrl Pts',(-0.0530170217188485,-0.198517432567176,
8.6));
#28833=CARTESIAN_POINT('Ctrl Pts',(-0.119028790974543,-0.180888011517996,
8.59629540364773));
#28834=CARTESIAN_POINT('Ctrl Pts',(-0.230934959138857,-0.074861353976339,
8.5888862109432));
#28835=CARTESIAN_POINT('Ctrl Pts',(-0.188121058383465,0.153833707952583,
8.57777242188639));
#28836=CARTESIAN_POINT('Ctrl Pts',(0.027212997215315,0.241280498724425,
8.56665863282958));
#28837=CARTESIAN_POINT('Ctrl Pts',(0.217474198098902,0.108094945242369,
8.5555448437728));
#28838=CARTESIAN_POINT('Ctrl Pts',(0.208761552554325,-0.124138522922833,
8.54443105471596));
#28839=CARTESIAN_POINT('Ctrl Pts',(0.00892537992430322,-0.24269250748312,
8.53331726565919));
#28840=CARTESIAN_POINT('Ctrl Pts',(-0.199059264243693,-0.139134553701345,
8.52220347660236));
#28841=CARTESIAN_POINT('Ctrl Pts',(-0.22485330991897,0.0917885826081383,
8.51108968754558));
#28842=CARTESIAN_POINT('Ctrl Pts',(-0.0448312245259985,0.238689656539759,
8.49997589848875));
#28843=CARTESIAN_POINT('Ctrl Pts',(0.176222693303572,0.167118876029215,
8.48886210943197));
#28844=CARTESIAN_POINT('Ctrl Pts',(0.235979340716847,-0.0574194692648986,
8.47774832037514));
#28845=CARTESIAN_POINT('Ctrl Pts',(0.0797407360187229,-0.229400234578822,
8.46663453131836));
#28846=CARTESIAN_POINT('Ctrl Pts',(-0.149485123105517,-0.191408811645189,
8.45552074226153));
#28847=CARTESIAN_POINT('Ctrl Pts',(-0.241885728018762,0.0217814932194586,
8.44440695320475));
#28848=CARTESIAN_POINT('Ctrl Pts',(-0.112885495048793,0.215034836414334,
8.43329316414793));
#28849=CARTESIAN_POINT('Ctrl Pts',(0.119440067448933,0.211464412612195,
8.42217937509113));
#28850=CARTESIAN_POINT('Ctrl Pts',(0.242440804004482,0.0143381848173731,
8.41106558603433));
#28851=CARTESIAN_POINT('Ctrl Pts',(0.143532711926644,-0.195911931545135,
8.39995179697752));
#28852=CARTESIAN_POINT('Ctrl Pts',(-0.0867524934706339,-0.226841642534413,
8.38883800792072));
#28853=CARTESIAN_POINT('Ctrl Pts',(-0.23763216061734,-0.0501406218404715,
8.37772421886392));
#28854=CARTESIAN_POINT('Ctrl Pts',(-0.17100441477528,0.172454676785586,
8.36661042980711));
#28855=CARTESIAN_POINT('Ctrl Pts',(0.05214561050461,0.237200254924533,8.35549664075031));
#28856=CARTESIAN_POINT('Ctrl Pts',(0.22756616748523,0.0848337492213278,
8.3443828516935));
#28857=CARTESIAN_POINT('Ctrl Pts',(0.19469283040568,-0.145182048984365,
8.3332690626367));
#28858=CARTESIAN_POINT('Ctrl Pts',(-0.016385062217743,-0.242311071399234,
8.3221552735799));
#28859=CARTESIAN_POINT('Ctrl Pts',(-0.212465521621073,-0.117650022106929,
8.31104148452309));
#28860=CARTESIAN_POINT('Ctrl Pts',(-0.214073879538015,0.114697426631087,
8.29992769546629));
#28861=CARTESIAN_POINT('Ctrl Pts',(-0.0197379877628579,0.242061020031891,
8.28881390640948));
#28862=CARTESIAN_POINT('Ctrl Pts',(0.19266430806168,0.147863416631009,8.27770011735268));
#28863=CARTESIAN_POINT('Ctrl Pts',(0.22871877775246,-0.0816752488934883,
8.26658632829587));
#28864=CARTESIAN_POINT('Ctrl Pts',(0.0554243563205898,-0.236455632847443,
8.25547253923908));
#28865=CARTESIAN_POINT('Ctrl Pts',(-0.168600607007242,-0.174805494465869,
8.24435875018226));
#28866=CARTESIAN_POINT('Ctrl Pts',(-0.238303522680024,0.0468460954289506,
8.23324496112547));
#28867=CARTESIAN_POINT('Ctrl Pts',(-0.0898845214982184,0.22561892290705,
8.22213117206865));
#28868=CARTESIAN_POINT('Ctrl Pts',(0.14080680157081,0.197880191555585,8.21101738301186));
#28869=CARTESIAN_POINT('Ctrl Pts',(0.242616062304287,-0.0109805232406446,
8.19990359395504));
#28870=CARTESIAN_POINT('Ctrl Pts',(0.122356089757392,-0.209790640587143,
8.18878980489824));
#28871=CARTESIAN_POINT('Ctrl Pts',(-0.109897799356892,-0.21657700541653,
8.17767601584145));
#28872=CARTESIAN_POINT('Ctrl Pts',(-0.241560986393994,-0.0251279810378811,
8.16656222678462));
#28873=CARTESIAN_POINT('Ctrl Pts',(-0.152120663096767,0.189320969355431,
8.15544843772784));
#28874=CARTESIAN_POINT('Ctrl Pts',(0.0765574282985869,0.230482289451893,
8.14433464867103));
#28875=CARTESIAN_POINT('Ctrl Pts',(0.235161637351955,0.0606805561660993,
8.13322085961422));
#28876=CARTESIAN_POINT('Ctrl Pts',(0.178519732822726,-0.164662778342839,
8.12210707055743));
#28877=CARTESIAN_POINT('Ctrl Pts',(-0.0415233077106159,-0.239288404431658,
8.1109932815006));
#28878=CARTESIAN_POINT('Ctrl Pts',(-0.223559593790088,-0.0948906402291072,
8.09987949244382));
#28879=CARTESIAN_POINT('Ctrl Pts',(-0.200969248335269,0.136361603108205,
8.088765703387));
#28880=CARTESIAN_POINT('Ctrl Pts',(0.00557052926712743,0.242800524674804,
8.0776519143302));
#28881=CARTESIAN_POINT('Ctrl Pts',(0.207011538257192,0.127001372461354,
8.06653812527341));
#28882=CARTESIAN_POINT('Ctrl Pts',(0.218972538609993,-0.105043576259552,
8.05542433621658));
#28883=CARTESIAN_POINT('Ctrl Pts',(0.0305054910554562,-0.240940948354804,
8.0443105471598));
#28884=CARTESIAN_POINT('Ctrl Pts',(-0.185883578417697,-0.156302337964917,
8.03319675810297));
#28885=CARTESIAN_POINT('Ctrl Pts',(-0.232131300502452,0.0714015749537549,
8.02208296904619));
#28886=CARTESIAN_POINT('Ctrl Pts',(-0.0659066106883685,0.233750816567481,
8.01096917998937));
#28887=CARTESIAN_POINT('Ctrl Pts',(0.160643147318701,0.182145284864098,
7.99985539093258));
#28888=CARTESIAN_POINT('Ctrl Pts',(0.240154410771491,-0.0361798917467206,
7.98874160187577));
#28889=CARTESIAN_POINT('Ctrl Pts',(0.0998496185014871,-0.221389203127338,
7.97762781281897));
#28890=CARTESIAN_POINT('Ctrl Pts',(-0.13184866193996,-0.203958466174165,
7.96651402376217));
#28891=CARTESIAN_POINT('Ctrl Pts',(-0.242864366871307,0.000157767940311883,
7.95540023470535));
#28892=CARTESIAN_POINT('Ctrl Pts',(-0.131583562478442,0.204129595218713,
7.94428644564855));
#28893=CARTESIAN_POINT('Ctrl Pts',(0.100137168795687,0.221259289107705,
7.93317265659175));
#28894=CARTESIAN_POINT('Ctrl Pts',(0.240201214065173,0.035867846224428,
7.92205886753494));
#28895=CARTESIAN_POINT('Ctrl Pts',(0.160406363583993,-0.182353842678505,
7.91094507847815));
#28896=CARTESIAN_POINT('Ctrl Pts',(-0.0662102497254891,-0.233664992135114,
7.89983128942133));
#28897=CARTESIAN_POINT('Ctrl Pts',(-0.232223872355038,-0.0710999227813469,
7.88871750036453));
#28898=CARTESIAN_POINT('Ctrl Pts',(-0.185680347511564,0.156543709112656,
7.87760371130772));
#28899=CARTESIAN_POINT('Ctrl Pts',(0.0308184982090563,0.240901114896414,
7.86648992225093));
#28900=CARTESIAN_POINT('Ctrl Pts',(0.21910883681408,0.104758985980235,7.85537613319412));
#28901=CARTESIAN_POINT('Ctrl Pts',(0.206846344849442,-0.12727020659438,
7.84426234413731));
#28902=CARTESIAN_POINT('Ctrl Pts',(0.00525510193017616,-0.242807583839013,
7.83314855508051));
#28903=CARTESIAN_POINT('Ctrl Pts',(-0.201146303040926,-0.136100330558978,
7.82203476602371));
#28904=CARTESIAN_POINT('Ctrl Pts',(-0.223436002168958,0.0951809095374688,
7.8109209769669));
#28905=CARTESIAN_POINT('Ctrl Pts',(-0.0412126180342513,0.239342358997698,
7.7998071879101));
#28906=CARTESIAN_POINT('Ctrl Pts',(0.178733982604362,0.164430288641772,
7.7886933988533));
#28907=CARTESIAN_POINT('Ctrl Pts',(0.23508167636479,-0.0609852135282689,
7.77757960979648));
#28908=CARTESIAN_POINT('Ctrl Pts',(0.0762597491160078,-0.230583185734543,
7.76646582073969));
#28909=CARTESIAN_POINT('Ctrl Pts',(-0.152370142836843,-0.189119946824214,
7.75535203168288));
#28910=CARTESIAN_POINT('Ctrl Pts',(-0.2415209216033,0.0254354088453453,
7.74423824262608));
#28911=CARTESIAN_POINT('Ctrl Pts',(-0.109630632113431,0.216732284629596,
7.73312445356927));
#28912=CARTESIAN_POINT('Ctrl Pts',(0.122656937311001,0.209606344739839,
7.72201066451247));
#28913=CARTESIAN_POINT('Ctrl Pts',(0.242573721631839,0.0107152160886697,
7.71089687545566));
#28914=CARTESIAN_POINT('Ctrl Pts',(0.140662758040614,-0.198162384952754,
7.69978308639886));
#28915=CARTESIAN_POINT('Ctrl Pts',(-0.0904173958729584,-0.225299516633279,
7.68866929734205));
#28916=CARTESIAN_POINT('Ctrl Pts',(-0.188575434363685,-0.106431345694509,
7.68126010463752));
#28917=CARTESIAN_POINT('Ctrl Pts',(-0.201667586144655,-0.0393720754290152,
7.67755550828525));
#28918=CARTESIAN_POINT('Ctrl Pts',(-0.0496734897087577,-0.18599788000028,
8.60748149723825));
#28919=CARTESIAN_POINT('Ctrl Pts',(-0.111522209883356,-0.169480262890407,
8.60377690088598));
#28920=CARTESIAN_POINT('Ctrl Pts',(-0.216370986982434,-0.0701402035755114,
8.59636770818144));
#28921=CARTESIAN_POINT('Ctrl Pts',(-0.176257155808688,0.144132145886385,
8.58525391912465));
#28922=CARTESIAN_POINT('Ctrl Pts',(0.025496802598378,0.226064082472793,
8.57414013006782));
#28923=CARTESIAN_POINT('Ctrl Pts',(0.203759132274033,0.101277909923722,
8.56302634101104));
#28924=CARTESIAN_POINT('Ctrl Pts',(0.195595951945087,-0.116309695281798,
8.55191255195423));
#28925=CARTESIAN_POINT('Ctrl Pts',(0.00836249856070296,-0.227387042538631,
8.54079876289741));
#28926=CARTESIAN_POINT('Ctrl Pts',(-0.186505540923786,-0.130359997550735,
8.52968497384063));
#28927=CARTESIAN_POINT('Ctrl Pts',(-0.21067287852326,0.085999912212078,
8.5185711847838));
#28928=CARTESIAN_POINT('Ctrl Pts',(-0.0420039319057314,0.223636632411953,
8.50745739572702));
#28929=CARTESIAN_POINT('Ctrl Pts',(0.165109164160243,0.156579481446523,
8.49634360667019));
#28930=CARTESIAN_POINT('Ctrl Pts',(0.221097243348363,-0.053798295776359,
8.48522981761341));
#28931=CARTESIAN_POINT('Ctrl Pts',(0.0747118661436728,-0.214933050218597,
8.4741160285566));
#28932=CARTESIAN_POINT('Ctrl Pts',(-0.140057805652904,-0.179337566071589,
8.46300223949979));
#28933=CARTESIAN_POINT('Ctrl Pts',(-0.226631142827166,0.0204078377886982,
8.45188845044299));
#28934=CARTESIAN_POINT('Ctrl Pts',(-0.105766342483563,0.201473609556878,
8.44077466138618));
#28935=CARTESIAN_POINT('Ctrl Pts',(0.111907549101888,0.19812835544336,8.42966087232938));
#28936=CARTESIAN_POINT('Ctrl Pts',(0.227151212804134,0.0134339435312874,
8.41854708327257));
#28937=CARTESIAN_POINT('Ctrl Pts',(0.134480784804694,-0.183556695565385,
8.40743329421579));
#28938=CARTESIAN_POINT('Ctrl Pts',(-0.0812814253217577,-0.212535816434684,
8.39631950515895));
#28939=CARTESIAN_POINT('Ctrl Pts',(-0.222645827739863,-0.0469784907230634,
8.38520571610218));
#28940=CARTESIAN_POINT('Ctrl Pts',(-0.160219977699579,0.16157877856595,
8.37409192704536));
#28941=CARTESIAN_POINT('Ctrl Pts',(0.0488570342652188,0.22224116028984,
8.36297813798856));
#28942=CARTESIAN_POINT('Ctrl Pts',(0.213214649034505,0.0794836871683949,
8.35186434893175));
#28943=CARTESIAN_POINT('Ctrl Pts',(0.182414477350531,-0.136026105999789,
8.34075055987495));
#28944=CARTESIAN_POINT('Ctrl Pts',(-0.0153517340858297,-0.227029661818758,
8.32963677081815));
#28945=CARTESIAN_POINT('Ctrl Pts',(-0.199066329257008,-0.110230393426381,
8.31852298176133));
#28946=CARTESIAN_POINT('Ctrl Pts',(-0.200573255671299,0.107464004138028,
8.30740919270455));
#28947=CARTESIAN_POINT('Ctrl Pts',(-0.0184932065254304,0.226795380004735,
8.29629540364772));
#28948=CARTESIAN_POINT('Ctrl Pts',(0.180513884286042,0.138538372511237,
8.28518161459093));
#28949=CARTESIAN_POINT('Ctrl Pts',(0.214294569640967,-0.0765243784701043,
8.27406782553412));
#28950=CARTESIAN_POINT('Ctrl Pts',(0.0519290051392408,-0.221543497994145,
8.26295403647732));
#28951=CARTESIAN_POINT('Ctrl Pts',(-0.157967766682131,-0.163781341329055,
8.25184024742051));
#28952=CARTESIAN_POINT('Ctrl Pts',(-0.223274850182662,0.0438917344607866,
8.24072645836371));
#28953=CARTESIAN_POINT('Ctrl Pts',(-0.0842159312021673,0.211390207932784,
8.22961266930691));
#28954=CARTESIAN_POINT('Ctrl Pts',(0.131926784681382,0.185400826755775,
8.21849888025009));
#28955=CARTESIAN_POINT('Ctrl Pts',(0.227315418394518,-0.0102880337391155,
8.20738509119331));
#28956=CARTESIAN_POINT('Ctrl Pts',(0.114639671718996,-0.196560140278386,
8.19627130213649));
#28957=CARTESIAN_POINT('Ctrl Pts',(-0.102967066583239,-0.20291852127723,
8.18515751307969));
#28958=CARTESIAN_POINT('Ctrl Pts',(-0.226326881115871,-0.0235432784984843,
8.17404372402289));
#28959=CARTESIAN_POINT('Ctrl Pts',(-0.142527134641746,0.177381394088866,
8.16292993496608));
#28960=CARTESIAN_POINT('Ctrl Pts',(0.0717293145376143,0.215946865024847,
8.15181614590928));
#28961=CARTESIAN_POINT('Ctrl Pts',(0.22033110865494,0.0568537213995711,
8.14070235685247));
#28962=CARTESIAN_POINT('Ctrl Pts',(0.167261340295681,-0.154278278187787,
8.12958856779567));
#28963=CARTESIAN_POINT('Ctrl Pts',(-0.038904629708831,-0.224197620115187,
8.11847477873885));
#28964=CARTESIAN_POINT('Ctrl Pts',(-0.209460750932336,-0.0889063377772168,
8.10736098968207));
#28965=CARTESIAN_POINT('Ctrl Pts',(-0.188295071381003,0.127761923794693,
8.09624720062525));
#28966=CARTESIAN_POINT('Ctrl Pts',(0.00521922241672461,0.227488247598545,
8.08513341156845));
#28967=CARTESIAN_POINT('Ctrl Pts',(0.193956302746387,0.118991998483278,
8.07401962251165));
#28968=CARTESIAN_POINT('Ctrl Pts',(0.205162979558262,-0.0984189763048294,
8.06290583345485));
#28969=CARTESIAN_POINT('Ctrl Pts',(0.0285816544739079,-0.225745945933921,
8.05179204439804));
#28970=CARTESIAN_POINT('Ctrl Pts',(-0.174160783088195,-0.146445091116742,
8.04067825534124));
#28971=CARTESIAN_POINT('Ctrl Pts',(-0.217491880772505,0.0668986164002777,
8.02956446628442));
#28972=CARTESIAN_POINT('Ctrl Pts',(-0.0617501934591672,0.219009261643426,
8.01845067722763));
#28973=CARTESIAN_POINT('Ctrl Pts',(0.150512146220409,0.170658245971951,
8.00733688817082));
#28974=CARTESIAN_POINT('Ctrl Pts',(0.225009011544104,-0.0338981976368876,
7.99622309911402));
#28975=CARTESIAN_POINT('Ctrl Pts',(0.0935525768188083,-0.207427236510839,
7.98510931005721));
#28976=CARTESIAN_POINT('Ctrl Pts',(-0.12353359241339,-0.191095773433733,
7.97399552100042));
#28977=CARTESIAN_POINT('Ctrl Pts',(-0.227548063570627,0.000147818264877529,
7.9628817319436));
#28978=CARTESIAN_POINT('Ctrl Pts',(-0.123285211517094,0.191256110181397,
7.95176794288681));
#28979=CARTESIAN_POINT('Ctrl Pts',(0.0938219926802922,0.207305515552022,
7.94065415382999));
#28980=CARTESIAN_POINT('Ctrl Pts',(0.225052863176122,0.0336058313451245,
7.9295403647732));
#28981=CARTESIAN_POINT('Ctrl Pts',(0.150290295312382,-0.170853651034546,
7.91842657571639));
#28982=CARTESIAN_POINT('Ctrl Pts',(-0.0620346834228921,-0.218928849750797,
7.90731278665959));
#28983=CARTESIAN_POINT('Ctrl Pts',(-0.217578614557574,-0.0666159879991351,
7.89619899760278));
#28984=CARTESIAN_POINT('Ctrl Pts',(-0.173970368991043,0.146671240131426,
7.88508520854598));
#28985=CARTESIAN_POINT('Ctrl Pts',(0.0288749217514545,0.225708624582753,
7.87397141948917));
#28986=CARTESIAN_POINT('Ctrl Pts',(0.205290682081311,0.0981523337841342,
7.86285763043236));
#28987=CARTESIAN_POINT('Ctrl Pts',(0.19380152730307,-0.119243878523071,
7.85174384137556));
#28988=CARTESIAN_POINT('Ctrl Pts',(0.00492368758530773,-0.227494861574761,
7.84063005231876));
#28989=CARTESIAN_POINT('Ctrl Pts',(-0.188460960086445,-0.127517128465487,
7.82951626326196));
#28990=CARTESIAN_POINT('Ctrl Pts',(-0.209344953648346,0.08917830117754,
7.81840247420515));
#28991=CARTESIAN_POINT('Ctrl Pts',(-0.0386135337562265,0.224248172022745,
7.80728868514835));
#28992=CARTESIAN_POINT('Ctrl Pts',(0.16746207836014,0.154060450509073,7.79617489609154));
#28993=CARTESIAN_POINT('Ctrl Pts',(0.220256190427845,-0.0571391654674155,
7.78506110703474));
#28994=CARTESIAN_POINT('Ctrl Pts',(0.071450408568683,-0.216041398257672,
7.77394731797793));
#28995=CARTESIAN_POINT('Ctrl Pts',(-0.14276088087832,-0.177193049094902,
7.76283352892113));
#28996=CARTESIAN_POINT('Ctrl Pts',(-0.226289343021431,0.0238313182927837,
7.75171973986433));
#28997=CARTESIAN_POINT('Ctrl Pts',(-0.102716748310195,0.203064007767081,
7.74060595080752));
#28998=CARTESIAN_POINT('Ctrl Pts',(0.114921546244829,0.196387467095744,
7.72949216175072));
#28999=CARTESIAN_POINT('Ctrl Pts',(0.227275747947388,0.0100394582504136,
7.71837837269392));
#29000=CARTESIAN_POINT('Ctrl Pts',(0.131791825293193,-0.185665223554306,
7.70726458363711));
#29001=CARTESIAN_POINT('Ctrl Pts',(-0.0847151997184201,-0.211090945097214,
7.69615079458031));
#29002=CARTESIAN_POINT('Ctrl Pts',(-0.176682876451711,-0.0997192257060688,
7.68874160187577));
#29003=CARTESIAN_POINT('Ctrl Pts',(-0.188949368338152,-0.0368890654402851,
7.6850370055235));
#29004=CARTESIAN_POINT('Ctrl Pts',(-0.0463299576986669,-0.173478327433383,
8.6149629944765));
#29005=CARTESIAN_POINT('Ctrl Pts',(-0.104015628792168,-0.158072514262817,
8.61125839812423));
#29006=CARTESIAN_POINT('Ctrl Pts',(-0.201807014826011,-0.0654190531746837,
8.60384920541969));
#29007=CARTESIAN_POINT('Ctrl Pts',(-0.16439325323391,0.134430583820185,
8.5927354163629));
#29008=CARTESIAN_POINT('Ctrl Pts',(0.0237806079814409,0.210847666221162,
8.58162162730608));
#29009=CARTESIAN_POINT('Ctrl Pts',(0.190044066449164,0.0944608746050748,
8.57050783824928));
#29010=CARTESIAN_POINT('Ctrl Pts',(0.182430351335849,-0.108480867640763,
8.55939404919248));
#29011=CARTESIAN_POINT('Ctrl Pts',(0.00779961719710285,-0.212081577594143,
8.54828026013567));
#29012=CARTESIAN_POINT('Ctrl Pts',(-0.173951817603879,-0.121585441400125,
8.53716647107887));
#29013=CARTESIAN_POINT('Ctrl Pts',(-0.196492447127551,0.080211241816018,
8.52605268202207));
#29014=CARTESIAN_POINT('Ctrl Pts',(-0.0391766392854642,0.208583608284146,
8.51493889296525));
#29015=CARTESIAN_POINT('Ctrl Pts',(0.153995635016914,0.146040086863831,
8.50382510390846));
#29016=CARTESIAN_POINT('Ctrl Pts',(0.20621514597988,-0.0501771222878196,
8.49271131485164));
#29017=CARTESIAN_POINT('Ctrl Pts',(0.0696829962686225,-0.200465865858373,
8.48159752579486));
#29018=CARTESIAN_POINT('Ctrl Pts',(-0.130630488200291,-0.167266320497988,
8.47048373673803));
#29019=CARTESIAN_POINT('Ctrl Pts',(-0.211376557635571,0.0190341823579378,
8.45936994768125));
#29020=CARTESIAN_POINT('Ctrl Pts',(-0.0986471899183328,0.187912382699423,
8.44825615862442));
#29021=CARTESIAN_POINT('Ctrl Pts',(0.104375030754843,0.184792298274526,
8.43714236956764));
#29022=CARTESIAN_POINT('Ctrl Pts',(0.211861621603787,0.0125297022452017,
8.42602858051082));
#29023=CARTESIAN_POINT('Ctrl Pts',(0.125428857682743,-0.171201459585636,
8.41491479145403));
#29024=CARTESIAN_POINT('Ctrl Pts',(-0.0758103571728818,-0.198229990334955,
8.40380100239721));
#29025=CARTESIAN_POINT('Ctrl Pts',(-0.207659494862385,-0.0438163596056552,
8.39268721334042));
#29026=CARTESIAN_POINT('Ctrl Pts',(-0.149435540623878,0.150702880346313,
8.38157342428361));
#29027=CARTESIAN_POINT('Ctrl Pts',(0.0455684580258277,0.207282065655146,
8.3704596352268));
#29028=CARTESIAN_POINT('Ctrl Pts',(0.19886313058378,0.0741336251154622,
8.35934584617));
#29029=CARTESIAN_POINT('Ctrl Pts',(0.170136124295381,-0.126870163015214,
8.34823205711319));
#29030=CARTESIAN_POINT('Ctrl Pts',(-0.0143184059539161,-0.211748252238281,
8.33711826805639));
#29031=CARTESIAN_POINT('Ctrl Pts',(-0.185667136892942,-0.102810764745833,
8.32600447899959));
#29032=CARTESIAN_POINT('Ctrl Pts',(-0.187072631804583,0.10023058164497,
8.31489068994278));
#29033=CARTESIAN_POINT('Ctrl Pts',(-0.0172484252880032,0.211529739977579,
8.30377690088599));
#29034=CARTESIAN_POINT('Ctrl Pts',(0.168363460510403,0.129213328391465,
8.29266311182917));
#29035=CARTESIAN_POINT('Ctrl Pts',(0.199870361529475,-0.0713735080467207,
8.28154932277237));
#29036=CARTESIAN_POINT('Ctrl Pts',(0.0484336539578921,-0.206631363140847,
8.27043553371557));
#29037=CARTESIAN_POINT('Ctrl Pts',(-0.14733492635702,-0.152757188192241,
8.25932174465876));
#29038=CARTESIAN_POINT('Ctrl Pts',(-0.208246177685301,0.0409373734926227,
8.24820795560196));
#29039=CARTESIAN_POINT('Ctrl Pts',(-0.0785473409061163,0.197161492958519,
8.23709416654515));
#29040=CARTESIAN_POINT('Ctrl Pts',(0.123046767791955,0.172921461955964,
8.22598037748835));
#29041=CARTESIAN_POINT('Ctrl Pts',(0.21201477448475,-0.00959554423758641,
8.21486658843154));
#29042=CARTESIAN_POINT('Ctrl Pts',(0.106923253680599,-0.18332963996963,
8.20375279937475));
#29043=CARTESIAN_POINT('Ctrl Pts',(-0.0960363338095857,-0.189260037137931,
8.19263901031793));
#29044=CARTESIAN_POINT('Ctrl Pts',(-0.211092775837749,-0.0219585759590876,
8.18152522126114));
#29045=CARTESIAN_POINT('Ctrl Pts',(-0.132933606186724,0.165441818822301,
8.17041143220433));
#29046=CARTESIAN_POINT('Ctrl Pts',(0.0669012007766416,0.2014114405978,8.15929764314753));
#29047=CARTESIAN_POINT('Ctrl Pts',(0.205500579957926,0.053026886633043,
8.14818385409072));
#29048=CARTESIAN_POINT('Ctrl Pts',(0.156002947768637,-0.143893778032735,
8.13707006503392));
#29049=CARTESIAN_POINT('Ctrl Pts',(-0.0362859517070463,-0.209106835798716,
8.12595627597711));
#29050=CARTESIAN_POINT('Ctrl Pts',(-0.195361908074584,-0.0829220353253264,
8.11484248692031));
#29051=CARTESIAN_POINT('Ctrl Pts',(-0.175620894426736,0.119162244481181,
8.10372869786351));
#29052=CARTESIAN_POINT('Ctrl Pts',(0.00486791556632166,0.212175970522286,
8.09261490880669));
#29053=CARTESIAN_POINT('Ctrl Pts',(0.180901067235581,0.110982624505203,
8.0815011197499));
#29054=CARTESIAN_POINT('Ctrl Pts',(0.19135342050653,-0.0917943763501063,
8.07038733069309));
#29055=CARTESIAN_POINT('Ctrl Pts',(0.0266578178923598,-0.210550943513038,
8.0592735416363));
#29056=CARTESIAN_POINT('Ctrl Pts',(-0.162437987758694,-0.136587844268567,
8.04815975257947));
#29057=CARTESIAN_POINT('Ctrl Pts',(-0.202852461042557,0.0623956578468004,
8.03704596352269));
#29058=CARTESIAN_POINT('Ctrl Pts',(-0.0575937762299663,0.204267706719371,
8.02593217446586));
#29059=CARTESIAN_POINT('Ctrl Pts',(0.140381145122117,0.159171207079804,
8.01481838540908));
#29060=CARTESIAN_POINT('Ctrl Pts',(0.209863612316717,-0.0316165035270548,
8.00370459635226));
#29061=CARTESIAN_POINT('Ctrl Pts',(0.0872555351361295,-0.193465269894341,
7.99259080729547));
#29062=CARTESIAN_POINT('Ctrl Pts',(-0.11521852288682,-0.178233080693301,
7.98147701823866));
#29063=CARTESIAN_POINT('Ctrl Pts',(-0.212231760269946,0.000137868589443255,
7.97036322918185));
#29064=CARTESIAN_POINT('Ctrl Pts',(-0.114986860555745,0.178382625144081,
7.95924944012505));
#29065=CARTESIAN_POINT('Ctrl Pts',(0.0875068165648974,0.193351741996339,
7.94813565106825));
#29066=CARTESIAN_POINT('Ctrl Pts',(0.20990451228707,0.031343816465821,7.93702186201144));
#29067=CARTESIAN_POINT('Ctrl Pts',(0.140174227040771,-0.159353459390588,
7.92590807295464));
#29068=CARTESIAN_POINT('Ctrl Pts',(-0.057859117120295,-0.20419270736648,
7.91479428389783));
#29069=CARTESIAN_POINT('Ctrl Pts',(-0.202933356760109,-0.0621320532169235,
7.90368049484103));
#29070=CARTESIAN_POINT('Ctrl Pts',(-0.162260390470522,0.136798771150197,
7.89256670578423));
#29071=CARTESIAN_POINT('Ctrl Pts',(0.0269313452938532,0.210516134269093,
7.88145291672742));
#29072=CARTESIAN_POINT('Ctrl Pts',(0.191472527348541,0.0915456815880331,
7.87033912767062));
#29073=CARTESIAN_POINT('Ctrl Pts',(0.180756709756699,-0.111217550451763,
7.85922533861381));
#29074=CARTESIAN_POINT('Ctrl Pts',(0.00459227324043899,-0.212182139310508,
7.84811154955701));
#29075=CARTESIAN_POINT('Ctrl Pts',(-0.175775617131964,-0.118933926371996,
7.83699776050021));
#29076=CARTESIAN_POINT('Ctrl Pts',(-0.195253905127734,0.0831756928176114,
7.8258839714434));
#29077=CARTESIAN_POINT('Ctrl Pts',(-0.0360144494782014,0.209153985047792,
7.8147701823866));
#29078=CARTESIAN_POINT('Ctrl Pts',(0.156190174115918,0.143690612376374,
7.80365639332979));
#29079=CARTESIAN_POINT('Ctrl Pts',(0.205430704490901,-0.0532931174065624,
7.79254260427299));
#29080=CARTESIAN_POINT('Ctrl Pts',(0.0666410680213578,-0.2014996107808,
7.78142881521619));
#29081=CARTESIAN_POINT('Ctrl Pts',(-0.133151618919797,-0.165266151365589,
7.77031502615938));
#29082=CARTESIAN_POINT('Ctrl Pts',(-0.211057764439563,0.022227227740222,
7.75920123710257));
#29083=CARTESIAN_POINT('Ctrl Pts',(-0.0958028645069595,0.189395730904567,
7.74808744804577));
#29084=CARTESIAN_POINT('Ctrl Pts',(0.107186155178657,0.183168589451649,
7.73697365898897));
#29085=CARTESIAN_POINT('Ctrl Pts',(0.211977774262937,0.00936370041215743,
7.72585986993216));
#29086=CARTESIAN_POINT('Ctrl Pts',(0.122920892545772,-0.173168062155858,
7.71474608087536));
#29087=CARTESIAN_POINT('Ctrl Pts',(-0.079013003563882,-0.196882373561149,
7.70363229181855));
#29088=CARTESIAN_POINT('Ctrl Pts',(-0.164790318539738,-0.0930071057176291,
7.69622309911402));
#29089=CARTESIAN_POINT('Ctrl Pts',(-0.17623115053165,-0.034406055451555,
7.69251850276175));
#29090=CARTESIAN_POINT('Ctrl Pts',(-0.042986425688576,-0.160958774866487,
8.62244449171475));
#29091=CARTESIAN_POINT('Ctrl Pts',(-0.0965090477009803,-0.146664765635227,
8.61873989536248));
#29092=CARTESIAN_POINT('Ctrl Pts',(-0.187243042669588,-0.0606979027738561,
8.61133070265794));
#29093=CARTESIAN_POINT('Ctrl Pts',(-0.152529350659133,0.124729021753987,
8.60021691360114));
#29094=CARTESIAN_POINT('Ctrl Pts',(0.022064413364504,0.19563124996953,8.58910312454432));
#29095=CARTESIAN_POINT('Ctrl Pts',(0.176329000624295,0.0876438392864277,
8.57798933548754));
#29096=CARTESIAN_POINT('Ctrl Pts',(0.169264750726611,-0.100652039999728,
8.56687554643072));
#29097=CARTESIAN_POINT('Ctrl Pts',(0.00723673583350253,-0.196776112649654,
8.55576175737392));
#29098=CARTESIAN_POINT('Ctrl Pts',(-0.161398094283972,-0.112810885249515,
8.54464796831711));
#29099=CARTESIAN_POINT('Ctrl Pts',(-0.182312015731842,0.0744225714199578,
8.53353417926031));
#29100=CARTESIAN_POINT('Ctrl Pts',(-0.0363493466651971,0.19353058415634,
8.52242039020351));
#29101=CARTESIAN_POINT('Ctrl Pts',(0.142882105873586,0.13550069228114,8.51130660114671));
#29102=CARTESIAN_POINT('Ctrl Pts',(0.191333048611396,-0.0465559487992802,
8.50019281208989));
#29103=CARTESIAN_POINT('Ctrl Pts',(0.0646541263935723,-0.185998681498147,
8.4890790230331));
#29104=CARTESIAN_POINT('Ctrl Pts',(-0.121203170747678,-0.155195074924388,
8.47796523397628));
#29105=CARTESIAN_POINT('Ctrl Pts',(-0.196121972443975,0.0176605269271775,
8.46685144491949));
#29106=CARTESIAN_POINT('Ctrl Pts',(-0.0915280373531031,0.174351155841967,
8.45573765586269));
#29107=CARTESIAN_POINT('Ctrl Pts',(0.0968425124077976,0.171456241105691,
8.44462386680587));
#29108=CARTESIAN_POINT('Ctrl Pts',(0.196572030403439,0.0116254609591159,
8.43351007774908));
#29109=CARTESIAN_POINT('Ctrl Pts',(0.116376930560793,-0.158846223605886,
8.42239628869226));
#29110=CARTESIAN_POINT('Ctrl Pts',(-0.0703392890240059,-0.183924164235226,
8.41128249963547));
#29111=CARTESIAN_POINT('Ctrl Pts',(-0.192673161984908,-0.040654228488247,
8.40016871057866));
#29112=CARTESIAN_POINT('Ctrl Pts',(-0.138651103548177,0.139826982126676,
8.38905492152185));
#29113=CARTESIAN_POINT('Ctrl Pts',(0.0422798817864365,0.192322971020452,
8.37794113246506));
#29114=CARTESIAN_POINT('Ctrl Pts',(0.184511612133054,0.0687835630625294,
8.36682734340824));
#29115=CARTESIAN_POINT('Ctrl Pts',(0.157857771240231,-0.117714220030638,
8.35571355435146));
#29116=CARTESIAN_POINT('Ctrl Pts',(-0.0132850778220027,-0.196466842657805,
8.34459976529463));
#29117=CARTESIAN_POINT('Ctrl Pts',(-0.172267944528876,-0.0953911360652848,
8.33348597623784));
#29118=CARTESIAN_POINT('Ctrl Pts',(-0.173572007937867,0.092997159151912,
8.32237218718103));
#29119=CARTESIAN_POINT('Ctrl Pts',(-0.016003644050576,0.196264099950422,
8.31125839812423));
#29120=CARTESIAN_POINT('Ctrl Pts',(0.156213036734765,0.119888284271693,
8.30014460906742));
#29121=CARTESIAN_POINT('Ctrl Pts',(0.185446153417982,-0.066222637623337,
8.28903082001062));
#29122=CARTESIAN_POINT('Ctrl Pts',(0.0449383027765433,-0.191719228287548,
8.27791703095383));
#29123=CARTESIAN_POINT('Ctrl Pts',(-0.136702086031909,-0.141733035055427,
8.266803241897));
#29124=CARTESIAN_POINT('Ctrl Pts',(-0.19321750518794,0.0379830125244588,
8.25568945284021));
#29125=CARTESIAN_POINT('Ctrl Pts',(-0.0728787506100653,0.182932777984253,
8.2445756637834));
#29126=CARTESIAN_POINT('Ctrl Pts',(0.114166750902528,0.160442097156153,
8.23346187472661));
#29127=CARTESIAN_POINT('Ctrl Pts',(0.196714130574981,-0.0089030547360575,
8.22234808566979));
#29128=CARTESIAN_POINT('Ctrl Pts',(0.0992068356422025,-0.170099139660873,
8.21123429661299));
#29129=CARTESIAN_POINT('Ctrl Pts',(-0.0891056010359326,-0.175601552998632,
8.20012050755619));
#29130=CARTESIAN_POINT('Ctrl Pts',(-0.195858670559627,-0.0203738734196908,
8.18900671849937));
#29131=CARTESIAN_POINT('Ctrl Pts',(-0.123340077731702,0.153502243555736,
8.17789292944259));
#29132=CARTESIAN_POINT('Ctrl Pts',(0.062073087015669,0.186876016170753,
8.16677914038577));
#29133=CARTESIAN_POINT('Ctrl Pts',(0.190670051260911,0.0492000518665148,
8.15566535132897));
#29134=CARTESIAN_POINT('Ctrl Pts',(0.144744555241592,-0.133509277877683,
8.14455156227217));
#29135=CARTESIAN_POINT('Ctrl Pts',(-0.0336672737052616,-0.194016051482245,
8.13343777321535));
#29136=CARTESIAN_POINT('Ctrl Pts',(-0.181263065216832,-0.076937732873436,
8.12232398415856));
#29137=CARTESIAN_POINT('Ctrl Pts',(-0.16294671747247,0.11056256516767,8.11121019510174));
#29138=CARTESIAN_POINT('Ctrl Pts',(0.00451660871591894,0.196863693446027,
8.10009640604495));
#29139=CARTESIAN_POINT('Ctrl Pts',(0.167845831724775,0.102973250527127,
8.08898261698814));
#29140=CARTESIAN_POINT('Ctrl Pts',(0.177543861454799,-0.0851697763953834,
8.07786882793134));
#29141=CARTESIAN_POINT('Ctrl Pts',(0.0247339813108116,-0.195355941092154,
8.06675503887455));
#29142=CARTESIAN_POINT('Ctrl Pts',(-0.150715192429192,-0.126730597420393,
8.05564124981772));
#29143=CARTESIAN_POINT('Ctrl Pts',(-0.18821304131261,0.0578926992933231,
8.04452746076093));
#29144=CARTESIAN_POINT('Ctrl Pts',(-0.0534373590007651,0.189526151795315,
8.03341367170412));
#29145=CARTESIAN_POINT('Ctrl Pts',(0.130250144023825,0.147684168187657,
8.02229988264732));
#29146=CARTESIAN_POINT('Ctrl Pts',(0.194718213089331,-0.0293348094172218,
8.01118609359052));
#29147=CARTESIAN_POINT('Ctrl Pts',(0.0809584934534505,-0.179503303277842,
8.00007230453371));
#29148=CARTESIAN_POINT('Ctrl Pts',(-0.10690345336025,-0.165370387952869,
7.98895851547691));
#29149=CARTESIAN_POINT('Ctrl Pts',(-0.196915456969266,0.000127918914008822,
7.9778447264201));
#29150=CARTESIAN_POINT('Ctrl Pts',(-0.106688509594396,0.165509140106765,
7.9667309373633));
#29151=CARTESIAN_POINT('Ctrl Pts',(0.0811916404495023,0.179397968440655,
7.95561714830649));
#29152=CARTESIAN_POINT('Ctrl Pts',(0.194756161398019,0.0290818015865176,
7.94450335924969));
#29153=CARTESIAN_POINT('Ctrl Pts',(0.13005815876916,-0.14785326774663,7.93338957019289));
#29154=CARTESIAN_POINT('Ctrl Pts',(-0.0536835508176979,-0.189456564982163,
7.92227578113608));
#29155=CARTESIAN_POINT('Ctrl Pts',(-0.188288098962645,-0.0576481184347118,
7.91116199207928));
#29156=CARTESIAN_POINT('Ctrl Pts',(-0.150550411950001,0.126926302168967,
7.90004820302248));
#29157=CARTESIAN_POINT('Ctrl Pts',(0.0249877688362514,0.195323643955433,
7.88893441396566));
#29158=CARTESIAN_POINT('Ctrl Pts',(0.177654372615772,0.0849390293919319,
7.87782062490887));
#29159=CARTESIAN_POINT('Ctrl Pts',(0.167711892210327,-0.103191222380454,
7.86670683585206));
#29160=CARTESIAN_POINT('Ctrl Pts',(0.00426085889557056,-0.196869417046256,
7.85559304679526));
#29161=CARTESIAN_POINT('Ctrl Pts',(-0.163090274177483,-0.110350724278505,
7.84447925773845));
#29162=CARTESIAN_POINT('Ctrl Pts',(-0.181162856607122,0.0771730844576825,
7.83336546868165));
#29163=CARTESIAN_POINT('Ctrl Pts',(-0.0334153652001765,0.194059798072839,
7.82225167962485));
#29164=CARTESIAN_POINT('Ctrl Pts',(0.144918269871696,0.133320774243675,
7.81113789056804));
#29165=CARTESIAN_POINT('Ctrl Pts',(0.190605218553956,-0.0494470693457091,
7.80002410151123));
#29166=CARTESIAN_POINT('Ctrl Pts',(0.0618317274740329,-0.186957823303929,
7.78891031245443));
#29167=CARTESIAN_POINT('Ctrl Pts',(-0.123542356961275,-0.153339253636277,
7.77779652339763));
#29168=CARTESIAN_POINT('Ctrl Pts',(-0.195826185857694,0.0206231371876604,
7.76668273434082));
#29169=CARTESIAN_POINT('Ctrl Pts',(-0.0888889807037237,0.175727454042052,
7.75556894528402));
#29170=CARTESIAN_POINT('Ctrl Pts',(0.0994507641124849,0.169949711807554,
7.74445515622721));
#29171=CARTESIAN_POINT('Ctrl Pts',(0.196679800578486,0.00868794257390136,
7.73334136717042));
#29172=CARTESIAN_POINT('Ctrl Pts',(0.114049959798351,-0.16067090075741,
7.72222757811361));
#29173=CARTESIAN_POINT('Ctrl Pts',(-0.0733108074093436,-0.182673802025085,
7.7111137890568));
#29174=CARTESIAN_POINT('Ctrl Pts',(-0.152897760627765,-0.0862949857291892,
7.70370459635227));
#29175=CARTESIAN_POINT('Ctrl Pts',(-0.163512932725147,-0.0319230454628249,
7.7));
#29176=CARTESIAN_POINT('Ctrl Pts',(-0.166383640089184,9.41837290711752E-5,
8.53785196366098));
#29177=CARTESIAN_POINT('Ctrl Pts',(-0.166495359952371,0.0216826172703768,
8.53641270219409));
#29178=CARTESIAN_POINT('Ctrl Pts',(-0.162596302111187,0.0432323652637361,
8.5349734407272));
#29179=CARTESIAN_POINT('Ctrl Pts',(-0.15449925064609,0.0630683307644428,
8.53353417926031));
#29180=CARTESIAN_POINT('Ctrl Pts',(-0.133657792709627,0.114125242332085,
8.52982958290805));
#29181=CARTESIAN_POINT('Ctrl Pts',(-0.0850035696874118,0.153827913244213,
8.52612498655578));
#29182=CARTESIAN_POINT('Ctrl Pts',(-0.0308045494198404,0.164007600054409,
8.52242039020351));
#29183=CARTESIAN_POINT('Ctrl Pts',(0.0233944708477309,0.174187286864606,
8.51871579385124));
#29184=CARTESIAN_POINT('Ctrl Pts',(0.0831382883606584,0.154843989572873,
8.51501119749897));
#29185=CARTESIAN_POINT('Ctrl Pts',(0.121085354240091,0.114829567413603,
8.51130660114671));
#29186=CARTESIAN_POINT('Ctrl Pts',(0.159032420119523,0.0748151452543328,
8.50760200479444));
#29187=CARTESIAN_POINT('Ctrl Pts',(0.17518273436546,0.0141295982275263,
8.50389740844216));
#29188=CARTESIAN_POINT('Ctrl Pts',(0.162144737785457,-0.0394536307356881,
8.5001928120899));
#29189=CARTESIAN_POINT('Ctrl Pts',(0.149106741205455,-0.0930368596989026,
8.49648821573763));
#29190=CARTESIAN_POINT('Ctrl Pts',(0.106880433799514,-0.139517770598525,
8.49278361938537));
#29191=CARTESIAN_POINT('Ctrl Pts',(0.0547910639063346,-0.157624291619376,
8.4890790230331));
#29192=CARTESIAN_POINT('Ctrl Pts',(0.00270169401315546,-0.175730812640227,
8.48537442668083));
#29193=CARTESIAN_POINT('Ctrl Pts',(-0.0592507383672613,-0.165462943782308,
8.48166983032856));
#29194=CARTESIAN_POINT('Ctrl Pts',(-0.102713421506852,-0.131519742378087,
8.47796523397629));
#29195=CARTESIAN_POINT('Ctrl Pts',(-0.142263377059629,-0.100632277318825,
8.47459414387118));
#29196=CARTESIAN_POINT('Ctrl Pts',(-0.166502812179775,-0.0501403461319692,
8.47122305376608));
#29197=CARTESIAN_POINT('Ctrl Pts',(-0.16681984310415,8.64016909114964E-5,
8.46785196366098));
#29198=CARTESIAN_POINT('Ctrl Pts',(-0.0530170217188485,-0.198517432567176,
8.6));
#29199=CARTESIAN_POINT('Ctrl Pts',(-0.06542081092342,-0.193924769288753,
8.6));
#29200=CARTESIAN_POINT('Ctrl Pts',(-0.0772704541431171,-0.188065565737325,
8.6));
#29201=CARTESIAN_POINT('Ctrl Pts',(-0.0884481740526511,-0.181102974015431,
8.6));
#29202=CARTESIAN_POINT('Ctrl Pts',(-0.0941164108607929,-0.1775722343836,
8.6));
#29203=CARTESIAN_POINT('Ctrl Pts',(-0.0996114240419522,-0.173757009103972,
8.6));
#29204=CARTESIAN_POINT('Ctrl Pts',(-0.104914415136506,-0.169674993381027,
8.6));
#29205=CARTESIAN_POINT('Ctrl Pts',(-0.109523380425031,-0.166127209038415,
8.6));
#29206=CARTESIAN_POINT('Ctrl Pts',(-0.113987272284976,-0.162377843722833,
8.6));
#29207=CARTESIAN_POINT('Ctrl Pts',(-0.118291910700038,-0.158437614516047,
8.6));
#29208=CARTESIAN_POINT('Ctrl Pts',(-0.121383799927864,-0.155607469201867,
8.6));
#29209=CARTESIAN_POINT('Ctrl Pts',(-0.124387199055957,-0.15268442084067,
8.6));
#29210=CARTESIAN_POINT('Ctrl Pts',(-0.127293146906171,-0.14967825940901,
8.6));
#29211=CARTESIAN_POINT('Ctrl Pts',(-0.136236980136076,-0.140425992027493,
8.6));
#29212=CARTESIAN_POINT('Ctrl Pts',(-0.144276520214277,-0.130374017836739,
8.6));
#29213=CARTESIAN_POINT('Ctrl Pts',(-0.151272696882763,-0.119653258631744,
8.6));
#29214=CARTESIAN_POINT('Ctrl Pts',(-0.155802688817768,-0.112711616784059,
8.6));
#29215=CARTESIAN_POINT('Ctrl Pts',(-0.159894413372832,-0.10548900882637,
8.6));
#29216=CARTESIAN_POINT('Ctrl Pts',(-0.163498383914012,-0.0980183248117674,
8.6));
#29217=CARTESIAN_POINT('Ctrl Pts',(-0.165162652591317,-0.0945684560457829,
8.6));
#29218=CARTESIAN_POINT('Ctrl Pts',(-0.166718761668699,-0.0910738139207644,
8.6));
#29219=CARTESIAN_POINT('Ctrl Pts',(-0.168161639193221,-0.0875412396582513,
8.6));
#29220=CARTESIAN_POINT('Ctrl Pts',(-0.172163015187704,-0.0777447339864133,
8.6));
#29221=CARTESIAN_POINT('Ctrl Pts',(-0.175299623694641,-0.0676487151368408,
8.6));
#29222=CARTESIAN_POINT('Ctrl Pts',(-0.177477376050015,-0.057326480317048,
8.6));
#29223=CARTESIAN_POINT('Ctrl Pts',(-0.179331110212822,-0.0485400454064169,
8.6));
#29224=CARTESIAN_POINT('Ctrl Pts',(-0.18048935110848,-0.0395892198362765,
8.6));
#29225=CARTESIAN_POINT('Ctrl Pts',(-0.180964733448231,-0.0305523301186972,
8.6));
#29226=CARTESIAN_POINT('Ctrl Pts',(-0.181133859445773,-0.0273372906433986,
8.6));
#29227=CARTESIAN_POINT('Ctrl Pts',(-0.181216193772417,-0.0241127956726884,
8.6));
#29228=CARTESIAN_POINT('Ctrl Pts',(-0.181212666773714,-0.0208920829129295,
8.6));
#29229=CARTESIAN_POINT('Ctrl Pts',(-0.18119984414273,-0.00918297420461843,
8.6));
#29230=CARTESIAN_POINT('Ctrl Pts',(-0.180057695209983,0.00251249492629139,
8.6));
#29231=CARTESIAN_POINT('Ctrl Pts',(-0.177831621291215,0.0140219353702633,
8.6));
#29232=CARTESIAN_POINT('Ctrl Pts',(-0.176688035248831,0.0199346031107226,
8.6));
#29233=CARTESIAN_POINT('Ctrl Pts',(-0.17525769513229,0.0257979924523235,
8.6));
#29234=CARTESIAN_POINT('Ctrl Pts',(-0.173542822423344,0.0315864625403328,
8.6));
#29235=CARTESIAN_POINT('Ctrl Pts',(-0.171856156212592,0.0372797229546229,
8.6));
#29236=CARTESIAN_POINT('Ctrl Pts',(-0.169891488737815,0.0429059368612729,
8.6));
#29237=CARTESIAN_POINT('Ctrl Pts',(-0.167662780533083,0.048407845623496,
8.6));
#29238=CARTESIAN_POINT('Ctrl Pts',(-0.164206394717703,0.0569404652651757,
8.6));
#29239=CARTESIAN_POINT('Ctrl Pts',(-0.160113292534287,0.0651877483840102,
8.6));
#29240=CARTESIAN_POINT('Ctrl Pts',(-0.155392822172953,0.0730538252569167,
8.6));
#29241=CARTESIAN_POINT('Ctrl Pts',(-0.152978226140765,0.0770774492927307,
8.6));
#29242=CARTESIAN_POINT('Ctrl Pts',(-0.150398552838242,0.0810014273591959,
8.6));
#29243=CARTESIAN_POINT('Ctrl Pts',(-0.147663850341513,0.0847992235167022,
8.6));
#29244=CARTESIAN_POINT('Ctrl Pts',(-0.142229060792935,0.0923467439102818,
8.6));
#29245=CARTESIAN_POINT('Ctrl Pts',(-0.136175359211409,0.0994106650199937,
8.6));
#29246=CARTESIAN_POINT('Ctrl Pts',(-0.129507404772142,0.105879808304267,
8.6));
#29247=CARTESIAN_POINT('Ctrl Pts',(-0.128728930874604,0.106635071291155,
8.6));
#29248=CARTESIAN_POINT('Ctrl Pts',(-0.127942070273424,0.107382201802382,
8.6));
#29249=CARTESIAN_POINT('Ctrl Pts',(-0.127146980098767,0.108121134152663,
8.6));
#29250=CARTESIAN_POINT('Origin',(0.,0.,8.1));
#29251=CARTESIAN_POINT('Origin',(0.,0.,7.6));
#29252=CARTESIAN_POINT('Origin',(0.,0.,7.1));
#29253=CARTESIAN_POINT('',(-0.6,-7.34788079488412E-17,7.36457513110646));
#29254=CARTESIAN_POINT('Origin',(0.,0.,7.36457513110646));
#29255=CARTESIAN_POINT('',(-0.6,-7.34788079488412E-17,6.83542486889354));
#29256=CARTESIAN_POINT('Origin',(-0.899999999999998,-1.10218211923262E-16,
7.1));
#29257=CARTESIAN_POINT('Origin',(0.,0.,6.83542486889354));
#29258=CARTESIAN_POINT('Origin',(0.,0.,2.4));
#29259=CARTESIAN_POINT('',(-0.6,-7.34788079488412E-17,6.56457513110646));
#29260=CARTESIAN_POINT('',(-0.6,-7.34788079488412E-17,2.4));
#29261=CARTESIAN_POINT('Origin',(0.,0.,6.56457513110646));
#29262=CARTESIAN_POINT('Origin',(0.,0.,6.3));
#29263=CARTESIAN_POINT('',(-0.6,-7.34788079488412E-17,6.03542486889354));
#29264=CARTESIAN_POINT('Origin',(-0.900000000000001,-1.10218211923262E-16,
6.3));
#29265=CARTESIAN_POINT('Origin',(0.,0.,6.03542486889354));
#29266=CARTESIAN_POINT('Origin',(0.,0.,2.4));
#29267=CARTESIAN_POINT('',(-0.6,-7.34788079488412E-17,2.4));
#29268=CARTESIAN_POINT('',(-0.6,-7.34788079488412E-17,2.4));
#29269=CARTESIAN_POINT('Origin',(0.,0.,2.4));
#29270=CARTESIAN_POINT('Origin',(0.,0.,7.8));
#29271=CARTESIAN_POINT('',(-1.,-1.22464679914735E-16,7.8));
#29272=CARTESIAN_POINT('Origin',(0.,0.,7.8));
#29273=CARTESIAN_POINT('',(-0.6,-7.34788079488412E-17,7.8));
#29274=CARTESIAN_POINT('Origin',(0.,0.,7.8));
#29275=CARTESIAN_POINT('Origin',(0.,0.,7.6));
#29276=CARTESIAN_POINT('',(-1.,-1.22464679914735E-16,7.6));
#29277=CARTESIAN_POINT('Origin',(0.,0.,7.6));
#29278=CARTESIAN_POINT('',(-0.6,7.34788079488412E-17,7.6));
#29279=CARTESIAN_POINT('Origin',(0.,0.,7.6));
#29280=CARTESIAN_POINT('Origin',(0.,0.,7.6));
#29281=CARTESIAN_POINT('',(-1.,-1.22464679914735E-16,7.6));
#29282=CARTESIAN_POINT('Origin',(0.,0.,2.4));
#29283=CARTESIAN_POINT('',(-0.6,-7.34788079488412E-17,2.4));
#29284=CARTESIAN_POINT('Origin',(-1.8,0.6,2.));
#29285=CARTESIAN_POINT('',(0.8,0.6,2.4));
#29286=CARTESIAN_POINT('',(0.8,0.6,2.));
#29287=CARTESIAN_POINT('',(1.8,0.6,2.4));
#29288=CARTESIAN_POINT('',(1.8,0.6,2.));
#29289=CARTESIAN_POINT('',(-1.8,0.6,2.4));
#29290=CARTESIAN_POINT('Origin',(1.8,1.4,2.));
#29291=CARTESIAN_POINT('',(-1.8,1.4,2.4));
#29292=CARTESIAN_POINT('',(-1.8,1.4,2.));
#29293=CARTESIAN_POINT('',(1.8,1.4,2.4));
#29294=CARTESIAN_POINT('',(1.8,1.4,2.4));
#29295=CARTESIAN_POINT('',(1.8,1.4,2.));
#29296=CARTESIAN_POINT('Origin',(1.8,0.6,2.));
#29297=CARTESIAN_POINT('',(1.8,0.6,2.4));
#29298=CARTESIAN_POINT('Origin',(-1.8,0.6,2.));
#29299=CARTESIAN_POINT('',(-0.8,0.6,2.4));
#29300=CARTESIAN_POINT('',(-0.8,0.6,2.));
#29301=CARTESIAN_POINT('',(-1.8,0.6,2.4));
#29302=CARTESIAN_POINT('',(-1.8,0.6,2.4));
#29303=CARTESIAN_POINT('',(-1.8,0.6,2.));
#29304=CARTESIAN_POINT('Origin',(-1.8,1.4,2.));
#29305=CARTESIAN_POINT('',(-1.8,1.4,2.4));
#29306=CARTESIAN_POINT('Origin',(0.,0.,2.));
#29307=CARTESIAN_POINT('Origin',(0.,0.,2.4));
#29308=CARTESIAN_POINT('Origin',(0.,0.,2.4));
#29309=CARTESIAN_POINT('',(-0.6,-7.34788079488412E-17,8.6));
#29310=CARTESIAN_POINT('Origin',(0.,0.,8.6));
#29311=CARTESIAN_POINT('',(-0.6,-7.34788079488412E-17,2.4));
#29312=CARTESIAN_POINT('Origin',(0.,0.,8.6));
#29313=CARTESIAN_POINT('Origin',(0.,0.,2.4));
#43947=UNCERTAINTY_MEASURE_WITH_UNIT(LENGTH_MEASURE(0.001),#43981,
'DISTANCE_ACCURACY_VALUE',
'Maximum model space distance between geometric entities at asserted c
onnectivities');
#43961=UNCERTAINTY_MEASURE_WITH_UNIT(LENGTH_MEASURE(0.001),#43981,
'DISTANCE_ACCURACY_VALUE',
'Maximum model space distance between geometric entities at asserted c
onnectivities');
#43966=(
GEOMETRIC_REPRESENTATION_CONTEXT(3)
GLOBAL_UNCERTAINTY_ASSIGNED_CONTEXT((#43947))
GLOBAL_UNIT_ASSIGNED_CONTEXT((#43981,#43983,#43984))
REPRESENTATION_CONTEXT('','3D')
);
#43980=(
GEOMETRIC_REPRESENTATION_CONTEXT(3)
GLOBAL_UNCERTAINTY_ASSIGNED_CONTEXT((#43961))
GLOBAL_UNIT_ASSIGNED_CONTEXT((#43981,#43983,#43984))
REPRESENTATION_CONTEXT('','3D')
);
#43981=(
LENGTH_UNIT()
NAMED_UNIT(*)
SI_UNIT(.CENTI.,.METRE.)
);
#43983=(
NAMED_UNIT(*)
PLANE_ANGLE_UNIT()
SI_UNIT($,.RADIAN.)
);
#43984=(
NAMED_UNIT(*)
SI_UNIT($,.STERADIAN.)
SOLID_ANGLE_UNIT()
);
#43989=SHAPE_DEFINITION_REPRESENTATION(#44007,#44059);
#44007=PRODUCT_DEFINITION_SHAPE('',$,#44078);
#44059=SHAPE_REPRESENTATION('',(#11740),#43966);
#44073=PRODUCT_DEFINITION_CONTEXT('part definition',#44129,'design');
#44078=PRODUCT_DEFINITION('Button actuator','Button actuator',#44096,#44073);
#44096=PRODUCT_DEFINITION_FORMATION('',$,#44135);
#44129=APPLICATION_CONTEXT(
'Core Data for Automotive Mechanical Design Process');
#44130=PRODUCT_CONTEXT('part definition',#44129,'mechanical');
#44135=PRODUCT('Button actuator','Button actuator',$,(#44130));
#44153=PRESENTATION_STYLE_ASSIGNMENT((#44165));
#44165=SURFACE_STYLE_USAGE(.BOTH.,#44177);
#44177=SURFACE_SIDE_STYLE('',(#44189));
#44189=SURFACE_STYLE_FILL_AREA(#44201);
#44201=FILL_AREA_STYLE('Light blue',(#44213));
#44213=FILL_AREA_STYLE_COLOUR('Light blue',#44225);
#44225=COLOUR_RGB('Light blue',0.662745098039216,0.831372549019608,0.949019607843137);
ENDSEC;
END-ISO-10303-21;
